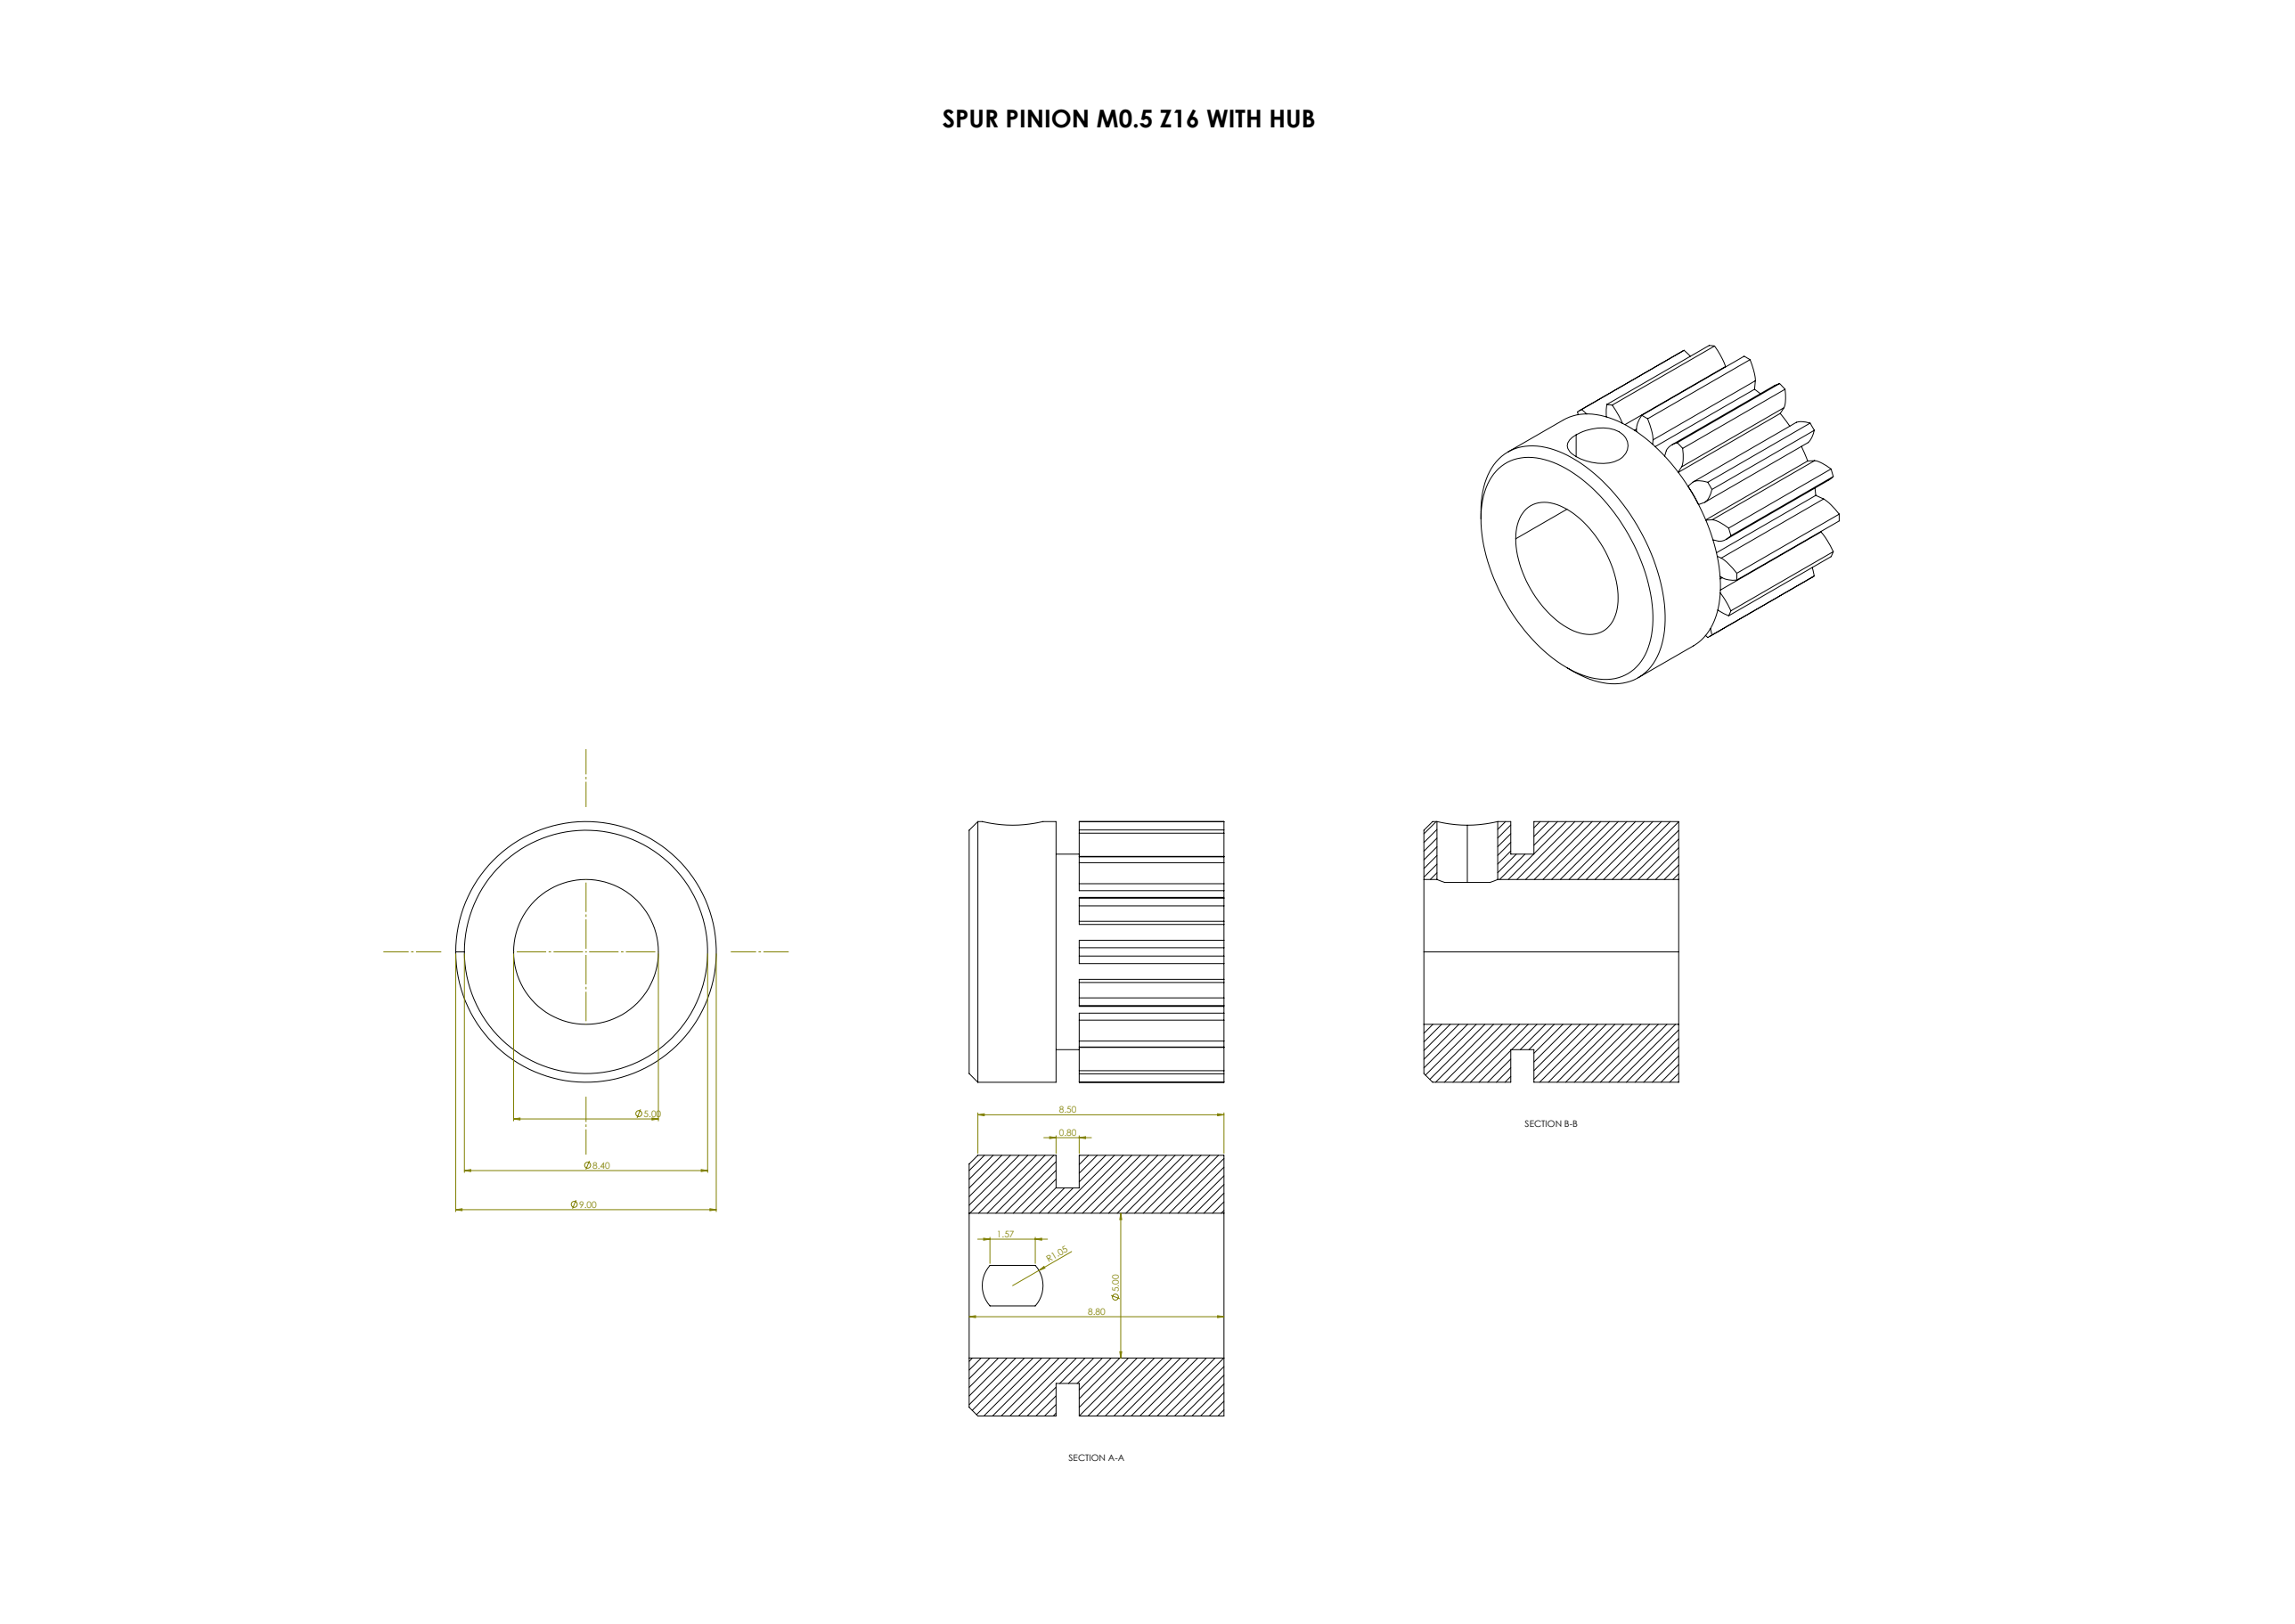
ISO-10303-21;
HEADER;
/* Generated by software containing ST-Developer
 * from STEP Tools, Inc. (www.steptools.com) 
 */

FILE_DESCRIPTION(
/* description */ (''),
/* implementation_level */ '2;1');

FILE_NAME(
/* name */ 'Spur Pinion m0.5 z16 with Hub.step',
/* time_stamp */ '2026-10-05T09:57:53+05:00',
/* author */ (''),
/* organization */ (''),
/* preprocessor_version */ 'ST-DEVELOPER v20.2',
/* originating_system */ 'Autodesk Translation Framework v15.15.0.0',
/* authorisation */ '');

FILE_SCHEMA (('AUTOMOTIVE_DESIGN { 1 0 10303 214 3 1 1 }'));
ENDSEC;

DATA;
#10=MECHANICAL_DESIGN_GEOMETRIC_PRESENTATION_REPRESENTATION('',(#555),#113984);
#110=(
BOUNDED_SURFACE()
B_SPLINE_SURFACE(5,1,((#92751,#92752),(#92753,#92754),(#92755,#92756),(#92757,
#92758),(#92759,#92760),(#92761,#92762),(#92763,#92764),(#92765,#92766),
(#92767,#92768),(#92769,#92770),(#92771,#92772),(#92773,#92774),(#92775,
#92776),(#92777,#92778),(#92779,#92780),(#92781,#92782),(#92783,#92784),
(#92785,#92786),(#92787,#92788),(#92789,#92790),(#92791,#92792),(#92793,
#92794),(#92795,#92796),(#92797,#92798),(#92799,#92800),(#92801,#92802),
(#92803,#92804),(#92805,#92806),(#92807,#92808),(#92809,#92810),(#92811,
#92812),(#92813,#92814),(#92815,#92816),(#92817,#92818),(#92819,#92820)),
 .UNSPECIFIED.,.F.,.F.,.F.)
B_SPLINE_SURFACE_WITH_KNOTS((6,1,1,1,1,1,1,1,1,1,1,1,1,1,1,1,1,1,1,1,1,
1,1,1,1,1,1,1,1,1,6),(2,2),(-1.,-0.966666666666667,-0.933333333333333,-0.9,
-0.866666666666667,-0.833333333333333,-0.8,-0.766666666666667,-0.733333333333333,
-0.7,-0.666666666666667,-0.633333333333333,-0.6,-0.566666666666667,-0.533333333333333,
-0.5,-0.466666666666667,-0.433333333333333,-0.4,-0.366666666666667,-0.333333333333333,
-0.3,-0.266666666666667,-0.233333333333333,-0.2,-0.166666666666667,-0.133333333333333,
-0.1,-0.0666666666666667,-0.0333333333333333,0.),(0.,0.5),.UNSPECIFIED.)
GEOMETRIC_REPRESENTATION_ITEM()
RATIONAL_B_SPLINE_SURFACE(((1.,1.),(1.,1.),(1.,1.),(1.,1.),(1.,1.),(1.,
1.),(1.,1.),(1.,1.),(1.,1.),(1.,1.),(1.,1.),(1.,1.),(1.,1.),(1.,1.),(1.,
1.),(1.,1.),(1.,1.),(1.,1.),(1.,1.),(1.,1.),(1.,1.),(1.,1.),(1.,1.),(1.,
1.),(1.,1.),(1.,1.),(1.,1.),(1.,1.),(1.,1.),(1.,1.),(1.,1.),(1.,1.),(1.,
1.),(1.,1.),(1.,1.)))
REPRESENTATION_ITEM('')
SURFACE()
);
#111=(
BOUNDED_SURFACE()
B_SPLINE_SURFACE(5,1,((#92900,#92901),(#92902,#92903),(#92904,#92905),(#92906,
#92907),(#92908,#92909),(#92910,#92911),(#92912,#92913),(#92914,#92915),
(#92916,#92917),(#92918,#92919),(#92920,#92921),(#92922,#92923),(#92924,
#92925),(#92926,#92927),(#92928,#92929),(#92930,#92931),(#92932,#92933),
(#92934,#92935),(#92936,#92937),(#92938,#92939),(#92940,#92941),(#92942,
#92943),(#92944,#92945),(#92946,#92947),(#92948,#92949),(#92950,#92951),
(#92952,#92953),(#92954,#92955),(#92956,#92957),(#92958,#92959),(#92960,
#92961),(#92962,#92963),(#92964,#92965),(#92966,#92967),(#92968,#92969)),
 .UNSPECIFIED.,.F.,.F.,.F.)
B_SPLINE_SURFACE_WITH_KNOTS((6,1,1,1,1,1,1,1,1,1,1,1,1,1,1,1,1,1,1,1,1,
1,1,1,1,1,1,1,1,1,6),(2,2),(0.,0.0333333333333333,0.0666666666666667,0.1,
0.133333333333333,0.166666666666667,0.2,0.233333333333333,0.266666666666667,
0.3,0.333333333333333,0.366666666666667,0.4,0.433333333333333,0.466666666666667,
0.5,0.533333333333333,0.566666666666667,0.6,0.633333333333333,0.666666666666667,
0.7,0.733333333333333,0.766666666666667,0.8,0.833333333333333,0.866666666666667,
0.9,0.933333333333333,0.966666666666667,1.),(0.,0.5),.UNSPECIFIED.)
GEOMETRIC_REPRESENTATION_ITEM()
RATIONAL_B_SPLINE_SURFACE(((1.,1.),(1.,1.),(1.,1.),(1.,1.),(1.,1.),(1.,
1.),(1.,1.),(1.,1.),(1.,1.),(1.,1.),(1.,1.),(1.,1.),(1.,1.),(1.,1.),(1.,
1.),(1.,1.),(1.,1.),(1.,1.),(1.,1.),(1.,1.),(1.,1.),(1.,1.),(1.,1.),(1.,
1.),(1.,1.),(1.,1.),(1.,1.),(1.,1.),(1.,1.),(1.,1.),(1.,1.),(1.,1.),(1.,
1.),(1.,1.),(1.,1.)))
REPRESENTATION_ITEM('')
SURFACE()
);
#112=(
BOUNDED_SURFACE()
B_SPLINE_SURFACE(5,1,((#93181,#93182),(#93183,#93184),(#93185,#93186),(#93187,
#93188),(#93189,#93190),(#93191,#93192),(#93193,#93194),(#93195,#93196),
(#93197,#93198),(#93199,#93200),(#93201,#93202),(#93203,#93204),(#93205,
#93206),(#93207,#93208),(#93209,#93210),(#93211,#93212),(#93213,#93214),
(#93215,#93216),(#93217,#93218),(#93219,#93220),(#93221,#93222),(#93223,
#93224),(#93225,#93226),(#93227,#93228),(#93229,#93230),(#93231,#93232),
(#93233,#93234),(#93235,#93236),(#93237,#93238),(#93239,#93240),(#93241,
#93242),(#93243,#93244),(#93245,#93246),(#93247,#93248),(#93249,#93250)),
 .UNSPECIFIED.,.F.,.F.,.F.)
B_SPLINE_SURFACE_WITH_KNOTS((6,1,1,1,1,1,1,1,1,1,1,1,1,1,1,1,1,1,1,1,1,
1,1,1,1,1,1,1,1,1,6),(2,2),(-1.,-0.966666666666667,-0.933333333333333,-0.9,
-0.866666666666667,-0.833333333333333,-0.8,-0.766666666666667,-0.733333333333333,
-0.7,-0.666666666666667,-0.633333333333333,-0.6,-0.566666666666667,-0.533333333333333,
-0.5,-0.466666666666667,-0.433333333333333,-0.4,-0.366666666666667,-0.333333333333333,
-0.3,-0.266666666666667,-0.233333333333333,-0.2,-0.166666666666667,-0.133333333333333,
-0.1,-0.0666666666666667,-0.0333333333333333,0.),(0.,0.5),.UNSPECIFIED.)
GEOMETRIC_REPRESENTATION_ITEM()
RATIONAL_B_SPLINE_SURFACE(((1.,1.),(1.,1.),(1.,1.),(1.,1.),(1.,1.),(1.,
1.),(1.,1.),(1.,1.),(1.,1.),(1.,1.),(1.,1.),(1.,1.),(1.,1.),(1.,1.),(1.,
1.),(1.,1.),(1.,1.),(1.,1.),(1.,1.),(1.,1.),(1.,1.),(1.,1.),(1.,1.),(1.,
1.),(1.,1.),(1.,1.),(1.,1.),(1.,1.),(1.,1.),(1.,1.),(1.,1.),(1.,1.),(1.,
1.),(1.,1.),(1.,1.)))
REPRESENTATION_ITEM('')
SURFACE()
);
#113=(
BOUNDED_SURFACE()
B_SPLINE_SURFACE(5,1,((#93330,#93331),(#93332,#93333),(#93334,#93335),(#93336,
#93337),(#93338,#93339),(#93340,#93341),(#93342,#93343),(#93344,#93345),
(#93346,#93347),(#93348,#93349),(#93350,#93351),(#93352,#93353),(#93354,
#93355),(#93356,#93357),(#93358,#93359),(#93360,#93361),(#93362,#93363),
(#93364,#93365),(#93366,#93367),(#93368,#93369),(#93370,#93371),(#93372,
#93373),(#93374,#93375),(#93376,#93377),(#93378,#93379),(#93380,#93381),
(#93382,#93383),(#93384,#93385),(#93386,#93387),(#93388,#93389),(#93390,
#93391),(#93392,#93393),(#93394,#93395),(#93396,#93397),(#93398,#93399)),
 .UNSPECIFIED.,.F.,.F.,.F.)
B_SPLINE_SURFACE_WITH_KNOTS((6,1,1,1,1,1,1,1,1,1,1,1,1,1,1,1,1,1,1,1,1,
1,1,1,1,1,1,1,1,1,6),(2,2),(0.,0.0333333333333333,0.0666666666666667,0.1,
0.133333333333333,0.166666666666667,0.2,0.233333333333333,0.266666666666667,
0.3,0.333333333333333,0.366666666666667,0.4,0.433333333333333,0.466666666666667,
0.5,0.533333333333333,0.566666666666667,0.6,0.633333333333333,0.666666666666667,
0.7,0.733333333333333,0.766666666666667,0.8,0.833333333333333,0.866666666666667,
0.9,0.933333333333333,0.966666666666667,1.),(0.,0.5),.UNSPECIFIED.)
GEOMETRIC_REPRESENTATION_ITEM()
RATIONAL_B_SPLINE_SURFACE(((1.,1.),(1.,1.),(1.,1.),(1.,1.),(1.,1.),(1.,
1.),(1.,1.),(1.,1.),(1.,1.),(1.,1.),(1.,1.),(1.,1.),(1.,1.),(1.,1.),(1.,
1.),(1.,1.),(1.,1.),(1.,1.),(1.,1.),(1.,1.),(1.,1.),(1.,1.),(1.,1.),(1.,
1.),(1.,1.),(1.,1.),(1.,1.),(1.,1.),(1.,1.),(1.,1.),(1.,1.),(1.,1.),(1.,
1.),(1.,1.),(1.,1.)))
REPRESENTATION_ITEM('')
SURFACE()
);
#114=(
BOUNDED_SURFACE()
B_SPLINE_SURFACE(5,1,((#93483,#93484),(#93485,#93486),(#93487,#93488),(#93489,
#93490),(#93491,#93492),(#93493,#93494),(#93495,#93496),(#93497,#93498),
(#93499,#93500),(#93501,#93502),(#93503,#93504),(#93505,#93506),(#93507,
#93508),(#93509,#93510),(#93511,#93512),(#93513,#93514),(#93515,#93516),
(#93517,#93518),(#93519,#93520),(#93521,#93522),(#93523,#93524),(#93525,
#93526),(#93527,#93528),(#93529,#93530),(#93531,#93532),(#93533,#93534),
(#93535,#93536),(#93537,#93538),(#93539,#93540),(#93541,#93542),(#93543,
#93544),(#93545,#93546),(#93547,#93548),(#93549,#93550),(#93551,#93552)),
 .UNSPECIFIED.,.F.,.F.,.F.)
B_SPLINE_SURFACE_WITH_KNOTS((6,1,1,1,1,1,1,1,1,1,1,1,1,1,1,1,1,1,1,1,1,
1,1,1,1,1,1,1,1,1,6),(2,2),(-1.,-0.966666666666667,-0.933333333333333,-0.9,
-0.866666666666667,-0.833333333333333,-0.8,-0.766666666666667,-0.733333333333333,
-0.7,-0.666666666666667,-0.633333333333333,-0.6,-0.566666666666667,-0.533333333333333,
-0.5,-0.466666666666667,-0.433333333333333,-0.4,-0.366666666666667,-0.333333333333333,
-0.3,-0.266666666666667,-0.233333333333333,-0.2,-0.166666666666667,-0.133333333333333,
-0.1,-0.0666666666666667,-0.0333333333333333,0.),(0.,0.5),.UNSPECIFIED.)
GEOMETRIC_REPRESENTATION_ITEM()
RATIONAL_B_SPLINE_SURFACE(((1.,1.),(1.,1.),(1.,1.),(1.,1.),(1.,1.),(1.,
1.),(1.,1.),(1.,1.),(1.,1.),(1.,1.),(1.,1.),(1.,1.),(1.,1.),(1.,1.),(1.,
1.),(1.,1.),(1.,1.),(1.,1.),(1.,1.),(1.,1.),(1.,1.),(1.,1.),(1.,1.),(1.,
1.),(1.,1.),(1.,1.),(1.,1.),(1.,1.),(1.,1.),(1.,1.),(1.,1.),(1.,1.),(1.,
1.),(1.,1.),(1.,1.)))
REPRESENTATION_ITEM('')
SURFACE()
);
#115=(
BOUNDED_SURFACE()
B_SPLINE_SURFACE(5,1,((#93632,#93633),(#93634,#93635),(#93636,#93637),(#93638,
#93639),(#93640,#93641),(#93642,#93643),(#93644,#93645),(#93646,#93647),
(#93648,#93649),(#93650,#93651),(#93652,#93653),(#93654,#93655),(#93656,
#93657),(#93658,#93659),(#93660,#93661),(#93662,#93663),(#93664,#93665),
(#93666,#93667),(#93668,#93669),(#93670,#93671),(#93672,#93673),(#93674,
#93675),(#93676,#93677),(#93678,#93679),(#93680,#93681),(#93682,#93683),
(#93684,#93685),(#93686,#93687),(#93688,#93689),(#93690,#93691),(#93692,
#93693),(#93694,#93695),(#93696,#93697),(#93698,#93699),(#93700,#93701)),
 .UNSPECIFIED.,.F.,.F.,.F.)
B_SPLINE_SURFACE_WITH_KNOTS((6,1,1,1,1,1,1,1,1,1,1,1,1,1,1,1,1,1,1,1,1,
1,1,1,1,1,1,1,1,1,6),(2,2),(0.,0.0333333333333333,0.0666666666666667,0.1,
0.133333333333333,0.166666666666667,0.2,0.233333333333333,0.266666666666667,
0.3,0.333333333333333,0.366666666666667,0.4,0.433333333333333,0.466666666666667,
0.5,0.533333333333333,0.566666666666667,0.6,0.633333333333333,0.666666666666667,
0.7,0.733333333333333,0.766666666666667,0.8,0.833333333333333,0.866666666666667,
0.9,0.933333333333333,0.966666666666667,1.),(0.,0.5),.UNSPECIFIED.)
GEOMETRIC_REPRESENTATION_ITEM()
RATIONAL_B_SPLINE_SURFACE(((1.,1.),(1.,1.),(1.,1.),(1.,1.),(1.,1.),(1.,
1.),(1.,1.),(1.,1.),(1.,1.),(1.,1.),(1.,1.),(1.,1.),(1.,1.),(1.,1.),(1.,
1.),(1.,1.),(1.,1.),(1.,1.),(1.,1.),(1.,1.),(1.,1.),(1.,1.),(1.,1.),(1.,
1.),(1.,1.),(1.,1.),(1.,1.),(1.,1.),(1.,1.),(1.,1.),(1.,1.),(1.,1.),(1.,
1.),(1.,1.),(1.,1.)))
REPRESENTATION_ITEM('')
SURFACE()
);
#116=(
BOUNDED_SURFACE()
B_SPLINE_SURFACE(5,1,((#93785,#93786),(#93787,#93788),(#93789,#93790),(#93791,
#93792),(#93793,#93794),(#93795,#93796),(#93797,#93798),(#93799,#93800),
(#93801,#93802),(#93803,#93804),(#93805,#93806),(#93807,#93808),(#93809,
#93810),(#93811,#93812),(#93813,#93814),(#93815,#93816),(#93817,#93818),
(#93819,#93820),(#93821,#93822),(#93823,#93824),(#93825,#93826),(#93827,
#93828),(#93829,#93830),(#93831,#93832),(#93833,#93834),(#93835,#93836),
(#93837,#93838),(#93839,#93840),(#93841,#93842),(#93843,#93844),(#93845,
#93846),(#93847,#93848),(#93849,#93850),(#93851,#93852),(#93853,#93854)),
 .UNSPECIFIED.,.F.,.F.,.F.)
B_SPLINE_SURFACE_WITH_KNOTS((6,1,1,1,1,1,1,1,1,1,1,1,1,1,1,1,1,1,1,1,1,
1,1,1,1,1,1,1,1,1,6),(2,2),(-1.,-0.966666666666667,-0.933333333333333,-0.9,
-0.866666666666667,-0.833333333333333,-0.8,-0.766666666666667,-0.733333333333333,
-0.7,-0.666666666666667,-0.633333333333333,-0.6,-0.566666666666667,-0.533333333333333,
-0.5,-0.466666666666667,-0.433333333333333,-0.4,-0.366666666666667,-0.333333333333333,
-0.3,-0.266666666666667,-0.233333333333333,-0.2,-0.166666666666667,-0.133333333333333,
-0.1,-0.0666666666666667,-0.0333333333333333,0.),(0.,0.5),.UNSPECIFIED.)
GEOMETRIC_REPRESENTATION_ITEM()
RATIONAL_B_SPLINE_SURFACE(((1.,1.),(1.,1.),(1.,1.),(1.,1.),(1.,1.),(1.,
1.),(1.,1.),(1.,1.),(1.,1.),(1.,1.),(1.,1.),(1.,1.),(1.,1.),(1.,1.),(1.,
1.),(1.,1.),(1.,1.),(1.,1.),(1.,1.),(1.,1.),(1.,1.),(1.,1.),(1.,1.),(1.,
1.),(1.,1.),(1.,1.),(1.,1.),(1.,1.),(1.,1.),(1.,1.),(1.,1.),(1.,1.),(1.,
1.),(1.,1.),(1.,1.)))
REPRESENTATION_ITEM('')
SURFACE()
);
#117=(
BOUNDED_SURFACE()
B_SPLINE_SURFACE(5,1,((#93934,#93935),(#93936,#93937),(#93938,#93939),(#93940,
#93941),(#93942,#93943),(#93944,#93945),(#93946,#93947),(#93948,#93949),
(#93950,#93951),(#93952,#93953),(#93954,#93955),(#93956,#93957),(#93958,
#93959),(#93960,#93961),(#93962,#93963),(#93964,#93965),(#93966,#93967),
(#93968,#93969),(#93970,#93971),(#93972,#93973),(#93974,#93975),(#93976,
#93977),(#93978,#93979),(#93980,#93981),(#93982,#93983),(#93984,#93985),
(#93986,#93987),(#93988,#93989),(#93990,#93991),(#93992,#93993),(#93994,
#93995),(#93996,#93997),(#93998,#93999),(#94000,#94001),(#94002,#94003)),
 .UNSPECIFIED.,.F.,.F.,.F.)
B_SPLINE_SURFACE_WITH_KNOTS((6,1,1,1,1,1,1,1,1,1,1,1,1,1,1,1,1,1,1,1,1,
1,1,1,1,1,1,1,1,1,6),(2,2),(0.,0.0333333333333333,0.0666666666666667,0.1,
0.133333333333333,0.166666666666667,0.2,0.233333333333333,0.266666666666667,
0.3,0.333333333333333,0.366666666666667,0.4,0.433333333333333,0.466666666666667,
0.5,0.533333333333333,0.566666666666667,0.6,0.633333333333333,0.666666666666667,
0.7,0.733333333333333,0.766666666666667,0.8,0.833333333333333,0.866666666666667,
0.9,0.933333333333333,0.966666666666667,1.),(0.,0.5),.UNSPECIFIED.)
GEOMETRIC_REPRESENTATION_ITEM()
RATIONAL_B_SPLINE_SURFACE(((1.,1.),(1.,1.),(1.,1.),(1.,1.),(1.,1.),(1.,
1.),(1.,1.),(1.,1.),(1.,1.),(1.,1.),(1.,1.),(1.,1.),(1.,1.),(1.,1.),(1.,
1.),(1.,1.),(1.,1.),(1.,1.),(1.,1.),(1.,1.),(1.,1.),(1.,1.),(1.,1.),(1.,
1.),(1.,1.),(1.,1.),(1.,1.),(1.,1.),(1.,1.),(1.,1.),(1.,1.),(1.,1.),(1.,
1.),(1.,1.),(1.,1.)))
REPRESENTATION_ITEM('')
SURFACE()
);
#118=(
BOUNDED_SURFACE()
B_SPLINE_SURFACE(5,1,((#94087,#94088),(#94089,#94090),(#94091,#94092),(#94093,
#94094),(#94095,#94096),(#94097,#94098),(#94099,#94100),(#94101,#94102),
(#94103,#94104),(#94105,#94106),(#94107,#94108),(#94109,#94110),(#94111,
#94112),(#94113,#94114),(#94115,#94116),(#94117,#94118),(#94119,#94120),
(#94121,#94122),(#94123,#94124),(#94125,#94126),(#94127,#94128),(#94129,
#94130),(#94131,#94132),(#94133,#94134),(#94135,#94136),(#94137,#94138),
(#94139,#94140),(#94141,#94142),(#94143,#94144),(#94145,#94146),(#94147,
#94148),(#94149,#94150),(#94151,#94152),(#94153,#94154),(#94155,#94156)),
 .UNSPECIFIED.,.F.,.F.,.F.)
B_SPLINE_SURFACE_WITH_KNOTS((6,1,1,1,1,1,1,1,1,1,1,1,1,1,1,1,1,1,1,1,1,
1,1,1,1,1,1,1,1,1,6),(2,2),(-1.,-0.966666666666667,-0.933333333333333,-0.9,
-0.866666666666667,-0.833333333333333,-0.8,-0.766666666666667,-0.733333333333333,
-0.7,-0.666666666666667,-0.633333333333333,-0.6,-0.566666666666667,-0.533333333333333,
-0.5,-0.466666666666667,-0.433333333333333,-0.4,-0.366666666666667,-0.333333333333333,
-0.3,-0.266666666666667,-0.233333333333333,-0.2,-0.166666666666667,-0.133333333333333,
-0.1,-0.0666666666666667,-0.0333333333333333,0.),(0.,0.5),.UNSPECIFIED.)
GEOMETRIC_REPRESENTATION_ITEM()
RATIONAL_B_SPLINE_SURFACE(((1.,1.),(1.,1.),(1.,1.),(1.,1.),(1.,1.),(1.,
1.),(1.,1.),(1.,1.),(1.,1.),(1.,1.),(1.,1.),(1.,1.),(1.,1.),(1.,1.),(1.,
1.),(1.,1.),(1.,1.),(1.,1.),(1.,1.),(1.,1.),(1.,1.),(1.,1.),(1.,1.),(1.,
1.),(1.,1.),(1.,1.),(1.,1.),(1.,1.),(1.,1.),(1.,1.),(1.,1.),(1.,1.),(1.,
1.),(1.,1.),(1.,1.)))
REPRESENTATION_ITEM('')
SURFACE()
);
#119=(
BOUNDED_SURFACE()
B_SPLINE_SURFACE(5,1,((#94236,#94237),(#94238,#94239),(#94240,#94241),(#94242,
#94243),(#94244,#94245),(#94246,#94247),(#94248,#94249),(#94250,#94251),
(#94252,#94253),(#94254,#94255),(#94256,#94257),(#94258,#94259),(#94260,
#94261),(#94262,#94263),(#94264,#94265),(#94266,#94267),(#94268,#94269),
(#94270,#94271),(#94272,#94273),(#94274,#94275),(#94276,#94277),(#94278,
#94279),(#94280,#94281),(#94282,#94283),(#94284,#94285),(#94286,#94287),
(#94288,#94289),(#94290,#94291),(#94292,#94293),(#94294,#94295),(#94296,
#94297),(#94298,#94299),(#94300,#94301),(#94302,#94303),(#94304,#94305)),
 .UNSPECIFIED.,.F.,.F.,.F.)
B_SPLINE_SURFACE_WITH_KNOTS((6,1,1,1,1,1,1,1,1,1,1,1,1,1,1,1,1,1,1,1,1,
1,1,1,1,1,1,1,1,1,6),(2,2),(0.,0.0333333333333333,0.0666666666666667,0.1,
0.133333333333333,0.166666666666667,0.2,0.233333333333333,0.266666666666667,
0.3,0.333333333333333,0.366666666666667,0.4,0.433333333333333,0.466666666666667,
0.5,0.533333333333333,0.566666666666667,0.6,0.633333333333333,0.666666666666667,
0.7,0.733333333333333,0.766666666666667,0.8,0.833333333333333,0.866666666666667,
0.9,0.933333333333333,0.966666666666667,1.),(0.,0.5),.UNSPECIFIED.)
GEOMETRIC_REPRESENTATION_ITEM()
RATIONAL_B_SPLINE_SURFACE(((1.,1.),(1.,1.),(1.,1.),(1.,1.),(1.,1.),(1.,
1.),(1.,1.),(1.,1.),(1.,1.),(1.,1.),(1.,1.),(1.,1.),(1.,1.),(1.,1.),(1.,
1.),(1.,1.),(1.,1.),(1.,1.),(1.,1.),(1.,1.),(1.,1.),(1.,1.),(1.,1.),(1.,
1.),(1.,1.),(1.,1.),(1.,1.),(1.,1.),(1.,1.),(1.,1.),(1.,1.),(1.,1.),(1.,
1.),(1.,1.),(1.,1.)))
REPRESENTATION_ITEM('')
SURFACE()
);
#120=(
BOUNDED_SURFACE()
B_SPLINE_SURFACE(5,1,((#94389,#94390),(#94391,#94392),(#94393,#94394),(#94395,
#94396),(#94397,#94398),(#94399,#94400),(#94401,#94402),(#94403,#94404),
(#94405,#94406),(#94407,#94408),(#94409,#94410),(#94411,#94412),(#94413,
#94414),(#94415,#94416),(#94417,#94418),(#94419,#94420),(#94421,#94422),
(#94423,#94424),(#94425,#94426),(#94427,#94428),(#94429,#94430),(#94431,
#94432),(#94433,#94434),(#94435,#94436),(#94437,#94438),(#94439,#94440),
(#94441,#94442),(#94443,#94444),(#94445,#94446),(#94447,#94448),(#94449,
#94450),(#94451,#94452),(#94453,#94454),(#94455,#94456),(#94457,#94458)),
 .UNSPECIFIED.,.F.,.F.,.F.)
B_SPLINE_SURFACE_WITH_KNOTS((6,1,1,1,1,1,1,1,1,1,1,1,1,1,1,1,1,1,1,1,1,
1,1,1,1,1,1,1,1,1,6),(2,2),(-1.,-0.966666666666667,-0.933333333333333,-0.9,
-0.866666666666667,-0.833333333333333,-0.8,-0.766666666666667,-0.733333333333333,
-0.7,-0.666666666666667,-0.633333333333333,-0.6,-0.566666666666667,-0.533333333333333,
-0.5,-0.466666666666667,-0.433333333333333,-0.4,-0.366666666666667,-0.333333333333333,
-0.3,-0.266666666666667,-0.233333333333333,-0.2,-0.166666666666667,-0.133333333333333,
-0.1,-0.0666666666666667,-0.0333333333333333,0.),(0.,0.5),.UNSPECIFIED.)
GEOMETRIC_REPRESENTATION_ITEM()
RATIONAL_B_SPLINE_SURFACE(((1.,1.),(1.,1.),(1.,1.),(1.,1.),(1.,1.),(1.,
1.),(1.,1.),(1.,1.),(1.,1.),(1.,1.),(1.,1.),(1.,1.),(1.,1.),(1.,1.),(1.,
1.),(1.,1.),(1.,1.),(1.,1.),(1.,1.),(1.,1.),(1.,1.),(1.,1.),(1.,1.),(1.,
1.),(1.,1.),(1.,1.),(1.,1.),(1.,1.),(1.,1.),(1.,1.),(1.,1.),(1.,1.),(1.,
1.),(1.,1.),(1.,1.)))
REPRESENTATION_ITEM('')
SURFACE()
);
#121=(
BOUNDED_SURFACE()
B_SPLINE_SURFACE(5,1,((#94538,#94539),(#94540,#94541),(#94542,#94543),(#94544,
#94545),(#94546,#94547),(#94548,#94549),(#94550,#94551),(#94552,#94553),
(#94554,#94555),(#94556,#94557),(#94558,#94559),(#94560,#94561),(#94562,
#94563),(#94564,#94565),(#94566,#94567),(#94568,#94569),(#94570,#94571),
(#94572,#94573),(#94574,#94575),(#94576,#94577),(#94578,#94579),(#94580,
#94581),(#94582,#94583),(#94584,#94585),(#94586,#94587),(#94588,#94589),
(#94590,#94591),(#94592,#94593),(#94594,#94595),(#94596,#94597),(#94598,
#94599),(#94600,#94601),(#94602,#94603),(#94604,#94605),(#94606,#94607)),
 .UNSPECIFIED.,.F.,.F.,.F.)
B_SPLINE_SURFACE_WITH_KNOTS((6,1,1,1,1,1,1,1,1,1,1,1,1,1,1,1,1,1,1,1,1,
1,1,1,1,1,1,1,1,1,6),(2,2),(0.,0.0333333333333333,0.0666666666666667,0.1,
0.133333333333333,0.166666666666667,0.2,0.233333333333333,0.266666666666667,
0.3,0.333333333333333,0.366666666666667,0.4,0.433333333333333,0.466666666666667,
0.5,0.533333333333333,0.566666666666667,0.6,0.633333333333333,0.666666666666667,
0.7,0.733333333333333,0.766666666666667,0.8,0.833333333333333,0.866666666666667,
0.9,0.933333333333333,0.966666666666667,1.),(0.,0.5),.UNSPECIFIED.)
GEOMETRIC_REPRESENTATION_ITEM()
RATIONAL_B_SPLINE_SURFACE(((1.,1.),(1.,1.),(1.,1.),(1.,1.),(1.,1.),(1.,
1.),(1.,1.),(1.,1.),(1.,1.),(1.,1.),(1.,1.),(1.,1.),(1.,1.),(1.,1.),(1.,
1.),(1.,1.),(1.,1.),(1.,1.),(1.,1.),(1.,1.),(1.,1.),(1.,1.),(1.,1.),(1.,
1.),(1.,1.),(1.,1.),(1.,1.),(1.,1.),(1.,1.),(1.,1.),(1.,1.),(1.,1.),(1.,
1.),(1.,1.),(1.,1.)))
REPRESENTATION_ITEM('')
SURFACE()
);
#122=(
BOUNDED_SURFACE()
B_SPLINE_SURFACE(5,1,((#94691,#94692),(#94693,#94694),(#94695,#94696),(#94697,
#94698),(#94699,#94700),(#94701,#94702),(#94703,#94704),(#94705,#94706),
(#94707,#94708),(#94709,#94710),(#94711,#94712),(#94713,#94714),(#94715,
#94716),(#94717,#94718),(#94719,#94720),(#94721,#94722),(#94723,#94724),
(#94725,#94726),(#94727,#94728),(#94729,#94730),(#94731,#94732),(#94733,
#94734),(#94735,#94736),(#94737,#94738),(#94739,#94740),(#94741,#94742),
(#94743,#94744),(#94745,#94746),(#94747,#94748),(#94749,#94750),(#94751,
#94752),(#94753,#94754),(#94755,#94756),(#94757,#94758),(#94759,#94760)),
 .UNSPECIFIED.,.F.,.F.,.F.)
B_SPLINE_SURFACE_WITH_KNOTS((6,1,1,1,1,1,1,1,1,1,1,1,1,1,1,1,1,1,1,1,1,
1,1,1,1,1,1,1,1,1,6),(2,2),(-1.,-0.966666666666667,-0.933333333333333,-0.9,
-0.866666666666667,-0.833333333333333,-0.8,-0.766666666666667,-0.733333333333333,
-0.7,-0.666666666666667,-0.633333333333333,-0.6,-0.566666666666667,-0.533333333333333,
-0.5,-0.466666666666667,-0.433333333333333,-0.4,-0.366666666666667,-0.333333333333333,
-0.3,-0.266666666666667,-0.233333333333333,-0.2,-0.166666666666667,-0.133333333333333,
-0.1,-0.0666666666666667,-0.0333333333333333,0.),(0.,0.5),.UNSPECIFIED.)
GEOMETRIC_REPRESENTATION_ITEM()
RATIONAL_B_SPLINE_SURFACE(((1.,1.),(1.,1.),(1.,1.),(1.,1.),(1.,1.),(1.,
1.),(1.,1.),(1.,1.),(1.,1.),(1.,1.),(1.,1.),(1.,1.),(1.,1.),(1.,1.),(1.,
1.),(1.,1.),(1.,1.),(1.,1.),(1.,1.),(1.,1.),(1.,1.),(1.,1.),(1.,1.),(1.,
1.),(1.,1.),(1.,1.),(1.,1.),(1.,1.),(1.,1.),(1.,1.),(1.,1.),(1.,1.),(1.,
1.),(1.,1.),(1.,1.)))
REPRESENTATION_ITEM('')
SURFACE()
);
#123=(
BOUNDED_SURFACE()
B_SPLINE_SURFACE(5,1,((#94840,#94841),(#94842,#94843),(#94844,#94845),(#94846,
#94847),(#94848,#94849),(#94850,#94851),(#94852,#94853),(#94854,#94855),
(#94856,#94857),(#94858,#94859),(#94860,#94861),(#94862,#94863),(#94864,
#94865),(#94866,#94867),(#94868,#94869),(#94870,#94871),(#94872,#94873),
(#94874,#94875),(#94876,#94877),(#94878,#94879),(#94880,#94881),(#94882,
#94883),(#94884,#94885),(#94886,#94887),(#94888,#94889),(#94890,#94891),
(#94892,#94893),(#94894,#94895),(#94896,#94897),(#94898,#94899),(#94900,
#94901),(#94902,#94903),(#94904,#94905),(#94906,#94907),(#94908,#94909)),
 .UNSPECIFIED.,.F.,.F.,.F.)
B_SPLINE_SURFACE_WITH_KNOTS((6,1,1,1,1,1,1,1,1,1,1,1,1,1,1,1,1,1,1,1,1,
1,1,1,1,1,1,1,1,1,6),(2,2),(0.,0.0333333333333333,0.0666666666666667,0.1,
0.133333333333333,0.166666666666667,0.2,0.233333333333333,0.266666666666667,
0.3,0.333333333333333,0.366666666666667,0.4,0.433333333333333,0.466666666666667,
0.5,0.533333333333333,0.566666666666667,0.6,0.633333333333333,0.666666666666667,
0.7,0.733333333333333,0.766666666666667,0.8,0.833333333333333,0.866666666666667,
0.9,0.933333333333333,0.966666666666667,1.),(0.,0.5),.UNSPECIFIED.)
GEOMETRIC_REPRESENTATION_ITEM()
RATIONAL_B_SPLINE_SURFACE(((1.,1.),(1.,1.),(1.,1.),(1.,1.),(1.,1.),(1.,
1.),(1.,1.),(1.,1.),(1.,1.),(1.,1.),(1.,1.),(1.,1.),(1.,1.),(1.,1.),(1.,
1.),(1.,1.),(1.,1.),(1.,1.),(1.,1.),(1.,1.),(1.,1.),(1.,1.),(1.,1.),(1.,
1.),(1.,1.),(1.,1.),(1.,1.),(1.,1.),(1.,1.),(1.,1.),(1.,1.),(1.,1.),(1.,
1.),(1.,1.),(1.,1.)))
REPRESENTATION_ITEM('')
SURFACE()
);
#124=(
BOUNDED_SURFACE()
B_SPLINE_SURFACE(5,1,((#94993,#94994),(#94995,#94996),(#94997,#94998),(#94999,
#95000),(#95001,#95002),(#95003,#95004),(#95005,#95006),(#95007,#95008),
(#95009,#95010),(#95011,#95012),(#95013,#95014),(#95015,#95016),(#95017,
#95018),(#95019,#95020),(#95021,#95022),(#95023,#95024),(#95025,#95026),
(#95027,#95028),(#95029,#95030),(#95031,#95032),(#95033,#95034),(#95035,
#95036),(#95037,#95038),(#95039,#95040),(#95041,#95042),(#95043,#95044),
(#95045,#95046),(#95047,#95048),(#95049,#95050),(#95051,#95052),(#95053,
#95054),(#95055,#95056),(#95057,#95058),(#95059,#95060),(#95061,#95062)),
 .UNSPECIFIED.,.F.,.F.,.F.)
B_SPLINE_SURFACE_WITH_KNOTS((6,1,1,1,1,1,1,1,1,1,1,1,1,1,1,1,1,1,1,1,1,
1,1,1,1,1,1,1,1,1,6),(2,2),(-1.,-0.966666666666667,-0.933333333333333,-0.9,
-0.866666666666667,-0.833333333333333,-0.8,-0.766666666666667,-0.733333333333333,
-0.7,-0.666666666666667,-0.633333333333333,-0.6,-0.566666666666667,-0.533333333333333,
-0.5,-0.466666666666667,-0.433333333333333,-0.4,-0.366666666666667,-0.333333333333333,
-0.3,-0.266666666666667,-0.233333333333333,-0.2,-0.166666666666667,-0.133333333333333,
-0.1,-0.0666666666666667,-0.0333333333333333,0.),(0.,0.5),.UNSPECIFIED.)
GEOMETRIC_REPRESENTATION_ITEM()
RATIONAL_B_SPLINE_SURFACE(((1.,1.),(1.,1.),(1.,1.),(1.,1.),(1.,1.),(1.,
1.),(1.,1.),(1.,1.),(1.,1.),(1.,1.),(1.,1.),(1.,1.),(1.,1.),(1.,1.),(1.,
1.),(1.,1.),(1.,1.),(1.,1.),(1.,1.),(1.,1.),(1.,1.),(1.,1.),(1.,1.),(1.,
1.),(1.,1.),(1.,1.),(1.,1.),(1.,1.),(1.,1.),(1.,1.),(1.,1.),(1.,1.),(1.,
1.),(1.,1.),(1.,1.)))
REPRESENTATION_ITEM('')
SURFACE()
);
#125=(
BOUNDED_SURFACE()
B_SPLINE_SURFACE(5,1,((#95142,#95143),(#95144,#95145),(#95146,#95147),(#95148,
#95149),(#95150,#95151),(#95152,#95153),(#95154,#95155),(#95156,#95157),
(#95158,#95159),(#95160,#95161),(#95162,#95163),(#95164,#95165),(#95166,
#95167),(#95168,#95169),(#95170,#95171),(#95172,#95173),(#95174,#95175),
(#95176,#95177),(#95178,#95179),(#95180,#95181),(#95182,#95183),(#95184,
#95185),(#95186,#95187),(#95188,#95189),(#95190,#95191),(#95192,#95193),
(#95194,#95195),(#95196,#95197),(#95198,#95199),(#95200,#95201),(#95202,
#95203),(#95204,#95205),(#95206,#95207),(#95208,#95209),(#95210,#95211)),
 .UNSPECIFIED.,.F.,.F.,.F.)
B_SPLINE_SURFACE_WITH_KNOTS((6,1,1,1,1,1,1,1,1,1,1,1,1,1,1,1,1,1,1,1,1,
1,1,1,1,1,1,1,1,1,6),(2,2),(0.,0.0333333333333333,0.0666666666666667,0.1,
0.133333333333333,0.166666666666667,0.2,0.233333333333333,0.266666666666667,
0.3,0.333333333333333,0.366666666666667,0.4,0.433333333333333,0.466666666666667,
0.5,0.533333333333333,0.566666666666667,0.6,0.633333333333333,0.666666666666667,
0.7,0.733333333333333,0.766666666666667,0.8,0.833333333333333,0.866666666666667,
0.9,0.933333333333333,0.966666666666667,1.),(0.,0.5),.UNSPECIFIED.)
GEOMETRIC_REPRESENTATION_ITEM()
RATIONAL_B_SPLINE_SURFACE(((1.,1.),(1.,1.),(1.,1.),(1.,1.),(1.,1.),(1.,
1.),(1.,1.),(1.,1.),(1.,1.),(1.,1.),(1.,1.),(1.,1.),(1.,1.),(1.,1.),(1.,
1.),(1.,1.),(1.,1.),(1.,1.),(1.,1.),(1.,1.),(1.,1.),(1.,1.),(1.,1.),(1.,
1.),(1.,1.),(1.,1.),(1.,1.),(1.,1.),(1.,1.),(1.,1.),(1.,1.),(1.,1.),(1.,
1.),(1.,1.),(1.,1.)))
REPRESENTATION_ITEM('')
SURFACE()
);
#126=(
BOUNDED_SURFACE()
B_SPLINE_SURFACE(5,1,((#95295,#95296),(#95297,#95298),(#95299,#95300),(#95301,
#95302),(#95303,#95304),(#95305,#95306),(#95307,#95308),(#95309,#95310),
(#95311,#95312),(#95313,#95314),(#95315,#95316),(#95317,#95318),(#95319,
#95320),(#95321,#95322),(#95323,#95324),(#95325,#95326),(#95327,#95328),
(#95329,#95330),(#95331,#95332),(#95333,#95334),(#95335,#95336),(#95337,
#95338),(#95339,#95340),(#95341,#95342),(#95343,#95344),(#95345,#95346),
(#95347,#95348),(#95349,#95350),(#95351,#95352),(#95353,#95354),(#95355,
#95356),(#95357,#95358),(#95359,#95360),(#95361,#95362),(#95363,#95364)),
 .UNSPECIFIED.,.F.,.F.,.F.)
B_SPLINE_SURFACE_WITH_KNOTS((6,1,1,1,1,1,1,1,1,1,1,1,1,1,1,1,1,1,1,1,1,
1,1,1,1,1,1,1,1,1,6),(2,2),(-1.,-0.966666666666667,-0.933333333333333,-0.9,
-0.866666666666667,-0.833333333333333,-0.8,-0.766666666666667,-0.733333333333333,
-0.7,-0.666666666666667,-0.633333333333333,-0.6,-0.566666666666667,-0.533333333333333,
-0.5,-0.466666666666667,-0.433333333333333,-0.4,-0.366666666666667,-0.333333333333333,
-0.3,-0.266666666666667,-0.233333333333333,-0.2,-0.166666666666667,-0.133333333333333,
-0.1,-0.0666666666666667,-0.0333333333333333,0.),(0.,0.5),.UNSPECIFIED.)
GEOMETRIC_REPRESENTATION_ITEM()
RATIONAL_B_SPLINE_SURFACE(((1.,1.),(1.,1.),(1.,1.),(1.,1.),(1.,1.),(1.,
1.),(1.,1.),(1.,1.),(1.,1.),(1.,1.),(1.,1.),(1.,1.),(1.,1.),(1.,1.),(1.,
1.),(1.,1.),(1.,1.),(1.,1.),(1.,1.),(1.,1.),(1.,1.),(1.,1.),(1.,1.),(1.,
1.),(1.,1.),(1.,1.),(1.,1.),(1.,1.),(1.,1.),(1.,1.),(1.,1.),(1.,1.),(1.,
1.),(1.,1.),(1.,1.)))
REPRESENTATION_ITEM('')
SURFACE()
);
#127=(
BOUNDED_SURFACE()
B_SPLINE_SURFACE(5,1,((#95444,#95445),(#95446,#95447),(#95448,#95449),(#95450,
#95451),(#95452,#95453),(#95454,#95455),(#95456,#95457),(#95458,#95459),
(#95460,#95461),(#95462,#95463),(#95464,#95465),(#95466,#95467),(#95468,
#95469),(#95470,#95471),(#95472,#95473),(#95474,#95475),(#95476,#95477),
(#95478,#95479),(#95480,#95481),(#95482,#95483),(#95484,#95485),(#95486,
#95487),(#95488,#95489),(#95490,#95491),(#95492,#95493),(#95494,#95495),
(#95496,#95497),(#95498,#95499),(#95500,#95501),(#95502,#95503),(#95504,
#95505),(#95506,#95507),(#95508,#95509),(#95510,#95511),(#95512,#95513)),
 .UNSPECIFIED.,.F.,.F.,.F.)
B_SPLINE_SURFACE_WITH_KNOTS((6,1,1,1,1,1,1,1,1,1,1,1,1,1,1,1,1,1,1,1,1,
1,1,1,1,1,1,1,1,1,6),(2,2),(0.,0.0333333333333333,0.0666666666666667,0.1,
0.133333333333333,0.166666666666667,0.2,0.233333333333333,0.266666666666667,
0.3,0.333333333333333,0.366666666666667,0.4,0.433333333333333,0.466666666666667,
0.5,0.533333333333333,0.566666666666667,0.6,0.633333333333333,0.666666666666667,
0.7,0.733333333333333,0.766666666666667,0.8,0.833333333333333,0.866666666666667,
0.9,0.933333333333333,0.966666666666667,1.),(0.,0.5),.UNSPECIFIED.)
GEOMETRIC_REPRESENTATION_ITEM()
RATIONAL_B_SPLINE_SURFACE(((1.,1.),(1.,1.),(1.,1.),(1.,1.),(1.,1.),(1.,
1.),(1.,1.),(1.,1.),(1.,1.),(1.,1.),(1.,1.),(1.,1.),(1.,1.),(1.,1.),(1.,
1.),(1.,1.),(1.,1.),(1.,1.),(1.,1.),(1.,1.),(1.,1.),(1.,1.),(1.,1.),(1.,
1.),(1.,1.),(1.,1.),(1.,1.),(1.,1.),(1.,1.),(1.,1.),(1.,1.),(1.,1.),(1.,
1.),(1.,1.),(1.,1.)))
REPRESENTATION_ITEM('')
SURFACE()
);
#128=(
BOUNDED_SURFACE()
B_SPLINE_SURFACE(5,1,((#95597,#95598),(#95599,#95600),(#95601,#95602),(#95603,
#95604),(#95605,#95606),(#95607,#95608),(#95609,#95610),(#95611,#95612),
(#95613,#95614),(#95615,#95616),(#95617,#95618),(#95619,#95620),(#95621,
#95622),(#95623,#95624),(#95625,#95626),(#95627,#95628),(#95629,#95630),
(#95631,#95632),(#95633,#95634),(#95635,#95636),(#95637,#95638),(#95639,
#95640),(#95641,#95642),(#95643,#95644),(#95645,#95646),(#95647,#95648),
(#95649,#95650),(#95651,#95652),(#95653,#95654),(#95655,#95656),(#95657,
#95658),(#95659,#95660),(#95661,#95662),(#95663,#95664),(#95665,#95666)),
 .UNSPECIFIED.,.F.,.F.,.F.)
B_SPLINE_SURFACE_WITH_KNOTS((6,1,1,1,1,1,1,1,1,1,1,1,1,1,1,1,1,1,1,1,1,
1,1,1,1,1,1,1,1,1,6),(2,2),(-1.,-0.966666666666667,-0.933333333333333,-0.9,
-0.866666666666667,-0.833333333333333,-0.8,-0.766666666666667,-0.733333333333333,
-0.7,-0.666666666666667,-0.633333333333333,-0.6,-0.566666666666667,-0.533333333333333,
-0.5,-0.466666666666667,-0.433333333333333,-0.4,-0.366666666666667,-0.333333333333333,
-0.3,-0.266666666666667,-0.233333333333333,-0.2,-0.166666666666667,-0.133333333333333,
-0.1,-0.0666666666666667,-0.0333333333333333,0.),(0.,0.5),.UNSPECIFIED.)
GEOMETRIC_REPRESENTATION_ITEM()
RATIONAL_B_SPLINE_SURFACE(((1.,1.),(1.,1.),(1.,1.),(1.,1.),(1.,1.),(1.,
1.),(1.,1.),(1.,1.),(1.,1.),(1.,1.),(1.,1.),(1.,1.),(1.,1.),(1.,1.),(1.,
1.),(1.,1.),(1.,1.),(1.,1.),(1.,1.),(1.,1.),(1.,1.),(1.,1.),(1.,1.),(1.,
1.),(1.,1.),(1.,1.),(1.,1.),(1.,1.),(1.,1.),(1.,1.),(1.,1.),(1.,1.),(1.,
1.),(1.,1.),(1.,1.)))
REPRESENTATION_ITEM('')
SURFACE()
);
#129=(
BOUNDED_SURFACE()
B_SPLINE_SURFACE(5,1,((#95746,#95747),(#95748,#95749),(#95750,#95751),(#95752,
#95753),(#95754,#95755),(#95756,#95757),(#95758,#95759),(#95760,#95761),
(#95762,#95763),(#95764,#95765),(#95766,#95767),(#95768,#95769),(#95770,
#95771),(#95772,#95773),(#95774,#95775),(#95776,#95777),(#95778,#95779),
(#95780,#95781),(#95782,#95783),(#95784,#95785),(#95786,#95787),(#95788,
#95789),(#95790,#95791),(#95792,#95793),(#95794,#95795),(#95796,#95797),
(#95798,#95799),(#95800,#95801),(#95802,#95803),(#95804,#95805),(#95806,
#95807),(#95808,#95809),(#95810,#95811),(#95812,#95813),(#95814,#95815)),
 .UNSPECIFIED.,.F.,.F.,.F.)
B_SPLINE_SURFACE_WITH_KNOTS((6,1,1,1,1,1,1,1,1,1,1,1,1,1,1,1,1,1,1,1,1,
1,1,1,1,1,1,1,1,1,6),(2,2),(0.,0.0333333333333333,0.0666666666666667,0.1,
0.133333333333333,0.166666666666667,0.2,0.233333333333333,0.266666666666667,
0.3,0.333333333333333,0.366666666666667,0.4,0.433333333333333,0.466666666666667,
0.5,0.533333333333333,0.566666666666667,0.6,0.633333333333333,0.666666666666667,
0.7,0.733333333333333,0.766666666666667,0.8,0.833333333333333,0.866666666666667,
0.9,0.933333333333333,0.966666666666667,1.),(0.,0.5),.UNSPECIFIED.)
GEOMETRIC_REPRESENTATION_ITEM()
RATIONAL_B_SPLINE_SURFACE(((1.,1.),(1.,1.),(1.,1.),(1.,1.),(1.,1.),(1.,
1.),(1.,1.),(1.,1.),(1.,1.),(1.,1.),(1.,1.),(1.,1.),(1.,1.),(1.,1.),(1.,
1.),(1.,1.),(1.,1.),(1.,1.),(1.,1.),(1.,1.),(1.,1.),(1.,1.),(1.,1.),(1.,
1.),(1.,1.),(1.,1.),(1.,1.),(1.,1.),(1.,1.),(1.,1.),(1.,1.),(1.,1.),(1.,
1.),(1.,1.),(1.,1.)))
REPRESENTATION_ITEM('')
SURFACE()
);
#130=(
BOUNDED_SURFACE()
B_SPLINE_SURFACE(5,1,((#95899,#95900),(#95901,#95902),(#95903,#95904),(#95905,
#95906),(#95907,#95908),(#95909,#95910),(#95911,#95912),(#95913,#95914),
(#95915,#95916),(#95917,#95918),(#95919,#95920),(#95921,#95922),(#95923,
#95924),(#95925,#95926),(#95927,#95928),(#95929,#95930),(#95931,#95932),
(#95933,#95934),(#95935,#95936),(#95937,#95938),(#95939,#95940),(#95941,
#95942),(#95943,#95944),(#95945,#95946),(#95947,#95948),(#95949,#95950),
(#95951,#95952),(#95953,#95954),(#95955,#95956),(#95957,#95958),(#95959,
#95960),(#95961,#95962),(#95963,#95964),(#95965,#95966),(#95967,#95968)),
 .UNSPECIFIED.,.F.,.F.,.F.)
B_SPLINE_SURFACE_WITH_KNOTS((6,1,1,1,1,1,1,1,1,1,1,1,1,1,1,1,1,1,1,1,1,
1,1,1,1,1,1,1,1,1,6),(2,2),(-1.,-0.966666666666667,-0.933333333333333,-0.9,
-0.866666666666667,-0.833333333333333,-0.8,-0.766666666666667,-0.733333333333333,
-0.7,-0.666666666666667,-0.633333333333333,-0.6,-0.566666666666667,-0.533333333333333,
-0.5,-0.466666666666667,-0.433333333333333,-0.4,-0.366666666666667,-0.333333333333333,
-0.3,-0.266666666666667,-0.233333333333333,-0.2,-0.166666666666667,-0.133333333333333,
-0.1,-0.0666666666666667,-0.0333333333333333,0.),(0.,0.5),.UNSPECIFIED.)
GEOMETRIC_REPRESENTATION_ITEM()
RATIONAL_B_SPLINE_SURFACE(((1.,1.),(1.,1.),(1.,1.),(1.,1.),(1.,1.),(1.,
1.),(1.,1.),(1.,1.),(1.,1.),(1.,1.),(1.,1.),(1.,1.),(1.,1.),(1.,1.),(1.,
1.),(1.,1.),(1.,1.),(1.,1.),(1.,1.),(1.,1.),(1.,1.),(1.,1.),(1.,1.),(1.,
1.),(1.,1.),(1.,1.),(1.,1.),(1.,1.),(1.,1.),(1.,1.),(1.,1.),(1.,1.),(1.,
1.),(1.,1.),(1.,1.)))
REPRESENTATION_ITEM('')
SURFACE()
);
#131=(
BOUNDED_SURFACE()
B_SPLINE_SURFACE(5,1,((#96048,#96049),(#96050,#96051),(#96052,#96053),(#96054,
#96055),(#96056,#96057),(#96058,#96059),(#96060,#96061),(#96062,#96063),
(#96064,#96065),(#96066,#96067),(#96068,#96069),(#96070,#96071),(#96072,
#96073),(#96074,#96075),(#96076,#96077),(#96078,#96079),(#96080,#96081),
(#96082,#96083),(#96084,#96085),(#96086,#96087),(#96088,#96089),(#96090,
#96091),(#96092,#96093),(#96094,#96095),(#96096,#96097),(#96098,#96099),
(#96100,#96101),(#96102,#96103),(#96104,#96105),(#96106,#96107),(#96108,
#96109),(#96110,#96111),(#96112,#96113),(#96114,#96115),(#96116,#96117)),
 .UNSPECIFIED.,.F.,.F.,.F.)
B_SPLINE_SURFACE_WITH_KNOTS((6,1,1,1,1,1,1,1,1,1,1,1,1,1,1,1,1,1,1,1,1,
1,1,1,1,1,1,1,1,1,6),(2,2),(0.,0.0333333333333333,0.0666666666666667,0.1,
0.133333333333333,0.166666666666667,0.2,0.233333333333333,0.266666666666667,
0.3,0.333333333333333,0.366666666666667,0.4,0.433333333333333,0.466666666666667,
0.5,0.533333333333333,0.566666666666667,0.6,0.633333333333333,0.666666666666667,
0.7,0.733333333333333,0.766666666666667,0.8,0.833333333333333,0.866666666666667,
0.9,0.933333333333333,0.966666666666667,1.),(0.,0.5),.UNSPECIFIED.)
GEOMETRIC_REPRESENTATION_ITEM()
RATIONAL_B_SPLINE_SURFACE(((1.,1.),(1.,1.),(1.,1.),(1.,1.),(1.,1.),(1.,
1.),(1.,1.),(1.,1.),(1.,1.),(1.,1.),(1.,1.),(1.,1.),(1.,1.),(1.,1.),(1.,
1.),(1.,1.),(1.,1.),(1.,1.),(1.,1.),(1.,1.),(1.,1.),(1.,1.),(1.,1.),(1.,
1.),(1.,1.),(1.,1.),(1.,1.),(1.,1.),(1.,1.),(1.,1.),(1.,1.),(1.,1.),(1.,
1.),(1.,1.),(1.,1.)))
REPRESENTATION_ITEM('')
SURFACE()
);
#132=(
BOUNDED_SURFACE()
B_SPLINE_SURFACE(5,1,((#96201,#96202),(#96203,#96204),(#96205,#96206),(#96207,
#96208),(#96209,#96210),(#96211,#96212),(#96213,#96214),(#96215,#96216),
(#96217,#96218),(#96219,#96220),(#96221,#96222),(#96223,#96224),(#96225,
#96226),(#96227,#96228),(#96229,#96230),(#96231,#96232),(#96233,#96234),
(#96235,#96236),(#96237,#96238),(#96239,#96240),(#96241,#96242),(#96243,
#96244),(#96245,#96246),(#96247,#96248),(#96249,#96250),(#96251,#96252),
(#96253,#96254),(#96255,#96256),(#96257,#96258),(#96259,#96260),(#96261,
#96262),(#96263,#96264),(#96265,#96266),(#96267,#96268),(#96269,#96270)),
 .UNSPECIFIED.,.F.,.F.,.F.)
B_SPLINE_SURFACE_WITH_KNOTS((6,1,1,1,1,1,1,1,1,1,1,1,1,1,1,1,1,1,1,1,1,
1,1,1,1,1,1,1,1,1,6),(2,2),(-1.,-0.966666666666667,-0.933333333333333,-0.9,
-0.866666666666667,-0.833333333333333,-0.8,-0.766666666666667,-0.733333333333333,
-0.7,-0.666666666666667,-0.633333333333333,-0.6,-0.566666666666667,-0.533333333333333,
-0.5,-0.466666666666667,-0.433333333333333,-0.4,-0.366666666666667,-0.333333333333333,
-0.3,-0.266666666666667,-0.233333333333333,-0.2,-0.166666666666667,-0.133333333333333,
-0.1,-0.0666666666666667,-0.0333333333333333,0.),(0.,0.5),.UNSPECIFIED.)
GEOMETRIC_REPRESENTATION_ITEM()
RATIONAL_B_SPLINE_SURFACE(((1.,1.),(1.,1.),(1.,1.),(1.,1.),(1.,1.),(1.,
1.),(1.,1.),(1.,1.),(1.,1.),(1.,1.),(1.,1.),(1.,1.),(1.,1.),(1.,1.),(1.,
1.),(1.,1.),(1.,1.),(1.,1.),(1.,1.),(1.,1.),(1.,1.),(1.,1.),(1.,1.),(1.,
1.),(1.,1.),(1.,1.),(1.,1.),(1.,1.),(1.,1.),(1.,1.),(1.,1.),(1.,1.),(1.,
1.),(1.,1.),(1.,1.)))
REPRESENTATION_ITEM('')
SURFACE()
);
#133=(
BOUNDED_SURFACE()
B_SPLINE_SURFACE(5,1,((#96350,#96351),(#96352,#96353),(#96354,#96355),(#96356,
#96357),(#96358,#96359),(#96360,#96361),(#96362,#96363),(#96364,#96365),
(#96366,#96367),(#96368,#96369),(#96370,#96371),(#96372,#96373),(#96374,
#96375),(#96376,#96377),(#96378,#96379),(#96380,#96381),(#96382,#96383),
(#96384,#96385),(#96386,#96387),(#96388,#96389),(#96390,#96391),(#96392,
#96393),(#96394,#96395),(#96396,#96397),(#96398,#96399),(#96400,#96401),
(#96402,#96403),(#96404,#96405),(#96406,#96407),(#96408,#96409),(#96410,
#96411),(#96412,#96413),(#96414,#96415),(#96416,#96417),(#96418,#96419)),
 .UNSPECIFIED.,.F.,.F.,.F.)
B_SPLINE_SURFACE_WITH_KNOTS((6,1,1,1,1,1,1,1,1,1,1,1,1,1,1,1,1,1,1,1,1,
1,1,1,1,1,1,1,1,1,6),(2,2),(0.,0.0333333333333333,0.0666666666666667,0.1,
0.133333333333333,0.166666666666667,0.2,0.233333333333333,0.266666666666667,
0.3,0.333333333333333,0.366666666666667,0.4,0.433333333333333,0.466666666666667,
0.5,0.533333333333333,0.566666666666667,0.6,0.633333333333333,0.666666666666667,
0.7,0.733333333333333,0.766666666666667,0.8,0.833333333333333,0.866666666666667,
0.9,0.933333333333333,0.966666666666667,1.),(0.,0.5),.UNSPECIFIED.)
GEOMETRIC_REPRESENTATION_ITEM()
RATIONAL_B_SPLINE_SURFACE(((1.,1.),(1.,1.),(1.,1.),(1.,1.),(1.,1.),(1.,
1.),(1.,1.),(1.,1.),(1.,1.),(1.,1.),(1.,1.),(1.,1.),(1.,1.),(1.,1.),(1.,
1.),(1.,1.),(1.,1.),(1.,1.),(1.,1.),(1.,1.),(1.,1.),(1.,1.),(1.,1.),(1.,
1.),(1.,1.),(1.,1.),(1.,1.),(1.,1.),(1.,1.),(1.,1.),(1.,1.),(1.,1.),(1.,
1.),(1.,1.),(1.,1.)))
REPRESENTATION_ITEM('')
SURFACE()
);
#134=(
BOUNDED_SURFACE()
B_SPLINE_SURFACE(5,1,((#96503,#96504),(#96505,#96506),(#96507,#96508),(#96509,
#96510),(#96511,#96512),(#96513,#96514),(#96515,#96516),(#96517,#96518),
(#96519,#96520),(#96521,#96522),(#96523,#96524),(#96525,#96526),(#96527,
#96528),(#96529,#96530),(#96531,#96532),(#96533,#96534),(#96535,#96536),
(#96537,#96538),(#96539,#96540),(#96541,#96542),(#96543,#96544),(#96545,
#96546),(#96547,#96548),(#96549,#96550),(#96551,#96552),(#96553,#96554),
(#96555,#96556),(#96557,#96558),(#96559,#96560),(#96561,#96562),(#96563,
#96564),(#96565,#96566),(#96567,#96568),(#96569,#96570),(#96571,#96572)),
 .UNSPECIFIED.,.F.,.F.,.F.)
B_SPLINE_SURFACE_WITH_KNOTS((6,1,1,1,1,1,1,1,1,1,1,1,1,1,1,1,1,1,1,1,1,
1,1,1,1,1,1,1,1,1,6),(2,2),(-1.,-0.966666666666667,-0.933333333333333,-0.9,
-0.866666666666667,-0.833333333333333,-0.8,-0.766666666666667,-0.733333333333333,
-0.7,-0.666666666666667,-0.633333333333333,-0.6,-0.566666666666667,-0.533333333333333,
-0.5,-0.466666666666667,-0.433333333333333,-0.4,-0.366666666666667,-0.333333333333333,
-0.3,-0.266666666666667,-0.233333333333333,-0.2,-0.166666666666667,-0.133333333333333,
-0.1,-0.0666666666666667,-0.0333333333333333,0.),(0.,0.5),.UNSPECIFIED.)
GEOMETRIC_REPRESENTATION_ITEM()
RATIONAL_B_SPLINE_SURFACE(((1.,1.),(1.,1.),(1.,1.),(1.,1.),(1.,1.),(1.,
1.),(1.,1.),(1.,1.),(1.,1.),(1.,1.),(1.,1.),(1.,1.),(1.,1.),(1.,1.),(1.,
1.),(1.,1.),(1.,1.),(1.,1.),(1.,1.),(1.,1.),(1.,1.),(1.,1.),(1.,1.),(1.,
1.),(1.,1.),(1.,1.),(1.,1.),(1.,1.),(1.,1.),(1.,1.),(1.,1.),(1.,1.),(1.,
1.),(1.,1.),(1.,1.)))
REPRESENTATION_ITEM('')
SURFACE()
);
#135=(
BOUNDED_SURFACE()
B_SPLINE_SURFACE(5,1,((#96652,#96653),(#96654,#96655),(#96656,#96657),(#96658,
#96659),(#96660,#96661),(#96662,#96663),(#96664,#96665),(#96666,#96667),
(#96668,#96669),(#96670,#96671),(#96672,#96673),(#96674,#96675),(#96676,
#96677),(#96678,#96679),(#96680,#96681),(#96682,#96683),(#96684,#96685),
(#96686,#96687),(#96688,#96689),(#96690,#96691),(#96692,#96693),(#96694,
#96695),(#96696,#96697),(#96698,#96699),(#96700,#96701),(#96702,#96703),
(#96704,#96705),(#96706,#96707),(#96708,#96709),(#96710,#96711),(#96712,
#96713),(#96714,#96715),(#96716,#96717),(#96718,#96719),(#96720,#96721)),
 .UNSPECIFIED.,.F.,.F.,.F.)
B_SPLINE_SURFACE_WITH_KNOTS((6,1,1,1,1,1,1,1,1,1,1,1,1,1,1,1,1,1,1,1,1,
1,1,1,1,1,1,1,1,1,6),(2,2),(0.,0.0333333333333333,0.0666666666666667,0.1,
0.133333333333333,0.166666666666667,0.2,0.233333333333333,0.266666666666667,
0.3,0.333333333333333,0.366666666666667,0.4,0.433333333333333,0.466666666666667,
0.5,0.533333333333333,0.566666666666667,0.6,0.633333333333333,0.666666666666667,
0.7,0.733333333333333,0.766666666666667,0.8,0.833333333333333,0.866666666666667,
0.9,0.933333333333333,0.966666666666667,1.),(0.,0.5),.UNSPECIFIED.)
GEOMETRIC_REPRESENTATION_ITEM()
RATIONAL_B_SPLINE_SURFACE(((1.,1.),(1.,1.),(1.,1.),(1.,1.),(1.,1.),(1.,
1.),(1.,1.),(1.,1.),(1.,1.),(1.,1.),(1.,1.),(1.,1.),(1.,1.),(1.,1.),(1.,
1.),(1.,1.),(1.,1.),(1.,1.),(1.,1.),(1.,1.),(1.,1.),(1.,1.),(1.,1.),(1.,
1.),(1.,1.),(1.,1.),(1.,1.),(1.,1.),(1.,1.),(1.,1.),(1.,1.),(1.,1.),(1.,
1.),(1.,1.),(1.,1.)))
REPRESENTATION_ITEM('')
SURFACE()
);
#136=(
BOUNDED_SURFACE()
B_SPLINE_SURFACE(5,1,((#96805,#96806),(#96807,#96808),(#96809,#96810),(#96811,
#96812),(#96813,#96814),(#96815,#96816),(#96817,#96818),(#96819,#96820),
(#96821,#96822),(#96823,#96824),(#96825,#96826),(#96827,#96828),(#96829,
#96830),(#96831,#96832),(#96833,#96834),(#96835,#96836),(#96837,#96838),
(#96839,#96840),(#96841,#96842),(#96843,#96844),(#96845,#96846),(#96847,
#96848),(#96849,#96850),(#96851,#96852),(#96853,#96854),(#96855,#96856),
(#96857,#96858),(#96859,#96860),(#96861,#96862),(#96863,#96864),(#96865,
#96866),(#96867,#96868),(#96869,#96870),(#96871,#96872),(#96873,#96874)),
 .UNSPECIFIED.,.F.,.F.,.F.)
B_SPLINE_SURFACE_WITH_KNOTS((6,1,1,1,1,1,1,1,1,1,1,1,1,1,1,1,1,1,1,1,1,
1,1,1,1,1,1,1,1,1,6),(2,2),(-1.,-0.966666666666667,-0.933333333333333,-0.9,
-0.866666666666667,-0.833333333333333,-0.8,-0.766666666666667,-0.733333333333333,
-0.7,-0.666666666666667,-0.633333333333333,-0.6,-0.566666666666667,-0.533333333333333,
-0.5,-0.466666666666667,-0.433333333333333,-0.4,-0.366666666666667,-0.333333333333333,
-0.3,-0.266666666666667,-0.233333333333333,-0.2,-0.166666666666667,-0.133333333333333,
-0.1,-0.0666666666666667,-0.0333333333333333,0.),(0.,0.5),.UNSPECIFIED.)
GEOMETRIC_REPRESENTATION_ITEM()
RATIONAL_B_SPLINE_SURFACE(((1.,1.),(1.,1.),(1.,1.),(1.,1.),(1.,1.),(1.,
1.),(1.,1.),(1.,1.),(1.,1.),(1.,1.),(1.,1.),(1.,1.),(1.,1.),(1.,1.),(1.,
1.),(1.,1.),(1.,1.),(1.,1.),(1.,1.),(1.,1.),(1.,1.),(1.,1.),(1.,1.),(1.,
1.),(1.,1.),(1.,1.),(1.,1.),(1.,1.),(1.,1.),(1.,1.),(1.,1.),(1.,1.),(1.,
1.),(1.,1.),(1.,1.)))
REPRESENTATION_ITEM('')
SURFACE()
);
#137=(
BOUNDED_SURFACE()
B_SPLINE_SURFACE(5,1,((#96954,#96955),(#96956,#96957),(#96958,#96959),(#96960,
#96961),(#96962,#96963),(#96964,#96965),(#96966,#96967),(#96968,#96969),
(#96970,#96971),(#96972,#96973),(#96974,#96975),(#96976,#96977),(#96978,
#96979),(#96980,#96981),(#96982,#96983),(#96984,#96985),(#96986,#96987),
(#96988,#96989),(#96990,#96991),(#96992,#96993),(#96994,#96995),(#96996,
#96997),(#96998,#96999),(#97000,#97001),(#97002,#97003),(#97004,#97005),
(#97006,#97007),(#97008,#97009),(#97010,#97011),(#97012,#97013),(#97014,
#97015),(#97016,#97017),(#97018,#97019),(#97020,#97021),(#97022,#97023)),
 .UNSPECIFIED.,.F.,.F.,.F.)
B_SPLINE_SURFACE_WITH_KNOTS((6,1,1,1,1,1,1,1,1,1,1,1,1,1,1,1,1,1,1,1,1,
1,1,1,1,1,1,1,1,1,6),(2,2),(0.,0.0333333333333333,0.0666666666666667,0.1,
0.133333333333333,0.166666666666667,0.2,0.233333333333333,0.266666666666667,
0.3,0.333333333333333,0.366666666666667,0.4,0.433333333333333,0.466666666666667,
0.5,0.533333333333333,0.566666666666667,0.6,0.633333333333333,0.666666666666667,
0.7,0.733333333333333,0.766666666666667,0.8,0.833333333333333,0.866666666666667,
0.9,0.933333333333333,0.966666666666667,1.),(0.,0.5),.UNSPECIFIED.)
GEOMETRIC_REPRESENTATION_ITEM()
RATIONAL_B_SPLINE_SURFACE(((1.,1.),(1.,1.),(1.,1.),(1.,1.),(1.,1.),(1.,
1.),(1.,1.),(1.,1.),(1.,1.),(1.,1.),(1.,1.),(1.,1.),(1.,1.),(1.,1.),(1.,
1.),(1.,1.),(1.,1.),(1.,1.),(1.,1.),(1.,1.),(1.,1.),(1.,1.),(1.,1.),(1.,
1.),(1.,1.),(1.,1.),(1.,1.),(1.,1.),(1.,1.),(1.,1.),(1.,1.),(1.,1.),(1.,
1.),(1.,1.),(1.,1.)))
REPRESENTATION_ITEM('')
SURFACE()
);
#138=(
BOUNDED_SURFACE()
B_SPLINE_SURFACE(5,1,((#97107,#97108),(#97109,#97110),(#97111,#97112),(#97113,
#97114),(#97115,#97116),(#97117,#97118),(#97119,#97120),(#97121,#97122),
(#97123,#97124),(#97125,#97126),(#97127,#97128),(#97129,#97130),(#97131,
#97132),(#97133,#97134),(#97135,#97136),(#97137,#97138),(#97139,#97140),
(#97141,#97142),(#97143,#97144),(#97145,#97146),(#97147,#97148),(#97149,
#97150),(#97151,#97152),(#97153,#97154),(#97155,#97156),(#97157,#97158),
(#97159,#97160),(#97161,#97162),(#97163,#97164),(#97165,#97166),(#97167,
#97168),(#97169,#97170),(#97171,#97172),(#97173,#97174),(#97175,#97176)),
 .UNSPECIFIED.,.F.,.F.,.F.)
B_SPLINE_SURFACE_WITH_KNOTS((6,1,1,1,1,1,1,1,1,1,1,1,1,1,1,1,1,1,1,1,1,
1,1,1,1,1,1,1,1,1,6),(2,2),(-1.,-0.966666666666667,-0.933333333333333,-0.9,
-0.866666666666667,-0.833333333333333,-0.8,-0.766666666666667,-0.733333333333333,
-0.7,-0.666666666666667,-0.633333333333333,-0.6,-0.566666666666667,-0.533333333333333,
-0.5,-0.466666666666667,-0.433333333333333,-0.4,-0.366666666666667,-0.333333333333333,
-0.3,-0.266666666666667,-0.233333333333333,-0.2,-0.166666666666667,-0.133333333333333,
-0.1,-0.0666666666666667,-0.0333333333333333,0.),(0.,0.5),.UNSPECIFIED.)
GEOMETRIC_REPRESENTATION_ITEM()
RATIONAL_B_SPLINE_SURFACE(((1.,1.),(1.,1.),(1.,1.),(1.,1.),(1.,1.),(1.,
1.),(1.,1.),(1.,1.),(1.,1.),(1.,1.),(1.,1.),(1.,1.),(1.,1.),(1.,1.),(1.,
1.),(1.,1.),(1.,1.),(1.,1.),(1.,1.),(1.,1.),(1.,1.),(1.,1.),(1.,1.),(1.,
1.),(1.,1.),(1.,1.),(1.,1.),(1.,1.),(1.,1.),(1.,1.),(1.,1.),(1.,1.),(1.,
1.),(1.,1.),(1.,1.)))
REPRESENTATION_ITEM('')
SURFACE()
);
#139=(
BOUNDED_SURFACE()
B_SPLINE_SURFACE(5,1,((#97256,#97257),(#97258,#97259),(#97260,#97261),(#97262,
#97263),(#97264,#97265),(#97266,#97267),(#97268,#97269),(#97270,#97271),
(#97272,#97273),(#97274,#97275),(#97276,#97277),(#97278,#97279),(#97280,
#97281),(#97282,#97283),(#97284,#97285),(#97286,#97287),(#97288,#97289),
(#97290,#97291),(#97292,#97293),(#97294,#97295),(#97296,#97297),(#97298,
#97299),(#97300,#97301),(#97302,#97303),(#97304,#97305),(#97306,#97307),
(#97308,#97309),(#97310,#97311),(#97312,#97313),(#97314,#97315),(#97316,
#97317),(#97318,#97319),(#97320,#97321),(#97322,#97323),(#97324,#97325)),
 .UNSPECIFIED.,.F.,.F.,.F.)
B_SPLINE_SURFACE_WITH_KNOTS((6,1,1,1,1,1,1,1,1,1,1,1,1,1,1,1,1,1,1,1,1,
1,1,1,1,1,1,1,1,1,6),(2,2),(0.,0.0333333333333333,0.0666666666666667,0.1,
0.133333333333333,0.166666666666667,0.2,0.233333333333333,0.266666666666667,
0.3,0.333333333333333,0.366666666666667,0.4,0.433333333333333,0.466666666666667,
0.5,0.533333333333333,0.566666666666667,0.6,0.633333333333333,0.666666666666667,
0.7,0.733333333333333,0.766666666666667,0.8,0.833333333333333,0.866666666666667,
0.9,0.933333333333333,0.966666666666667,1.),(0.,0.5),.UNSPECIFIED.)
GEOMETRIC_REPRESENTATION_ITEM()
RATIONAL_B_SPLINE_SURFACE(((1.,1.),(1.,1.),(1.,1.),(1.,1.),(1.,1.),(1.,
1.),(1.,1.),(1.,1.),(1.,1.),(1.,1.),(1.,1.),(1.,1.),(1.,1.),(1.,1.),(1.,
1.),(1.,1.),(1.,1.),(1.,1.),(1.,1.),(1.,1.),(1.,1.),(1.,1.),(1.,1.),(1.,
1.),(1.,1.),(1.,1.),(1.,1.),(1.,1.),(1.,1.),(1.,1.),(1.,1.),(1.,1.),(1.,
1.),(1.,1.),(1.,1.)))
REPRESENTATION_ITEM('')
SURFACE()
);
#140=(
BOUNDED_SURFACE()
B_SPLINE_SURFACE(5,1,((#97403,#97404),(#97405,#97406),(#97407,#97408),(#97409,
#97410),(#97411,#97412),(#97413,#97414),(#97415,#97416),(#97417,#97418),
(#97419,#97420),(#97421,#97422),(#97423,#97424),(#97425,#97426),(#97427,
#97428),(#97429,#97430),(#97431,#97432),(#97433,#97434),(#97435,#97436),
(#97437,#97438),(#97439,#97440),(#97441,#97442),(#97443,#97444),(#97445,
#97446),(#97447,#97448),(#97449,#97450),(#97451,#97452),(#97453,#97454),
(#97455,#97456),(#97457,#97458),(#97459,#97460),(#97461,#97462),(#97463,
#97464),(#97465,#97466),(#97467,#97468),(#97469,#97470),(#97471,#97472)),
 .UNSPECIFIED.,.F.,.F.,.F.)
B_SPLINE_SURFACE_WITH_KNOTS((6,1,1,1,1,1,1,1,1,1,1,1,1,1,1,1,1,1,1,1,1,
1,1,1,1,1,1,1,1,1,6),(2,2),(-1.,-0.966666666666667,-0.933333333333333,-0.9,
-0.866666666666667,-0.833333333333333,-0.8,-0.766666666666667,-0.733333333333333,
-0.7,-0.666666666666667,-0.633333333333333,-0.6,-0.566666666666667,-0.533333333333333,
-0.5,-0.466666666666667,-0.433333333333333,-0.4,-0.366666666666667,-0.333333333333333,
-0.3,-0.266666666666667,-0.233333333333333,-0.2,-0.166666666666667,-0.133333333333333,
-0.1,-0.0666666666666667,-0.0333333333333333,0.),(0.,0.5),.UNSPECIFIED.)
GEOMETRIC_REPRESENTATION_ITEM()
RATIONAL_B_SPLINE_SURFACE(((1.,1.),(1.,1.),(1.,1.),(1.,1.),(1.,1.),(1.,
1.),(1.,1.),(1.,1.),(1.,1.),(1.,1.),(1.,1.),(1.,1.),(1.,1.),(1.,1.),(1.,
1.),(1.,1.),(1.,1.),(1.,1.),(1.,1.),(1.,1.),(1.,1.),(1.,1.),(1.,1.),(1.,
1.),(1.,1.),(1.,1.),(1.,1.),(1.,1.),(1.,1.),(1.,1.),(1.,1.),(1.,1.),(1.,
1.),(1.,1.),(1.,1.)))
REPRESENTATION_ITEM('')
SURFACE()
);
#141=(
BOUNDED_SURFACE()
B_SPLINE_SURFACE(5,1,((#97552,#97553),(#97554,#97555),(#97556,#97557),(#97558,
#97559),(#97560,#97561),(#97562,#97563),(#97564,#97565),(#97566,#97567),
(#97568,#97569),(#97570,#97571),(#97572,#97573),(#97574,#97575),(#97576,
#97577),(#97578,#97579),(#97580,#97581),(#97582,#97583),(#97584,#97585),
(#97586,#97587),(#97588,#97589),(#97590,#97591),(#97592,#97593),(#97594,
#97595),(#97596,#97597),(#97598,#97599),(#97600,#97601),(#97602,#97603),
(#97604,#97605),(#97606,#97607),(#97608,#97609),(#97610,#97611),(#97612,
#97613),(#97614,#97615),(#97616,#97617),(#97618,#97619),(#97620,#97621)),
 .UNSPECIFIED.,.F.,.F.,.F.)
B_SPLINE_SURFACE_WITH_KNOTS((6,1,1,1,1,1,1,1,1,1,1,1,1,1,1,1,1,1,1,1,1,
1,1,1,1,1,1,1,1,1,6),(2,2),(0.,0.0333333333333333,0.0666666666666667,0.1,
0.133333333333333,0.166666666666667,0.2,0.233333333333333,0.266666666666667,
0.3,0.333333333333333,0.366666666666667,0.4,0.433333333333333,0.466666666666667,
0.5,0.533333333333333,0.566666666666667,0.6,0.633333333333333,0.666666666666667,
0.7,0.733333333333333,0.766666666666667,0.8,0.833333333333333,0.866666666666667,
0.9,0.933333333333333,0.966666666666667,1.),(0.,0.5),.UNSPECIFIED.)
GEOMETRIC_REPRESENTATION_ITEM()
RATIONAL_B_SPLINE_SURFACE(((1.,1.),(1.,1.),(1.,1.),(1.,1.),(1.,1.),(1.,
1.),(1.,1.),(1.,1.),(1.,1.),(1.,1.),(1.,1.),(1.,1.),(1.,1.),(1.,1.),(1.,
1.),(1.,1.),(1.,1.),(1.,1.),(1.,1.),(1.,1.),(1.,1.),(1.,1.),(1.,1.),(1.,
1.),(1.,1.),(1.,1.),(1.,1.),(1.,1.),(1.,1.),(1.,1.),(1.,1.),(1.,1.),(1.,
1.),(1.,1.),(1.,1.)))
REPRESENTATION_ITEM('')
SURFACE()
);
#147=(
BOUNDED_CURVE()
B_SPLINE_CURVE(5,(#92822,#92823,#92824,#92825,#92826,#92827,#92828,#92829,
#92830,#92831,#92832,#92833,#92834,#92835,#92836,#92837,#92838,#92839,#92840,
#92841,#92842,#92843,#92844,#92845,#92846,#92847,#92848,#92849,#92850,#92851,
#92852,#92853,#92854,#92855,#92856),.UNSPECIFIED.,.F.,.F.)
B_SPLINE_CURVE_WITH_KNOTS((6,1,1,1,1,1,1,1,1,1,1,1,1,1,1,1,1,1,1,1,1,1,
1,1,1,1,1,1,1,1,6),(0.,0.0333333333333333,0.0666666666666667,0.1,0.133333333333333,
0.166666666666667,0.2,0.233333333333333,0.266666666666667,0.3,0.333333333333333,
0.366666666666667,0.4,0.433333333333333,0.466666666666667,0.5,0.533333333333333,
0.566666666666667,0.6,0.633333333333333,0.666666666666667,0.7,0.733333333333333,
0.766666666666667,0.8,0.833333333333333,0.866666666666667,0.9,0.933333333333333,
0.966666666666667,1.),.UNSPECIFIED.)
CURVE()
GEOMETRIC_REPRESENTATION_ITEM()
RATIONAL_B_SPLINE_CURVE((1.,1.,1.,1.,1.,1.,1.,1.,1.,1.,1.,1.,1.,1.,1.,1.,
1.,1.,1.,1.,1.,1.,1.,1.,1.,1.,1.,1.,1.,1.,1.,1.,1.,1.,1.))
REPRESENTATION_ITEM('')
);
#148=(
BOUNDED_CURVE()
B_SPLINE_CURVE(5,(#92858,#92859,#92860,#92861,#92862,#92863,#92864,#92865,
#92866,#92867,#92868,#92869,#92870,#92871,#92872,#92873,#92874,#92875,#92876,
#92877,#92878,#92879,#92880,#92881,#92882,#92883,#92884,#92885,#92886,#92887,
#92888,#92889,#92890,#92891,#92892),.UNSPECIFIED.,.F.,.F.)
B_SPLINE_CURVE_WITH_KNOTS((6,1,1,1,1,1,1,1,1,1,1,1,1,1,1,1,1,1,1,1,1,1,
1,1,1,1,1,1,1,1,6),(-1.,-0.966666666666667,-0.933333333333333,-0.9,-0.866666666666667,
-0.833333333333333,-0.8,-0.766666666666667,-0.733333333333333,-0.7,-0.666666666666667,
-0.633333333333333,-0.6,-0.566666666666667,-0.533333333333333,-0.5,-0.466666666666667,
-0.433333333333333,-0.4,-0.366666666666667,-0.333333333333333,-0.3,-0.266666666666667,
-0.233333333333333,-0.2,-0.166666666666667,-0.133333333333333,-0.1,-0.0666666666666667,
-0.0333333333333333,0.),.UNSPECIFIED.)
CURVE()
GEOMETRIC_REPRESENTATION_ITEM()
RATIONAL_B_SPLINE_CURVE((1.,1.,1.,1.,1.,1.,1.,1.,1.,1.,1.,1.,1.,1.,1.,1.,
1.,1.,1.,1.,1.,1.,1.,1.,1.,1.,1.,1.,1.,1.,1.,1.,1.,1.,1.))
REPRESENTATION_ITEM('')
);
#149=(
BOUNDED_CURVE()
B_SPLINE_CURVE(5,(#92970,#92971,#92972,#92973,#92974,#92975,#92976,#92977,
#92978,#92979,#92980,#92981,#92982,#92983,#92984,#92985,#92986,#92987,#92988,
#92989,#92990,#92991,#92992,#92993,#92994,#92995,#92996,#92997,#92998,#92999,
#93000,#93001,#93002,#93003,#93004),.UNSPECIFIED.,.F.,.F.)
B_SPLINE_CURVE_WITH_KNOTS((6,1,1,1,1,1,1,1,1,1,1,1,1,1,1,1,1,1,1,1,1,1,
1,1,1,1,1,1,1,1,6),(0.,0.0333333333333333,0.0666666666666667,0.1,0.133333333333333,
0.166666666666667,0.2,0.233333333333333,0.266666666666667,0.3,0.333333333333333,
0.366666666666667,0.4,0.433333333333333,0.466666666666667,0.5,0.533333333333333,
0.566666666666667,0.6,0.633333333333333,0.666666666666667,0.7,0.733333333333333,
0.766666666666667,0.8,0.833333333333333,0.866666666666667,0.9,0.933333333333333,
0.966666666666667,1.),.UNSPECIFIED.)
CURVE()
GEOMETRIC_REPRESENTATION_ITEM()
RATIONAL_B_SPLINE_CURVE((1.,1.,1.,1.,1.,1.,1.,1.,1.,1.,1.,1.,1.,1.,1.,1.,
1.,1.,1.,1.,1.,1.,1.,1.,1.,1.,1.,1.,1.,1.,1.,1.,1.,1.,1.))
REPRESENTATION_ITEM('')
);
#150=(
BOUNDED_CURVE()
B_SPLINE_CURVE(5,(#93005,#93006,#93007,#93008,#93009,#93010,#93011,#93012,
#93013,#93014,#93015,#93016,#93017,#93018,#93019,#93020,#93021,#93022,#93023,
#93024,#93025,#93026,#93027,#93028,#93029,#93030,#93031,#93032,#93033,#93034,
#93035,#93036,#93037,#93038,#93039),.UNSPECIFIED.,.F.,.F.)
B_SPLINE_CURVE_WITH_KNOTS((6,1,1,1,1,1,1,1,1,1,1,1,1,1,1,1,1,1,1,1,1,1,
1,1,1,1,1,1,1,1,6),(0.,0.0333333333333333,0.0666666666666667,0.1,0.133333333333333,
0.166666666666667,0.2,0.233333333333333,0.266666666666667,0.3,0.333333333333333,
0.366666666666667,0.4,0.433333333333333,0.466666666666667,0.5,0.533333333333333,
0.566666666666667,0.6,0.633333333333333,0.666666666666667,0.7,0.733333333333333,
0.766666666666667,0.8,0.833333333333333,0.866666666666667,0.9,0.933333333333333,
0.966666666666667,1.),.UNSPECIFIED.)
CURVE()
GEOMETRIC_REPRESENTATION_ITEM()
RATIONAL_B_SPLINE_CURVE((1.,1.,1.,1.,1.,1.,1.,1.,1.,1.,1.,1.,1.,1.,1.,1.,
1.,1.,1.,1.,1.,1.,1.,1.,1.,1.,1.,1.,1.,1.,1.,1.,1.,1.,1.))
REPRESENTATION_ITEM('')
);
#151=(
BOUNDED_CURVE()
B_SPLINE_CURVE(5,(#93252,#93253,#93254,#93255,#93256,#93257,#93258,#93259,
#93260,#93261,#93262,#93263,#93264,#93265,#93266,#93267,#93268,#93269,#93270,
#93271,#93272,#93273,#93274,#93275,#93276,#93277,#93278,#93279,#93280,#93281,
#93282,#93283,#93284,#93285,#93286),.UNSPECIFIED.,.F.,.F.)
B_SPLINE_CURVE_WITH_KNOTS((6,1,1,1,1,1,1,1,1,1,1,1,1,1,1,1,1,1,1,1,1,1,
1,1,1,1,1,1,1,1,6),(0.,0.0333333333333333,0.0666666666666667,0.1,0.133333333333333,
0.166666666666667,0.2,0.233333333333333,0.266666666666667,0.3,0.333333333333333,
0.366666666666667,0.4,0.433333333333333,0.466666666666667,0.5,0.533333333333333,
0.566666666666667,0.6,0.633333333333333,0.666666666666667,0.7,0.733333333333333,
0.766666666666667,0.8,0.833333333333333,0.866666666666667,0.9,0.933333333333333,
0.966666666666667,1.),.UNSPECIFIED.)
CURVE()
GEOMETRIC_REPRESENTATION_ITEM()
RATIONAL_B_SPLINE_CURVE((1.,1.,1.,1.,1.,1.,1.,1.,1.,1.,1.,1.,1.,1.,1.,1.,
1.,1.,1.,1.,1.,1.,1.,1.,1.,1.,1.,1.,1.,1.,1.,1.,1.,1.,1.))
REPRESENTATION_ITEM('')
);
#152=(
BOUNDED_CURVE()
B_SPLINE_CURVE(5,(#93288,#93289,#93290,#93291,#93292,#93293,#93294,#93295,
#93296,#93297,#93298,#93299,#93300,#93301,#93302,#93303,#93304,#93305,#93306,
#93307,#93308,#93309,#93310,#93311,#93312,#93313,#93314,#93315,#93316,#93317,
#93318,#93319,#93320,#93321,#93322),.UNSPECIFIED.,.F.,.F.)
B_SPLINE_CURVE_WITH_KNOTS((6,1,1,1,1,1,1,1,1,1,1,1,1,1,1,1,1,1,1,1,1,1,
1,1,1,1,1,1,1,1,6),(-1.,-0.966666666666667,-0.933333333333333,-0.9,-0.866666666666667,
-0.833333333333333,-0.8,-0.766666666666667,-0.733333333333333,-0.7,-0.666666666666667,
-0.633333333333333,-0.6,-0.566666666666667,-0.533333333333333,-0.5,-0.466666666666667,
-0.433333333333333,-0.4,-0.366666666666667,-0.333333333333333,-0.3,-0.266666666666667,
-0.233333333333333,-0.2,-0.166666666666667,-0.133333333333333,-0.1,-0.0666666666666667,
-0.0333333333333333,0.),.UNSPECIFIED.)
CURVE()
GEOMETRIC_REPRESENTATION_ITEM()
RATIONAL_B_SPLINE_CURVE((1.,1.,1.,1.,1.,1.,1.,1.,1.,1.,1.,1.,1.,1.,1.,1.,
1.,1.,1.,1.,1.,1.,1.,1.,1.,1.,1.,1.,1.,1.,1.,1.,1.,1.,1.))
REPRESENTATION_ITEM('')
);
#153=(
BOUNDED_CURVE()
B_SPLINE_CURVE(5,(#93400,#93401,#93402,#93403,#93404,#93405,#93406,#93407,
#93408,#93409,#93410,#93411,#93412,#93413,#93414,#93415,#93416,#93417,#93418,
#93419,#93420,#93421,#93422,#93423,#93424,#93425,#93426,#93427,#93428,#93429,
#93430,#93431,#93432,#93433,#93434),.UNSPECIFIED.,.F.,.F.)
B_SPLINE_CURVE_WITH_KNOTS((6,1,1,1,1,1,1,1,1,1,1,1,1,1,1,1,1,1,1,1,1,1,
1,1,1,1,1,1,1,1,6),(0.,0.0333333333333333,0.0666666666666667,0.1,0.133333333333333,
0.166666666666667,0.2,0.233333333333333,0.266666666666667,0.3,0.333333333333333,
0.366666666666667,0.4,0.433333333333333,0.466666666666667,0.5,0.533333333333333,
0.566666666666667,0.6,0.633333333333333,0.666666666666667,0.7,0.733333333333333,
0.766666666666667,0.8,0.833333333333333,0.866666666666667,0.9,0.933333333333333,
0.966666666666667,1.),.UNSPECIFIED.)
CURVE()
GEOMETRIC_REPRESENTATION_ITEM()
RATIONAL_B_SPLINE_CURVE((1.,1.,1.,1.,1.,1.,1.,1.,1.,1.,1.,1.,1.,1.,1.,1.,
1.,1.,1.,1.,1.,1.,1.,1.,1.,1.,1.,1.,1.,1.,1.,1.,1.,1.,1.))
REPRESENTATION_ITEM('')
);
#154=(
BOUNDED_CURVE()
B_SPLINE_CURVE(5,(#93435,#93436,#93437,#93438,#93439,#93440,#93441,#93442,
#93443,#93444,#93445,#93446,#93447,#93448,#93449,#93450,#93451,#93452,#93453,
#93454,#93455,#93456,#93457,#93458,#93459,#93460,#93461,#93462,#93463,#93464,
#93465,#93466,#93467,#93468,#93469),.UNSPECIFIED.,.F.,.F.)
B_SPLINE_CURVE_WITH_KNOTS((6,1,1,1,1,1,1,1,1,1,1,1,1,1,1,1,1,1,1,1,1,1,
1,1,1,1,1,1,1,1,6),(0.,0.0333333333333333,0.0666666666666667,0.1,0.133333333333333,
0.166666666666667,0.2,0.233333333333333,0.266666666666667,0.3,0.333333333333333,
0.366666666666667,0.4,0.433333333333333,0.466666666666667,0.5,0.533333333333333,
0.566666666666667,0.6,0.633333333333333,0.666666666666667,0.7,0.733333333333333,
0.766666666666667,0.8,0.833333333333333,0.866666666666667,0.9,0.933333333333333,
0.966666666666667,1.),.UNSPECIFIED.)
CURVE()
GEOMETRIC_REPRESENTATION_ITEM()
RATIONAL_B_SPLINE_CURVE((1.,1.,1.,1.,1.,1.,1.,1.,1.,1.,1.,1.,1.,1.,1.,1.,
1.,1.,1.,1.,1.,1.,1.,1.,1.,1.,1.,1.,1.,1.,1.,1.,1.,1.,1.))
REPRESENTATION_ITEM('')
);
#155=(
BOUNDED_CURVE()
B_SPLINE_CURVE(5,(#93554,#93555,#93556,#93557,#93558,#93559,#93560,#93561,
#93562,#93563,#93564,#93565,#93566,#93567,#93568,#93569,#93570,#93571,#93572,
#93573,#93574,#93575,#93576,#93577,#93578,#93579,#93580,#93581,#93582,#93583,
#93584,#93585,#93586,#93587,#93588),.UNSPECIFIED.,.F.,.F.)
B_SPLINE_CURVE_WITH_KNOTS((6,1,1,1,1,1,1,1,1,1,1,1,1,1,1,1,1,1,1,1,1,1,
1,1,1,1,1,1,1,1,6),(0.,0.0333333333333333,0.0666666666666667,0.1,0.133333333333333,
0.166666666666667,0.2,0.233333333333333,0.266666666666667,0.3,0.333333333333333,
0.366666666666667,0.4,0.433333333333333,0.466666666666667,0.5,0.533333333333333,
0.566666666666667,0.6,0.633333333333333,0.666666666666667,0.7,0.733333333333333,
0.766666666666667,0.8,0.833333333333333,0.866666666666667,0.9,0.933333333333333,
0.966666666666667,1.),.UNSPECIFIED.)
CURVE()
GEOMETRIC_REPRESENTATION_ITEM()
RATIONAL_B_SPLINE_CURVE((1.,1.,1.,1.,1.,1.,1.,1.,1.,1.,1.,1.,1.,1.,1.,1.,
1.,1.,1.,1.,1.,1.,1.,1.,1.,1.,1.,1.,1.,1.,1.,1.,1.,1.,1.))
REPRESENTATION_ITEM('')
);
#156=(
BOUNDED_CURVE()
B_SPLINE_CURVE(5,(#93590,#93591,#93592,#93593,#93594,#93595,#93596,#93597,
#93598,#93599,#93600,#93601,#93602,#93603,#93604,#93605,#93606,#93607,#93608,
#93609,#93610,#93611,#93612,#93613,#93614,#93615,#93616,#93617,#93618,#93619,
#93620,#93621,#93622,#93623,#93624),.UNSPECIFIED.,.F.,.F.)
B_SPLINE_CURVE_WITH_KNOTS((6,1,1,1,1,1,1,1,1,1,1,1,1,1,1,1,1,1,1,1,1,1,
1,1,1,1,1,1,1,1,6),(-1.,-0.966666666666667,-0.933333333333333,-0.9,-0.866666666666667,
-0.833333333333333,-0.8,-0.766666666666667,-0.733333333333333,-0.7,-0.666666666666667,
-0.633333333333333,-0.6,-0.566666666666667,-0.533333333333333,-0.5,-0.466666666666667,
-0.433333333333333,-0.4,-0.366666666666667,-0.333333333333333,-0.3,-0.266666666666667,
-0.233333333333333,-0.2,-0.166666666666667,-0.133333333333333,-0.1,-0.0666666666666667,
-0.0333333333333333,0.),.UNSPECIFIED.)
CURVE()
GEOMETRIC_REPRESENTATION_ITEM()
RATIONAL_B_SPLINE_CURVE((1.,1.,1.,1.,1.,1.,1.,1.,1.,1.,1.,1.,1.,1.,1.,1.,
1.,1.,1.,1.,1.,1.,1.,1.,1.,1.,1.,1.,1.,1.,1.,1.,1.,1.,1.))
REPRESENTATION_ITEM('')
);
#157=(
BOUNDED_CURVE()
B_SPLINE_CURVE(5,(#93702,#93703,#93704,#93705,#93706,#93707,#93708,#93709,
#93710,#93711,#93712,#93713,#93714,#93715,#93716,#93717,#93718,#93719,#93720,
#93721,#93722,#93723,#93724,#93725,#93726,#93727,#93728,#93729,#93730,#93731,
#93732,#93733,#93734,#93735,#93736),.UNSPECIFIED.,.F.,.F.)
B_SPLINE_CURVE_WITH_KNOTS((6,1,1,1,1,1,1,1,1,1,1,1,1,1,1,1,1,1,1,1,1,1,
1,1,1,1,1,1,1,1,6),(0.,0.0333333333333333,0.0666666666666667,0.1,0.133333333333333,
0.166666666666667,0.2,0.233333333333333,0.266666666666667,0.3,0.333333333333333,
0.366666666666667,0.4,0.433333333333333,0.466666666666667,0.5,0.533333333333333,
0.566666666666667,0.6,0.633333333333333,0.666666666666667,0.7,0.733333333333333,
0.766666666666667,0.8,0.833333333333333,0.866666666666667,0.9,0.933333333333333,
0.966666666666667,1.),.UNSPECIFIED.)
CURVE()
GEOMETRIC_REPRESENTATION_ITEM()
RATIONAL_B_SPLINE_CURVE((1.,1.,1.,1.,1.,1.,1.,1.,1.,1.,1.,1.,1.,1.,1.,1.,
1.,1.,1.,1.,1.,1.,1.,1.,1.,1.,1.,1.,1.,1.,1.,1.,1.,1.,1.))
REPRESENTATION_ITEM('')
);
#158=(
BOUNDED_CURVE()
B_SPLINE_CURVE(5,(#93737,#93738,#93739,#93740,#93741,#93742,#93743,#93744,
#93745,#93746,#93747,#93748,#93749,#93750,#93751,#93752,#93753,#93754,#93755,
#93756,#93757,#93758,#93759,#93760,#93761,#93762,#93763,#93764,#93765,#93766,
#93767,#93768,#93769,#93770,#93771),.UNSPECIFIED.,.F.,.F.)
B_SPLINE_CURVE_WITH_KNOTS((6,1,1,1,1,1,1,1,1,1,1,1,1,1,1,1,1,1,1,1,1,1,
1,1,1,1,1,1,1,1,6),(0.,0.0333333333333333,0.0666666666666667,0.1,0.133333333333333,
0.166666666666667,0.2,0.233333333333333,0.266666666666667,0.3,0.333333333333333,
0.366666666666667,0.4,0.433333333333333,0.466666666666667,0.5,0.533333333333333,
0.566666666666667,0.6,0.633333333333333,0.666666666666667,0.7,0.733333333333333,
0.766666666666667,0.8,0.833333333333333,0.866666666666667,0.9,0.933333333333333,
0.966666666666667,1.),.UNSPECIFIED.)
CURVE()
GEOMETRIC_REPRESENTATION_ITEM()
RATIONAL_B_SPLINE_CURVE((1.,1.,1.,1.,1.,1.,1.,1.,1.,1.,1.,1.,1.,1.,1.,1.,
1.,1.,1.,1.,1.,1.,1.,1.,1.,1.,1.,1.,1.,1.,1.,1.,1.,1.,1.))
REPRESENTATION_ITEM('')
);
#159=(
BOUNDED_CURVE()
B_SPLINE_CURVE(5,(#93856,#93857,#93858,#93859,#93860,#93861,#93862,#93863,
#93864,#93865,#93866,#93867,#93868,#93869,#93870,#93871,#93872,#93873,#93874,
#93875,#93876,#93877,#93878,#93879,#93880,#93881,#93882,#93883,#93884,#93885,
#93886,#93887,#93888,#93889,#93890),.UNSPECIFIED.,.F.,.F.)
B_SPLINE_CURVE_WITH_KNOTS((6,1,1,1,1,1,1,1,1,1,1,1,1,1,1,1,1,1,1,1,1,1,
1,1,1,1,1,1,1,1,6),(0.,0.0333333333333333,0.0666666666666667,0.1,0.133333333333333,
0.166666666666667,0.2,0.233333333333333,0.266666666666667,0.3,0.333333333333333,
0.366666666666667,0.4,0.433333333333333,0.466666666666667,0.5,0.533333333333333,
0.566666666666667,0.6,0.633333333333333,0.666666666666667,0.7,0.733333333333333,
0.766666666666667,0.8,0.833333333333333,0.866666666666667,0.9,0.933333333333333,
0.966666666666667,1.),.UNSPECIFIED.)
CURVE()
GEOMETRIC_REPRESENTATION_ITEM()
RATIONAL_B_SPLINE_CURVE((1.,1.,1.,1.,1.,1.,1.,1.,1.,1.,1.,1.,1.,1.,1.,1.,
1.,1.,1.,1.,1.,1.,1.,1.,1.,1.,1.,1.,1.,1.,1.,1.,1.,1.,1.))
REPRESENTATION_ITEM('')
);
#160=(
BOUNDED_CURVE()
B_SPLINE_CURVE(5,(#93892,#93893,#93894,#93895,#93896,#93897,#93898,#93899,
#93900,#93901,#93902,#93903,#93904,#93905,#93906,#93907,#93908,#93909,#93910,
#93911,#93912,#93913,#93914,#93915,#93916,#93917,#93918,#93919,#93920,#93921,
#93922,#93923,#93924,#93925,#93926),.UNSPECIFIED.,.F.,.F.)
B_SPLINE_CURVE_WITH_KNOTS((6,1,1,1,1,1,1,1,1,1,1,1,1,1,1,1,1,1,1,1,1,1,
1,1,1,1,1,1,1,1,6),(-1.,-0.966666666666667,-0.933333333333333,-0.9,-0.866666666666667,
-0.833333333333333,-0.8,-0.766666666666667,-0.733333333333333,-0.7,-0.666666666666667,
-0.633333333333333,-0.6,-0.566666666666667,-0.533333333333333,-0.5,-0.466666666666667,
-0.433333333333333,-0.4,-0.366666666666667,-0.333333333333333,-0.3,-0.266666666666667,
-0.233333333333333,-0.2,-0.166666666666667,-0.133333333333333,-0.1,-0.0666666666666667,
-0.0333333333333333,0.),.UNSPECIFIED.)
CURVE()
GEOMETRIC_REPRESENTATION_ITEM()
RATIONAL_B_SPLINE_CURVE((1.,1.,1.,1.,1.,1.,1.,1.,1.,1.,1.,1.,1.,1.,1.,1.,
1.,1.,1.,1.,1.,1.,1.,1.,1.,1.,1.,1.,1.,1.,1.,1.,1.,1.,1.))
REPRESENTATION_ITEM('')
);
#161=(
BOUNDED_CURVE()
B_SPLINE_CURVE(5,(#94004,#94005,#94006,#94007,#94008,#94009,#94010,#94011,
#94012,#94013,#94014,#94015,#94016,#94017,#94018,#94019,#94020,#94021,#94022,
#94023,#94024,#94025,#94026,#94027,#94028,#94029,#94030,#94031,#94032,#94033,
#94034,#94035,#94036,#94037,#94038),.UNSPECIFIED.,.F.,.F.)
B_SPLINE_CURVE_WITH_KNOTS((6,1,1,1,1,1,1,1,1,1,1,1,1,1,1,1,1,1,1,1,1,1,
1,1,1,1,1,1,1,1,6),(0.,0.0333333333333333,0.0666666666666667,0.1,0.133333333333333,
0.166666666666667,0.2,0.233333333333333,0.266666666666667,0.3,0.333333333333333,
0.366666666666667,0.4,0.433333333333333,0.466666666666667,0.5,0.533333333333333,
0.566666666666667,0.6,0.633333333333333,0.666666666666667,0.7,0.733333333333333,
0.766666666666667,0.8,0.833333333333333,0.866666666666667,0.9,0.933333333333333,
0.966666666666667,1.),.UNSPECIFIED.)
CURVE()
GEOMETRIC_REPRESENTATION_ITEM()
RATIONAL_B_SPLINE_CURVE((1.,1.,1.,1.,1.,1.,1.,1.,1.,1.,1.,1.,1.,1.,1.,1.,
1.,1.,1.,1.,1.,1.,1.,1.,1.,1.,1.,1.,1.,1.,1.,1.,1.,1.,1.))
REPRESENTATION_ITEM('')
);
#162=(
BOUNDED_CURVE()
B_SPLINE_CURVE(5,(#94039,#94040,#94041,#94042,#94043,#94044,#94045,#94046,
#94047,#94048,#94049,#94050,#94051,#94052,#94053,#94054,#94055,#94056,#94057,
#94058,#94059,#94060,#94061,#94062,#94063,#94064,#94065,#94066,#94067,#94068,
#94069,#94070,#94071,#94072,#94073),.UNSPECIFIED.,.F.,.F.)
B_SPLINE_CURVE_WITH_KNOTS((6,1,1,1,1,1,1,1,1,1,1,1,1,1,1,1,1,1,1,1,1,1,
1,1,1,1,1,1,1,1,6),(0.,0.0333333333333333,0.0666666666666667,0.1,0.133333333333333,
0.166666666666667,0.2,0.233333333333333,0.266666666666667,0.3,0.333333333333333,
0.366666666666667,0.4,0.433333333333333,0.466666666666667,0.5,0.533333333333333,
0.566666666666667,0.6,0.633333333333333,0.666666666666667,0.7,0.733333333333333,
0.766666666666667,0.8,0.833333333333333,0.866666666666667,0.9,0.933333333333333,
0.966666666666667,1.),.UNSPECIFIED.)
CURVE()
GEOMETRIC_REPRESENTATION_ITEM()
RATIONAL_B_SPLINE_CURVE((1.,1.,1.,1.,1.,1.,1.,1.,1.,1.,1.,1.,1.,1.,1.,1.,
1.,1.,1.,1.,1.,1.,1.,1.,1.,1.,1.,1.,1.,1.,1.,1.,1.,1.,1.))
REPRESENTATION_ITEM('')
);
#163=(
BOUNDED_CURVE()
B_SPLINE_CURVE(5,(#94158,#94159,#94160,#94161,#94162,#94163,#94164,#94165,
#94166,#94167,#94168,#94169,#94170,#94171,#94172,#94173,#94174,#94175,#94176,
#94177,#94178,#94179,#94180,#94181,#94182,#94183,#94184,#94185,#94186,#94187,
#94188,#94189,#94190,#94191,#94192),.UNSPECIFIED.,.F.,.F.)
B_SPLINE_CURVE_WITH_KNOTS((6,1,1,1,1,1,1,1,1,1,1,1,1,1,1,1,1,1,1,1,1,1,
1,1,1,1,1,1,1,1,6),(0.,0.0333333333333333,0.0666666666666667,0.1,0.133333333333333,
0.166666666666667,0.2,0.233333333333333,0.266666666666667,0.3,0.333333333333333,
0.366666666666667,0.4,0.433333333333333,0.466666666666667,0.5,0.533333333333333,
0.566666666666667,0.6,0.633333333333333,0.666666666666667,0.7,0.733333333333333,
0.766666666666667,0.8,0.833333333333333,0.866666666666667,0.9,0.933333333333333,
0.966666666666667,1.),.UNSPECIFIED.)
CURVE()
GEOMETRIC_REPRESENTATION_ITEM()
RATIONAL_B_SPLINE_CURVE((1.,1.,1.,1.,1.,1.,1.,1.,1.,1.,1.,1.,1.,1.,1.,1.,
1.,1.,1.,1.,1.,1.,1.,1.,1.,1.,1.,1.,1.,1.,1.,1.,1.,1.,1.))
REPRESENTATION_ITEM('')
);
#164=(
BOUNDED_CURVE()
B_SPLINE_CURVE(5,(#94194,#94195,#94196,#94197,#94198,#94199,#94200,#94201,
#94202,#94203,#94204,#94205,#94206,#94207,#94208,#94209,#94210,#94211,#94212,
#94213,#94214,#94215,#94216,#94217,#94218,#94219,#94220,#94221,#94222,#94223,
#94224,#94225,#94226,#94227,#94228),.UNSPECIFIED.,.F.,.F.)
B_SPLINE_CURVE_WITH_KNOTS((6,1,1,1,1,1,1,1,1,1,1,1,1,1,1,1,1,1,1,1,1,1,
1,1,1,1,1,1,1,1,6),(-1.,-0.966666666666667,-0.933333333333333,-0.9,-0.866666666666667,
-0.833333333333333,-0.8,-0.766666666666667,-0.733333333333333,-0.7,-0.666666666666667,
-0.633333333333333,-0.6,-0.566666666666667,-0.533333333333333,-0.5,-0.466666666666667,
-0.433333333333333,-0.4,-0.366666666666667,-0.333333333333333,-0.3,-0.266666666666667,
-0.233333333333333,-0.2,-0.166666666666667,-0.133333333333333,-0.1,-0.0666666666666667,
-0.0333333333333333,0.),.UNSPECIFIED.)
CURVE()
GEOMETRIC_REPRESENTATION_ITEM()
RATIONAL_B_SPLINE_CURVE((1.,1.,1.,1.,1.,1.,1.,1.,1.,1.,1.,1.,1.,1.,1.,1.,
1.,1.,1.,1.,1.,1.,1.,1.,1.,1.,1.,1.,1.,1.,1.,1.,1.,1.,1.))
REPRESENTATION_ITEM('')
);
#165=(
BOUNDED_CURVE()
B_SPLINE_CURVE(5,(#94306,#94307,#94308,#94309,#94310,#94311,#94312,#94313,
#94314,#94315,#94316,#94317,#94318,#94319,#94320,#94321,#94322,#94323,#94324,
#94325,#94326,#94327,#94328,#94329,#94330,#94331,#94332,#94333,#94334,#94335,
#94336,#94337,#94338,#94339,#94340),.UNSPECIFIED.,.F.,.F.)
B_SPLINE_CURVE_WITH_KNOTS((6,1,1,1,1,1,1,1,1,1,1,1,1,1,1,1,1,1,1,1,1,1,
1,1,1,1,1,1,1,1,6),(0.,0.0333333333333333,0.0666666666666667,0.1,0.133333333333333,
0.166666666666667,0.2,0.233333333333333,0.266666666666667,0.3,0.333333333333333,
0.366666666666667,0.4,0.433333333333333,0.466666666666667,0.5,0.533333333333333,
0.566666666666667,0.6,0.633333333333333,0.666666666666667,0.7,0.733333333333333,
0.766666666666667,0.8,0.833333333333333,0.866666666666667,0.9,0.933333333333333,
0.966666666666667,1.),.UNSPECIFIED.)
CURVE()
GEOMETRIC_REPRESENTATION_ITEM()
RATIONAL_B_SPLINE_CURVE((1.,1.,1.,1.,1.,1.,1.,1.,1.,1.,1.,1.,1.,1.,1.,1.,
1.,1.,1.,1.,1.,1.,1.,1.,1.,1.,1.,1.,1.,1.,1.,1.,1.,1.,1.))
REPRESENTATION_ITEM('')
);
#166=(
BOUNDED_CURVE()
B_SPLINE_CURVE(5,(#94341,#94342,#94343,#94344,#94345,#94346,#94347,#94348,
#94349,#94350,#94351,#94352,#94353,#94354,#94355,#94356,#94357,#94358,#94359,
#94360,#94361,#94362,#94363,#94364,#94365,#94366,#94367,#94368,#94369,#94370,
#94371,#94372,#94373,#94374,#94375),.UNSPECIFIED.,.F.,.F.)
B_SPLINE_CURVE_WITH_KNOTS((6,1,1,1,1,1,1,1,1,1,1,1,1,1,1,1,1,1,1,1,1,1,
1,1,1,1,1,1,1,1,6),(0.,0.0333333333333333,0.0666666666666667,0.1,0.133333333333333,
0.166666666666667,0.2,0.233333333333333,0.266666666666667,0.3,0.333333333333333,
0.366666666666667,0.4,0.433333333333333,0.466666666666667,0.5,0.533333333333333,
0.566666666666667,0.6,0.633333333333333,0.666666666666667,0.7,0.733333333333333,
0.766666666666667,0.8,0.833333333333333,0.866666666666667,0.9,0.933333333333333,
0.966666666666667,1.),.UNSPECIFIED.)
CURVE()
GEOMETRIC_REPRESENTATION_ITEM()
RATIONAL_B_SPLINE_CURVE((1.,1.,1.,1.,1.,1.,1.,1.,1.,1.,1.,1.,1.,1.,1.,1.,
1.,1.,1.,1.,1.,1.,1.,1.,1.,1.,1.,1.,1.,1.,1.,1.,1.,1.,1.))
REPRESENTATION_ITEM('')
);
#167=(
BOUNDED_CURVE()
B_SPLINE_CURVE(5,(#94460,#94461,#94462,#94463,#94464,#94465,#94466,#94467,
#94468,#94469,#94470,#94471,#94472,#94473,#94474,#94475,#94476,#94477,#94478,
#94479,#94480,#94481,#94482,#94483,#94484,#94485,#94486,#94487,#94488,#94489,
#94490,#94491,#94492,#94493,#94494),.UNSPECIFIED.,.F.,.F.)
B_SPLINE_CURVE_WITH_KNOTS((6,1,1,1,1,1,1,1,1,1,1,1,1,1,1,1,1,1,1,1,1,1,
1,1,1,1,1,1,1,1,6),(0.,0.0333333333333333,0.0666666666666667,0.1,0.133333333333333,
0.166666666666667,0.2,0.233333333333333,0.266666666666667,0.3,0.333333333333333,
0.366666666666667,0.4,0.433333333333333,0.466666666666667,0.5,0.533333333333333,
0.566666666666667,0.6,0.633333333333333,0.666666666666667,0.7,0.733333333333333,
0.766666666666667,0.8,0.833333333333333,0.866666666666667,0.9,0.933333333333333,
0.966666666666667,1.),.UNSPECIFIED.)
CURVE()
GEOMETRIC_REPRESENTATION_ITEM()
RATIONAL_B_SPLINE_CURVE((1.,1.,1.,1.,1.,1.,1.,1.,1.,1.,1.,1.,1.,1.,1.,1.,
1.,1.,1.,1.,1.,1.,1.,1.,1.,1.,1.,1.,1.,1.,1.,1.,1.,1.,1.))
REPRESENTATION_ITEM('')
);
#168=(
BOUNDED_CURVE()
B_SPLINE_CURVE(5,(#94496,#94497,#94498,#94499,#94500,#94501,#94502,#94503,
#94504,#94505,#94506,#94507,#94508,#94509,#94510,#94511,#94512,#94513,#94514,
#94515,#94516,#94517,#94518,#94519,#94520,#94521,#94522,#94523,#94524,#94525,
#94526,#94527,#94528,#94529,#94530),.UNSPECIFIED.,.F.,.F.)
B_SPLINE_CURVE_WITH_KNOTS((6,1,1,1,1,1,1,1,1,1,1,1,1,1,1,1,1,1,1,1,1,1,
1,1,1,1,1,1,1,1,6),(-1.,-0.966666666666667,-0.933333333333333,-0.9,-0.866666666666667,
-0.833333333333333,-0.8,-0.766666666666667,-0.733333333333333,-0.7,-0.666666666666667,
-0.633333333333333,-0.6,-0.566666666666667,-0.533333333333333,-0.5,-0.466666666666667,
-0.433333333333333,-0.4,-0.366666666666667,-0.333333333333333,-0.3,-0.266666666666667,
-0.233333333333333,-0.2,-0.166666666666667,-0.133333333333333,-0.1,-0.0666666666666667,
-0.0333333333333333,0.),.UNSPECIFIED.)
CURVE()
GEOMETRIC_REPRESENTATION_ITEM()
RATIONAL_B_SPLINE_CURVE((1.,1.,1.,1.,1.,1.,1.,1.,1.,1.,1.,1.,1.,1.,1.,1.,
1.,1.,1.,1.,1.,1.,1.,1.,1.,1.,1.,1.,1.,1.,1.,1.,1.,1.,1.))
REPRESENTATION_ITEM('')
);
#169=(
BOUNDED_CURVE()
B_SPLINE_CURVE(5,(#94608,#94609,#94610,#94611,#94612,#94613,#94614,#94615,
#94616,#94617,#94618,#94619,#94620,#94621,#94622,#94623,#94624,#94625,#94626,
#94627,#94628,#94629,#94630,#94631,#94632,#94633,#94634,#94635,#94636,#94637,
#94638,#94639,#94640,#94641,#94642),.UNSPECIFIED.,.F.,.F.)
B_SPLINE_CURVE_WITH_KNOTS((6,1,1,1,1,1,1,1,1,1,1,1,1,1,1,1,1,1,1,1,1,1,
1,1,1,1,1,1,1,1,6),(0.,0.0333333333333333,0.0666666666666667,0.1,0.133333333333333,
0.166666666666667,0.2,0.233333333333333,0.266666666666667,0.3,0.333333333333333,
0.366666666666667,0.4,0.433333333333333,0.466666666666667,0.5,0.533333333333333,
0.566666666666667,0.6,0.633333333333333,0.666666666666667,0.7,0.733333333333333,
0.766666666666667,0.8,0.833333333333333,0.866666666666667,0.9,0.933333333333333,
0.966666666666667,1.),.UNSPECIFIED.)
CURVE()
GEOMETRIC_REPRESENTATION_ITEM()
RATIONAL_B_SPLINE_CURVE((1.,1.,1.,1.,1.,1.,1.,1.,1.,1.,1.,1.,1.,1.,1.,1.,
1.,1.,1.,1.,1.,1.,1.,1.,1.,1.,1.,1.,1.,1.,1.,1.,1.,1.,1.))
REPRESENTATION_ITEM('')
);
#170=(
BOUNDED_CURVE()
B_SPLINE_CURVE(5,(#94643,#94644,#94645,#94646,#94647,#94648,#94649,#94650,
#94651,#94652,#94653,#94654,#94655,#94656,#94657,#94658,#94659,#94660,#94661,
#94662,#94663,#94664,#94665,#94666,#94667,#94668,#94669,#94670,#94671,#94672,
#94673,#94674,#94675,#94676,#94677),.UNSPECIFIED.,.F.,.F.)
B_SPLINE_CURVE_WITH_KNOTS((6,1,1,1,1,1,1,1,1,1,1,1,1,1,1,1,1,1,1,1,1,1,
1,1,1,1,1,1,1,1,6),(0.,0.0333333333333333,0.0666666666666667,0.1,0.133333333333333,
0.166666666666667,0.2,0.233333333333333,0.266666666666667,0.3,0.333333333333333,
0.366666666666667,0.4,0.433333333333333,0.466666666666667,0.5,0.533333333333333,
0.566666666666667,0.6,0.633333333333333,0.666666666666667,0.7,0.733333333333333,
0.766666666666667,0.8,0.833333333333333,0.866666666666667,0.9,0.933333333333333,
0.966666666666667,1.),.UNSPECIFIED.)
CURVE()
GEOMETRIC_REPRESENTATION_ITEM()
RATIONAL_B_SPLINE_CURVE((1.,1.,1.,1.,1.,1.,1.,1.,1.,1.,1.,1.,1.,1.,1.,1.,
1.,1.,1.,1.,1.,1.,1.,1.,1.,1.,1.,1.,1.,1.,1.,1.,1.,1.,1.))
REPRESENTATION_ITEM('')
);
#171=(
BOUNDED_CURVE()
B_SPLINE_CURVE(5,(#94762,#94763,#94764,#94765,#94766,#94767,#94768,#94769,
#94770,#94771,#94772,#94773,#94774,#94775,#94776,#94777,#94778,#94779,#94780,
#94781,#94782,#94783,#94784,#94785,#94786,#94787,#94788,#94789,#94790,#94791,
#94792,#94793,#94794,#94795,#94796),.UNSPECIFIED.,.F.,.F.)
B_SPLINE_CURVE_WITH_KNOTS((6,1,1,1,1,1,1,1,1,1,1,1,1,1,1,1,1,1,1,1,1,1,
1,1,1,1,1,1,1,1,6),(0.,0.0333333333333333,0.0666666666666667,0.1,0.133333333333333,
0.166666666666667,0.2,0.233333333333333,0.266666666666667,0.3,0.333333333333333,
0.366666666666667,0.4,0.433333333333333,0.466666666666667,0.5,0.533333333333333,
0.566666666666667,0.6,0.633333333333333,0.666666666666667,0.7,0.733333333333333,
0.766666666666667,0.8,0.833333333333333,0.866666666666667,0.9,0.933333333333333,
0.966666666666667,1.),.UNSPECIFIED.)
CURVE()
GEOMETRIC_REPRESENTATION_ITEM()
RATIONAL_B_SPLINE_CURVE((1.,1.,1.,1.,1.,1.,1.,1.,1.,1.,1.,1.,1.,1.,1.,1.,
1.,1.,1.,1.,1.,1.,1.,1.,1.,1.,1.,1.,1.,1.,1.,1.,1.,1.,1.))
REPRESENTATION_ITEM('')
);
#172=(
BOUNDED_CURVE()
B_SPLINE_CURVE(5,(#94798,#94799,#94800,#94801,#94802,#94803,#94804,#94805,
#94806,#94807,#94808,#94809,#94810,#94811,#94812,#94813,#94814,#94815,#94816,
#94817,#94818,#94819,#94820,#94821,#94822,#94823,#94824,#94825,#94826,#94827,
#94828,#94829,#94830,#94831,#94832),.UNSPECIFIED.,.F.,.F.)
B_SPLINE_CURVE_WITH_KNOTS((6,1,1,1,1,1,1,1,1,1,1,1,1,1,1,1,1,1,1,1,1,1,
1,1,1,1,1,1,1,1,6),(-1.,-0.966666666666667,-0.933333333333333,-0.9,-0.866666666666667,
-0.833333333333333,-0.8,-0.766666666666667,-0.733333333333333,-0.7,-0.666666666666667,
-0.633333333333333,-0.6,-0.566666666666667,-0.533333333333333,-0.5,-0.466666666666667,
-0.433333333333333,-0.4,-0.366666666666667,-0.333333333333333,-0.3,-0.266666666666667,
-0.233333333333333,-0.2,-0.166666666666667,-0.133333333333333,-0.1,-0.0666666666666667,
-0.0333333333333333,0.),.UNSPECIFIED.)
CURVE()
GEOMETRIC_REPRESENTATION_ITEM()
RATIONAL_B_SPLINE_CURVE((1.,1.,1.,1.,1.,1.,1.,1.,1.,1.,1.,1.,1.,1.,1.,1.,
1.,1.,1.,1.,1.,1.,1.,1.,1.,1.,1.,1.,1.,1.,1.,1.,1.,1.,1.))
REPRESENTATION_ITEM('')
);
#173=(
BOUNDED_CURVE()
B_SPLINE_CURVE(5,(#94910,#94911,#94912,#94913,#94914,#94915,#94916,#94917,
#94918,#94919,#94920,#94921,#94922,#94923,#94924,#94925,#94926,#94927,#94928,
#94929,#94930,#94931,#94932,#94933,#94934,#94935,#94936,#94937,#94938,#94939,
#94940,#94941,#94942,#94943,#94944),.UNSPECIFIED.,.F.,.F.)
B_SPLINE_CURVE_WITH_KNOTS((6,1,1,1,1,1,1,1,1,1,1,1,1,1,1,1,1,1,1,1,1,1,
1,1,1,1,1,1,1,1,6),(0.,0.0333333333333333,0.0666666666666667,0.1,0.133333333333333,
0.166666666666667,0.2,0.233333333333333,0.266666666666667,0.3,0.333333333333333,
0.366666666666667,0.4,0.433333333333333,0.466666666666667,0.5,0.533333333333333,
0.566666666666667,0.6,0.633333333333333,0.666666666666667,0.7,0.733333333333333,
0.766666666666667,0.8,0.833333333333333,0.866666666666667,0.9,0.933333333333333,
0.966666666666667,1.),.UNSPECIFIED.)
CURVE()
GEOMETRIC_REPRESENTATION_ITEM()
RATIONAL_B_SPLINE_CURVE((1.,1.,1.,1.,1.,1.,1.,1.,1.,1.,1.,1.,1.,1.,1.,1.,
1.,1.,1.,1.,1.,1.,1.,1.,1.,1.,1.,1.,1.,1.,1.,1.,1.,1.,1.))
REPRESENTATION_ITEM('')
);
#174=(
BOUNDED_CURVE()
B_SPLINE_CURVE(5,(#94945,#94946,#94947,#94948,#94949,#94950,#94951,#94952,
#94953,#94954,#94955,#94956,#94957,#94958,#94959,#94960,#94961,#94962,#94963,
#94964,#94965,#94966,#94967,#94968,#94969,#94970,#94971,#94972,#94973,#94974,
#94975,#94976,#94977,#94978,#94979),.UNSPECIFIED.,.F.,.F.)
B_SPLINE_CURVE_WITH_KNOTS((6,1,1,1,1,1,1,1,1,1,1,1,1,1,1,1,1,1,1,1,1,1,
1,1,1,1,1,1,1,1,6),(0.,0.0333333333333333,0.0666666666666667,0.1,0.133333333333333,
0.166666666666667,0.2,0.233333333333333,0.266666666666667,0.3,0.333333333333333,
0.366666666666667,0.4,0.433333333333333,0.466666666666667,0.5,0.533333333333333,
0.566666666666667,0.6,0.633333333333333,0.666666666666667,0.7,0.733333333333333,
0.766666666666667,0.8,0.833333333333333,0.866666666666667,0.9,0.933333333333333,
0.966666666666667,1.),.UNSPECIFIED.)
CURVE()
GEOMETRIC_REPRESENTATION_ITEM()
RATIONAL_B_SPLINE_CURVE((1.,1.,1.,1.,1.,1.,1.,1.,1.,1.,1.,1.,1.,1.,1.,1.,
1.,1.,1.,1.,1.,1.,1.,1.,1.,1.,1.,1.,1.,1.,1.,1.,1.,1.,1.))
REPRESENTATION_ITEM('')
);
#175=(
BOUNDED_CURVE()
B_SPLINE_CURVE(5,(#95064,#95065,#95066,#95067,#95068,#95069,#95070,#95071,
#95072,#95073,#95074,#95075,#95076,#95077,#95078,#95079,#95080,#95081,#95082,
#95083,#95084,#95085,#95086,#95087,#95088,#95089,#95090,#95091,#95092,#95093,
#95094,#95095,#95096,#95097,#95098),.UNSPECIFIED.,.F.,.F.)
B_SPLINE_CURVE_WITH_KNOTS((6,1,1,1,1,1,1,1,1,1,1,1,1,1,1,1,1,1,1,1,1,1,
1,1,1,1,1,1,1,1,6),(0.,0.0333333333333333,0.0666666666666667,0.1,0.133333333333333,
0.166666666666667,0.2,0.233333333333333,0.266666666666667,0.3,0.333333333333333,
0.366666666666667,0.4,0.433333333333333,0.466666666666667,0.5,0.533333333333333,
0.566666666666667,0.6,0.633333333333333,0.666666666666667,0.7,0.733333333333333,
0.766666666666667,0.8,0.833333333333333,0.866666666666667,0.9,0.933333333333333,
0.966666666666667,1.),.UNSPECIFIED.)
CURVE()
GEOMETRIC_REPRESENTATION_ITEM()
RATIONAL_B_SPLINE_CURVE((1.,1.,1.,1.,1.,1.,1.,1.,1.,1.,1.,1.,1.,1.,1.,1.,
1.,1.,1.,1.,1.,1.,1.,1.,1.,1.,1.,1.,1.,1.,1.,1.,1.,1.,1.))
REPRESENTATION_ITEM('')
);
#176=(
BOUNDED_CURVE()
B_SPLINE_CURVE(5,(#95100,#95101,#95102,#95103,#95104,#95105,#95106,#95107,
#95108,#95109,#95110,#95111,#95112,#95113,#95114,#95115,#95116,#95117,#95118,
#95119,#95120,#95121,#95122,#95123,#95124,#95125,#95126,#95127,#95128,#95129,
#95130,#95131,#95132,#95133,#95134),.UNSPECIFIED.,.F.,.F.)
B_SPLINE_CURVE_WITH_KNOTS((6,1,1,1,1,1,1,1,1,1,1,1,1,1,1,1,1,1,1,1,1,1,
1,1,1,1,1,1,1,1,6),(-1.,-0.966666666666667,-0.933333333333333,-0.9,-0.866666666666667,
-0.833333333333333,-0.8,-0.766666666666667,-0.733333333333333,-0.7,-0.666666666666667,
-0.633333333333333,-0.6,-0.566666666666667,-0.533333333333333,-0.5,-0.466666666666667,
-0.433333333333333,-0.4,-0.366666666666667,-0.333333333333333,-0.3,-0.266666666666667,
-0.233333333333333,-0.2,-0.166666666666667,-0.133333333333333,-0.1,-0.0666666666666667,
-0.0333333333333333,0.),.UNSPECIFIED.)
CURVE()
GEOMETRIC_REPRESENTATION_ITEM()
RATIONAL_B_SPLINE_CURVE((1.,1.,1.,1.,1.,1.,1.,1.,1.,1.,1.,1.,1.,1.,1.,1.,
1.,1.,1.,1.,1.,1.,1.,1.,1.,1.,1.,1.,1.,1.,1.,1.,1.,1.,1.))
REPRESENTATION_ITEM('')
);
#177=(
BOUNDED_CURVE()
B_SPLINE_CURVE(5,(#95212,#95213,#95214,#95215,#95216,#95217,#95218,#95219,
#95220,#95221,#95222,#95223,#95224,#95225,#95226,#95227,#95228,#95229,#95230,
#95231,#95232,#95233,#95234,#95235,#95236,#95237,#95238,#95239,#95240,#95241,
#95242,#95243,#95244,#95245,#95246),.UNSPECIFIED.,.F.,.F.)
B_SPLINE_CURVE_WITH_KNOTS((6,1,1,1,1,1,1,1,1,1,1,1,1,1,1,1,1,1,1,1,1,1,
1,1,1,1,1,1,1,1,6),(0.,0.0333333333333333,0.0666666666666667,0.1,0.133333333333333,
0.166666666666667,0.2,0.233333333333333,0.266666666666667,0.3,0.333333333333333,
0.366666666666667,0.4,0.433333333333333,0.466666666666667,0.5,0.533333333333333,
0.566666666666667,0.6,0.633333333333333,0.666666666666667,0.7,0.733333333333333,
0.766666666666667,0.8,0.833333333333333,0.866666666666667,0.9,0.933333333333333,
0.966666666666667,1.),.UNSPECIFIED.)
CURVE()
GEOMETRIC_REPRESENTATION_ITEM()
RATIONAL_B_SPLINE_CURVE((1.,1.,1.,1.,1.,1.,1.,1.,1.,1.,1.,1.,1.,1.,1.,1.,
1.,1.,1.,1.,1.,1.,1.,1.,1.,1.,1.,1.,1.,1.,1.,1.,1.,1.,1.))
REPRESENTATION_ITEM('')
);
#178=(
BOUNDED_CURVE()
B_SPLINE_CURVE(5,(#95247,#95248,#95249,#95250,#95251,#95252,#95253,#95254,
#95255,#95256,#95257,#95258,#95259,#95260,#95261,#95262,#95263,#95264,#95265,
#95266,#95267,#95268,#95269,#95270,#95271,#95272,#95273,#95274,#95275,#95276,
#95277,#95278,#95279,#95280,#95281),.UNSPECIFIED.,.F.,.F.)
B_SPLINE_CURVE_WITH_KNOTS((6,1,1,1,1,1,1,1,1,1,1,1,1,1,1,1,1,1,1,1,1,1,
1,1,1,1,1,1,1,1,6),(0.,0.0333333333333333,0.0666666666666667,0.1,0.133333333333333,
0.166666666666667,0.2,0.233333333333333,0.266666666666667,0.3,0.333333333333333,
0.366666666666667,0.4,0.433333333333333,0.466666666666667,0.5,0.533333333333333,
0.566666666666667,0.6,0.633333333333333,0.666666666666667,0.7,0.733333333333333,
0.766666666666667,0.8,0.833333333333333,0.866666666666667,0.9,0.933333333333333,
0.966666666666667,1.),.UNSPECIFIED.)
CURVE()
GEOMETRIC_REPRESENTATION_ITEM()
RATIONAL_B_SPLINE_CURVE((1.,1.,1.,1.,1.,1.,1.,1.,1.,1.,1.,1.,1.,1.,1.,1.,
1.,1.,1.,1.,1.,1.,1.,1.,1.,1.,1.,1.,1.,1.,1.,1.,1.,1.,1.))
REPRESENTATION_ITEM('')
);
#179=(
BOUNDED_CURVE()
B_SPLINE_CURVE(5,(#95366,#95367,#95368,#95369,#95370,#95371,#95372,#95373,
#95374,#95375,#95376,#95377,#95378,#95379,#95380,#95381,#95382,#95383,#95384,
#95385,#95386,#95387,#95388,#95389,#95390,#95391,#95392,#95393,#95394,#95395,
#95396,#95397,#95398,#95399,#95400),.UNSPECIFIED.,.F.,.F.)
B_SPLINE_CURVE_WITH_KNOTS((6,1,1,1,1,1,1,1,1,1,1,1,1,1,1,1,1,1,1,1,1,1,
1,1,1,1,1,1,1,1,6),(0.,0.0333333333333333,0.0666666666666667,0.1,0.133333333333333,
0.166666666666667,0.2,0.233333333333333,0.266666666666667,0.3,0.333333333333333,
0.366666666666667,0.4,0.433333333333333,0.466666666666667,0.5,0.533333333333333,
0.566666666666667,0.6,0.633333333333333,0.666666666666667,0.7,0.733333333333333,
0.766666666666667,0.8,0.833333333333333,0.866666666666667,0.9,0.933333333333333,
0.966666666666667,1.),.UNSPECIFIED.)
CURVE()
GEOMETRIC_REPRESENTATION_ITEM()
RATIONAL_B_SPLINE_CURVE((1.,1.,1.,1.,1.,1.,1.,1.,1.,1.,1.,1.,1.,1.,1.,1.,
1.,1.,1.,1.,1.,1.,1.,1.,1.,1.,1.,1.,1.,1.,1.,1.,1.,1.,1.))
REPRESENTATION_ITEM('')
);
#180=(
BOUNDED_CURVE()
B_SPLINE_CURVE(5,(#95402,#95403,#95404,#95405,#95406,#95407,#95408,#95409,
#95410,#95411,#95412,#95413,#95414,#95415,#95416,#95417,#95418,#95419,#95420,
#95421,#95422,#95423,#95424,#95425,#95426,#95427,#95428,#95429,#95430,#95431,
#95432,#95433,#95434,#95435,#95436),.UNSPECIFIED.,.F.,.F.)
B_SPLINE_CURVE_WITH_KNOTS((6,1,1,1,1,1,1,1,1,1,1,1,1,1,1,1,1,1,1,1,1,1,
1,1,1,1,1,1,1,1,6),(-1.,-0.966666666666667,-0.933333333333333,-0.9,-0.866666666666667,
-0.833333333333333,-0.8,-0.766666666666667,-0.733333333333333,-0.7,-0.666666666666667,
-0.633333333333333,-0.6,-0.566666666666667,-0.533333333333333,-0.5,-0.466666666666667,
-0.433333333333333,-0.4,-0.366666666666667,-0.333333333333333,-0.3,-0.266666666666667,
-0.233333333333333,-0.2,-0.166666666666667,-0.133333333333333,-0.1,-0.0666666666666667,
-0.0333333333333333,0.),.UNSPECIFIED.)
CURVE()
GEOMETRIC_REPRESENTATION_ITEM()
RATIONAL_B_SPLINE_CURVE((1.,1.,1.,1.,1.,1.,1.,1.,1.,1.,1.,1.,1.,1.,1.,1.,
1.,1.,1.,1.,1.,1.,1.,1.,1.,1.,1.,1.,1.,1.,1.,1.,1.,1.,1.))
REPRESENTATION_ITEM('')
);
#181=(
BOUNDED_CURVE()
B_SPLINE_CURVE(5,(#95514,#95515,#95516,#95517,#95518,#95519,#95520,#95521,
#95522,#95523,#95524,#95525,#95526,#95527,#95528,#95529,#95530,#95531,#95532,
#95533,#95534,#95535,#95536,#95537,#95538,#95539,#95540,#95541,#95542,#95543,
#95544,#95545,#95546,#95547,#95548),.UNSPECIFIED.,.F.,.F.)
B_SPLINE_CURVE_WITH_KNOTS((6,1,1,1,1,1,1,1,1,1,1,1,1,1,1,1,1,1,1,1,1,1,
1,1,1,1,1,1,1,1,6),(0.,0.0333333333333333,0.0666666666666667,0.1,0.133333333333333,
0.166666666666667,0.2,0.233333333333333,0.266666666666667,0.3,0.333333333333333,
0.366666666666667,0.4,0.433333333333333,0.466666666666667,0.5,0.533333333333333,
0.566666666666667,0.6,0.633333333333333,0.666666666666667,0.7,0.733333333333333,
0.766666666666667,0.8,0.833333333333333,0.866666666666667,0.9,0.933333333333333,
0.966666666666667,1.),.UNSPECIFIED.)
CURVE()
GEOMETRIC_REPRESENTATION_ITEM()
RATIONAL_B_SPLINE_CURVE((1.,1.,1.,1.,1.,1.,1.,1.,1.,1.,1.,1.,1.,1.,1.,1.,
1.,1.,1.,1.,1.,1.,1.,1.,1.,1.,1.,1.,1.,1.,1.,1.,1.,1.,1.))
REPRESENTATION_ITEM('')
);
#182=(
BOUNDED_CURVE()
B_SPLINE_CURVE(5,(#95549,#95550,#95551,#95552,#95553,#95554,#95555,#95556,
#95557,#95558,#95559,#95560,#95561,#95562,#95563,#95564,#95565,#95566,#95567,
#95568,#95569,#95570,#95571,#95572,#95573,#95574,#95575,#95576,#95577,#95578,
#95579,#95580,#95581,#95582,#95583),.UNSPECIFIED.,.F.,.F.)
B_SPLINE_CURVE_WITH_KNOTS((6,1,1,1,1,1,1,1,1,1,1,1,1,1,1,1,1,1,1,1,1,1,
1,1,1,1,1,1,1,1,6),(0.,0.0333333333333333,0.0666666666666667,0.1,0.133333333333333,
0.166666666666667,0.2,0.233333333333333,0.266666666666667,0.3,0.333333333333333,
0.366666666666667,0.4,0.433333333333333,0.466666666666667,0.5,0.533333333333333,
0.566666666666667,0.6,0.633333333333333,0.666666666666667,0.7,0.733333333333333,
0.766666666666667,0.8,0.833333333333333,0.866666666666667,0.9,0.933333333333333,
0.966666666666667,1.),.UNSPECIFIED.)
CURVE()
GEOMETRIC_REPRESENTATION_ITEM()
RATIONAL_B_SPLINE_CURVE((1.,1.,1.,1.,1.,1.,1.,1.,1.,1.,1.,1.,1.,1.,1.,1.,
1.,1.,1.,1.,1.,1.,1.,1.,1.,1.,1.,1.,1.,1.,1.,1.,1.,1.,1.))
REPRESENTATION_ITEM('')
);
#183=(
BOUNDED_CURVE()
B_SPLINE_CURVE(5,(#95668,#95669,#95670,#95671,#95672,#95673,#95674,#95675,
#95676,#95677,#95678,#95679,#95680,#95681,#95682,#95683,#95684,#95685,#95686,
#95687,#95688,#95689,#95690,#95691,#95692,#95693,#95694,#95695,#95696,#95697,
#95698,#95699,#95700,#95701,#95702),.UNSPECIFIED.,.F.,.F.)
B_SPLINE_CURVE_WITH_KNOTS((6,1,1,1,1,1,1,1,1,1,1,1,1,1,1,1,1,1,1,1,1,1,
1,1,1,1,1,1,1,1,6),(0.,0.0333333333333333,0.0666666666666667,0.1,0.133333333333333,
0.166666666666667,0.2,0.233333333333333,0.266666666666667,0.3,0.333333333333333,
0.366666666666667,0.4,0.433333333333333,0.466666666666667,0.5,0.533333333333333,
0.566666666666667,0.6,0.633333333333333,0.666666666666667,0.7,0.733333333333333,
0.766666666666667,0.8,0.833333333333333,0.866666666666667,0.9,0.933333333333333,
0.966666666666667,1.),.UNSPECIFIED.)
CURVE()
GEOMETRIC_REPRESENTATION_ITEM()
RATIONAL_B_SPLINE_CURVE((1.,1.,1.,1.,1.,1.,1.,1.,1.,1.,1.,1.,1.,1.,1.,1.,
1.,1.,1.,1.,1.,1.,1.,1.,1.,1.,1.,1.,1.,1.,1.,1.,1.,1.,1.))
REPRESENTATION_ITEM('')
);
#184=(
BOUNDED_CURVE()
B_SPLINE_CURVE(5,(#95704,#95705,#95706,#95707,#95708,#95709,#95710,#95711,
#95712,#95713,#95714,#95715,#95716,#95717,#95718,#95719,#95720,#95721,#95722,
#95723,#95724,#95725,#95726,#95727,#95728,#95729,#95730,#95731,#95732,#95733,
#95734,#95735,#95736,#95737,#95738),.UNSPECIFIED.,.F.,.F.)
B_SPLINE_CURVE_WITH_KNOTS((6,1,1,1,1,1,1,1,1,1,1,1,1,1,1,1,1,1,1,1,1,1,
1,1,1,1,1,1,1,1,6),(-1.,-0.966666666666667,-0.933333333333333,-0.9,-0.866666666666667,
-0.833333333333333,-0.8,-0.766666666666667,-0.733333333333333,-0.7,-0.666666666666667,
-0.633333333333333,-0.6,-0.566666666666667,-0.533333333333333,-0.5,-0.466666666666667,
-0.433333333333333,-0.4,-0.366666666666667,-0.333333333333333,-0.3,-0.266666666666667,
-0.233333333333333,-0.2,-0.166666666666667,-0.133333333333333,-0.1,-0.0666666666666667,
-0.0333333333333333,0.),.UNSPECIFIED.)
CURVE()
GEOMETRIC_REPRESENTATION_ITEM()
RATIONAL_B_SPLINE_CURVE((1.,1.,1.,1.,1.,1.,1.,1.,1.,1.,1.,1.,1.,1.,1.,1.,
1.,1.,1.,1.,1.,1.,1.,1.,1.,1.,1.,1.,1.,1.,1.,1.,1.,1.,1.))
REPRESENTATION_ITEM('')
);
#185=(
BOUNDED_CURVE()
B_SPLINE_CURVE(5,(#95816,#95817,#95818,#95819,#95820,#95821,#95822,#95823,
#95824,#95825,#95826,#95827,#95828,#95829,#95830,#95831,#95832,#95833,#95834,
#95835,#95836,#95837,#95838,#95839,#95840,#95841,#95842,#95843,#95844,#95845,
#95846,#95847,#95848,#95849,#95850),.UNSPECIFIED.,.F.,.F.)
B_SPLINE_CURVE_WITH_KNOTS((6,1,1,1,1,1,1,1,1,1,1,1,1,1,1,1,1,1,1,1,1,1,
1,1,1,1,1,1,1,1,6),(0.,0.0333333333333333,0.0666666666666667,0.1,0.133333333333333,
0.166666666666667,0.2,0.233333333333333,0.266666666666667,0.3,0.333333333333333,
0.366666666666667,0.4,0.433333333333333,0.466666666666667,0.5,0.533333333333333,
0.566666666666667,0.6,0.633333333333333,0.666666666666667,0.7,0.733333333333333,
0.766666666666667,0.8,0.833333333333333,0.866666666666667,0.9,0.933333333333333,
0.966666666666667,1.),.UNSPECIFIED.)
CURVE()
GEOMETRIC_REPRESENTATION_ITEM()
RATIONAL_B_SPLINE_CURVE((1.,1.,1.,1.,1.,1.,1.,1.,1.,1.,1.,1.,1.,1.,1.,1.,
1.,1.,1.,1.,1.,1.,1.,1.,1.,1.,1.,1.,1.,1.,1.,1.,1.,1.,1.))
REPRESENTATION_ITEM('')
);
#186=(
BOUNDED_CURVE()
B_SPLINE_CURVE(5,(#95851,#95852,#95853,#95854,#95855,#95856,#95857,#95858,
#95859,#95860,#95861,#95862,#95863,#95864,#95865,#95866,#95867,#95868,#95869,
#95870,#95871,#95872,#95873,#95874,#95875,#95876,#95877,#95878,#95879,#95880,
#95881,#95882,#95883,#95884,#95885),.UNSPECIFIED.,.F.,.F.)
B_SPLINE_CURVE_WITH_KNOTS((6,1,1,1,1,1,1,1,1,1,1,1,1,1,1,1,1,1,1,1,1,1,
1,1,1,1,1,1,1,1,6),(0.,0.0333333333333333,0.0666666666666667,0.1,0.133333333333333,
0.166666666666667,0.2,0.233333333333333,0.266666666666667,0.3,0.333333333333333,
0.366666666666667,0.4,0.433333333333333,0.466666666666667,0.5,0.533333333333333,
0.566666666666667,0.6,0.633333333333333,0.666666666666667,0.7,0.733333333333333,
0.766666666666667,0.8,0.833333333333333,0.866666666666667,0.9,0.933333333333333,
0.966666666666667,1.),.UNSPECIFIED.)
CURVE()
GEOMETRIC_REPRESENTATION_ITEM()
RATIONAL_B_SPLINE_CURVE((1.,1.,1.,1.,1.,1.,1.,1.,1.,1.,1.,1.,1.,1.,1.,1.,
1.,1.,1.,1.,1.,1.,1.,1.,1.,1.,1.,1.,1.,1.,1.,1.,1.,1.,1.))
REPRESENTATION_ITEM('')
);
#187=(
BOUNDED_CURVE()
B_SPLINE_CURVE(5,(#95970,#95971,#95972,#95973,#95974,#95975,#95976,#95977,
#95978,#95979,#95980,#95981,#95982,#95983,#95984,#95985,#95986,#95987,#95988,
#95989,#95990,#95991,#95992,#95993,#95994,#95995,#95996,#95997,#95998,#95999,
#96000,#96001,#96002,#96003,#96004),.UNSPECIFIED.,.F.,.F.)
B_SPLINE_CURVE_WITH_KNOTS((6,1,1,1,1,1,1,1,1,1,1,1,1,1,1,1,1,1,1,1,1,1,
1,1,1,1,1,1,1,1,6),(0.,0.0333333333333333,0.0666666666666667,0.1,0.133333333333333,
0.166666666666667,0.2,0.233333333333333,0.266666666666667,0.3,0.333333333333333,
0.366666666666667,0.4,0.433333333333333,0.466666666666667,0.5,0.533333333333333,
0.566666666666667,0.6,0.633333333333333,0.666666666666667,0.7,0.733333333333333,
0.766666666666667,0.8,0.833333333333333,0.866666666666667,0.9,0.933333333333333,
0.966666666666667,1.),.UNSPECIFIED.)
CURVE()
GEOMETRIC_REPRESENTATION_ITEM()
RATIONAL_B_SPLINE_CURVE((1.,1.,1.,1.,1.,1.,1.,1.,1.,1.,1.,1.,1.,1.,1.,1.,
1.,1.,1.,1.,1.,1.,1.,1.,1.,1.,1.,1.,1.,1.,1.,1.,1.,1.,1.))
REPRESENTATION_ITEM('')
);
#188=(
BOUNDED_CURVE()
B_SPLINE_CURVE(5,(#96006,#96007,#96008,#96009,#96010,#96011,#96012,#96013,
#96014,#96015,#96016,#96017,#96018,#96019,#96020,#96021,#96022,#96023,#96024,
#96025,#96026,#96027,#96028,#96029,#96030,#96031,#96032,#96033,#96034,#96035,
#96036,#96037,#96038,#96039,#96040),.UNSPECIFIED.,.F.,.F.)
B_SPLINE_CURVE_WITH_KNOTS((6,1,1,1,1,1,1,1,1,1,1,1,1,1,1,1,1,1,1,1,1,1,
1,1,1,1,1,1,1,1,6),(-1.,-0.966666666666667,-0.933333333333333,-0.9,-0.866666666666667,
-0.833333333333333,-0.8,-0.766666666666667,-0.733333333333333,-0.7,-0.666666666666667,
-0.633333333333333,-0.6,-0.566666666666667,-0.533333333333333,-0.5,-0.466666666666667,
-0.433333333333333,-0.4,-0.366666666666667,-0.333333333333333,-0.3,-0.266666666666667,
-0.233333333333333,-0.2,-0.166666666666667,-0.133333333333333,-0.1,-0.0666666666666667,
-0.0333333333333333,0.),.UNSPECIFIED.)
CURVE()
GEOMETRIC_REPRESENTATION_ITEM()
RATIONAL_B_SPLINE_CURVE((1.,1.,1.,1.,1.,1.,1.,1.,1.,1.,1.,1.,1.,1.,1.,1.,
1.,1.,1.,1.,1.,1.,1.,1.,1.,1.,1.,1.,1.,1.,1.,1.,1.,1.,1.))
REPRESENTATION_ITEM('')
);
#189=(
BOUNDED_CURVE()
B_SPLINE_CURVE(5,(#96118,#96119,#96120,#96121,#96122,#96123,#96124,#96125,
#96126,#96127,#96128,#96129,#96130,#96131,#96132,#96133,#96134,#96135,#96136,
#96137,#96138,#96139,#96140,#96141,#96142,#96143,#96144,#96145,#96146,#96147,
#96148,#96149,#96150,#96151,#96152),.UNSPECIFIED.,.F.,.F.)
B_SPLINE_CURVE_WITH_KNOTS((6,1,1,1,1,1,1,1,1,1,1,1,1,1,1,1,1,1,1,1,1,1,
1,1,1,1,1,1,1,1,6),(0.,0.0333333333333333,0.0666666666666667,0.1,0.133333333333333,
0.166666666666667,0.2,0.233333333333333,0.266666666666667,0.3,0.333333333333333,
0.366666666666667,0.4,0.433333333333333,0.466666666666667,0.5,0.533333333333333,
0.566666666666667,0.6,0.633333333333333,0.666666666666667,0.7,0.733333333333333,
0.766666666666667,0.8,0.833333333333333,0.866666666666667,0.9,0.933333333333333,
0.966666666666667,1.),.UNSPECIFIED.)
CURVE()
GEOMETRIC_REPRESENTATION_ITEM()
RATIONAL_B_SPLINE_CURVE((1.,1.,1.,1.,1.,1.,1.,1.,1.,1.,1.,1.,1.,1.,1.,1.,
1.,1.,1.,1.,1.,1.,1.,1.,1.,1.,1.,1.,1.,1.,1.,1.,1.,1.,1.))
REPRESENTATION_ITEM('')
);
#190=(
BOUNDED_CURVE()
B_SPLINE_CURVE(5,(#96153,#96154,#96155,#96156,#96157,#96158,#96159,#96160,
#96161,#96162,#96163,#96164,#96165,#96166,#96167,#96168,#96169,#96170,#96171,
#96172,#96173,#96174,#96175,#96176,#96177,#96178,#96179,#96180,#96181,#96182,
#96183,#96184,#96185,#96186,#96187),.UNSPECIFIED.,.F.,.F.)
B_SPLINE_CURVE_WITH_KNOTS((6,1,1,1,1,1,1,1,1,1,1,1,1,1,1,1,1,1,1,1,1,1,
1,1,1,1,1,1,1,1,6),(0.,0.0333333333333333,0.0666666666666667,0.1,0.133333333333333,
0.166666666666667,0.2,0.233333333333333,0.266666666666667,0.3,0.333333333333333,
0.366666666666667,0.4,0.433333333333333,0.466666666666667,0.5,0.533333333333333,
0.566666666666667,0.6,0.633333333333333,0.666666666666667,0.7,0.733333333333333,
0.766666666666667,0.8,0.833333333333333,0.866666666666667,0.9,0.933333333333333,
0.966666666666667,1.),.UNSPECIFIED.)
CURVE()
GEOMETRIC_REPRESENTATION_ITEM()
RATIONAL_B_SPLINE_CURVE((1.,1.,1.,1.,1.,1.,1.,1.,1.,1.,1.,1.,1.,1.,1.,1.,
1.,1.,1.,1.,1.,1.,1.,1.,1.,1.,1.,1.,1.,1.,1.,1.,1.,1.,1.))
REPRESENTATION_ITEM('')
);
#191=(
BOUNDED_CURVE()
B_SPLINE_CURVE(5,(#96272,#96273,#96274,#96275,#96276,#96277,#96278,#96279,
#96280,#96281,#96282,#96283,#96284,#96285,#96286,#96287,#96288,#96289,#96290,
#96291,#96292,#96293,#96294,#96295,#96296,#96297,#96298,#96299,#96300,#96301,
#96302,#96303,#96304,#96305,#96306),.UNSPECIFIED.,.F.,.F.)
B_SPLINE_CURVE_WITH_KNOTS((6,1,1,1,1,1,1,1,1,1,1,1,1,1,1,1,1,1,1,1,1,1,
1,1,1,1,1,1,1,1,6),(0.,0.0333333333333333,0.0666666666666667,0.1,0.133333333333333,
0.166666666666667,0.2,0.233333333333333,0.266666666666667,0.3,0.333333333333333,
0.366666666666667,0.4,0.433333333333333,0.466666666666667,0.5,0.533333333333333,
0.566666666666667,0.6,0.633333333333333,0.666666666666667,0.7,0.733333333333333,
0.766666666666667,0.8,0.833333333333333,0.866666666666667,0.9,0.933333333333333,
0.966666666666667,1.),.UNSPECIFIED.)
CURVE()
GEOMETRIC_REPRESENTATION_ITEM()
RATIONAL_B_SPLINE_CURVE((1.,1.,1.,1.,1.,1.,1.,1.,1.,1.,1.,1.,1.,1.,1.,1.,
1.,1.,1.,1.,1.,1.,1.,1.,1.,1.,1.,1.,1.,1.,1.,1.,1.,1.,1.))
REPRESENTATION_ITEM('')
);
#192=(
BOUNDED_CURVE()
B_SPLINE_CURVE(5,(#96308,#96309,#96310,#96311,#96312,#96313,#96314,#96315,
#96316,#96317,#96318,#96319,#96320,#96321,#96322,#96323,#96324,#96325,#96326,
#96327,#96328,#96329,#96330,#96331,#96332,#96333,#96334,#96335,#96336,#96337,
#96338,#96339,#96340,#96341,#96342),.UNSPECIFIED.,.F.,.F.)
B_SPLINE_CURVE_WITH_KNOTS((6,1,1,1,1,1,1,1,1,1,1,1,1,1,1,1,1,1,1,1,1,1,
1,1,1,1,1,1,1,1,6),(-1.,-0.966666666666667,-0.933333333333333,-0.9,-0.866666666666667,
-0.833333333333333,-0.8,-0.766666666666667,-0.733333333333333,-0.7,-0.666666666666667,
-0.633333333333333,-0.6,-0.566666666666667,-0.533333333333333,-0.5,-0.466666666666667,
-0.433333333333333,-0.4,-0.366666666666667,-0.333333333333333,-0.3,-0.266666666666667,
-0.233333333333333,-0.2,-0.166666666666667,-0.133333333333333,-0.1,-0.0666666666666667,
-0.0333333333333333,0.),.UNSPECIFIED.)
CURVE()
GEOMETRIC_REPRESENTATION_ITEM()
RATIONAL_B_SPLINE_CURVE((1.,1.,1.,1.,1.,1.,1.,1.,1.,1.,1.,1.,1.,1.,1.,1.,
1.,1.,1.,1.,1.,1.,1.,1.,1.,1.,1.,1.,1.,1.,1.,1.,1.,1.,1.))
REPRESENTATION_ITEM('')
);
#193=(
BOUNDED_CURVE()
B_SPLINE_CURVE(5,(#96420,#96421,#96422,#96423,#96424,#96425,#96426,#96427,
#96428,#96429,#96430,#96431,#96432,#96433,#96434,#96435,#96436,#96437,#96438,
#96439,#96440,#96441,#96442,#96443,#96444,#96445,#96446,#96447,#96448,#96449,
#96450,#96451,#96452,#96453,#96454),.UNSPECIFIED.,.F.,.F.)
B_SPLINE_CURVE_WITH_KNOTS((6,1,1,1,1,1,1,1,1,1,1,1,1,1,1,1,1,1,1,1,1,1,
1,1,1,1,1,1,1,1,6),(0.,0.0333333333333333,0.0666666666666667,0.1,0.133333333333333,
0.166666666666667,0.2,0.233333333333333,0.266666666666667,0.3,0.333333333333333,
0.366666666666667,0.4,0.433333333333333,0.466666666666667,0.5,0.533333333333333,
0.566666666666667,0.6,0.633333333333333,0.666666666666667,0.7,0.733333333333333,
0.766666666666667,0.8,0.833333333333333,0.866666666666667,0.9,0.933333333333333,
0.966666666666667,1.),.UNSPECIFIED.)
CURVE()
GEOMETRIC_REPRESENTATION_ITEM()
RATIONAL_B_SPLINE_CURVE((1.,1.,1.,1.,1.,1.,1.,1.,1.,1.,1.,1.,1.,1.,1.,1.,
1.,1.,1.,1.,1.,1.,1.,1.,1.,1.,1.,1.,1.,1.,1.,1.,1.,1.,1.))
REPRESENTATION_ITEM('')
);
#194=(
BOUNDED_CURVE()
B_SPLINE_CURVE(5,(#96455,#96456,#96457,#96458,#96459,#96460,#96461,#96462,
#96463,#96464,#96465,#96466,#96467,#96468,#96469,#96470,#96471,#96472,#96473,
#96474,#96475,#96476,#96477,#96478,#96479,#96480,#96481,#96482,#96483,#96484,
#96485,#96486,#96487,#96488,#96489),.UNSPECIFIED.,.F.,.F.)
B_SPLINE_CURVE_WITH_KNOTS((6,1,1,1,1,1,1,1,1,1,1,1,1,1,1,1,1,1,1,1,1,1,
1,1,1,1,1,1,1,1,6),(0.,0.0333333333333333,0.0666666666666667,0.1,0.133333333333333,
0.166666666666667,0.2,0.233333333333333,0.266666666666667,0.3,0.333333333333333,
0.366666666666667,0.4,0.433333333333333,0.466666666666667,0.5,0.533333333333333,
0.566666666666667,0.6,0.633333333333333,0.666666666666667,0.7,0.733333333333333,
0.766666666666667,0.8,0.833333333333333,0.866666666666667,0.9,0.933333333333333,
0.966666666666667,1.),.UNSPECIFIED.)
CURVE()
GEOMETRIC_REPRESENTATION_ITEM()
RATIONAL_B_SPLINE_CURVE((1.,1.,1.,1.,1.,1.,1.,1.,1.,1.,1.,1.,1.,1.,1.,1.,
1.,1.,1.,1.,1.,1.,1.,1.,1.,1.,1.,1.,1.,1.,1.,1.,1.,1.,1.))
REPRESENTATION_ITEM('')
);
#195=(
BOUNDED_CURVE()
B_SPLINE_CURVE(5,(#96574,#96575,#96576,#96577,#96578,#96579,#96580,#96581,
#96582,#96583,#96584,#96585,#96586,#96587,#96588,#96589,#96590,#96591,#96592,
#96593,#96594,#96595,#96596,#96597,#96598,#96599,#96600,#96601,#96602,#96603,
#96604,#96605,#96606,#96607,#96608),.UNSPECIFIED.,.F.,.F.)
B_SPLINE_CURVE_WITH_KNOTS((6,1,1,1,1,1,1,1,1,1,1,1,1,1,1,1,1,1,1,1,1,1,
1,1,1,1,1,1,1,1,6),(0.,0.0333333333333333,0.0666666666666667,0.1,0.133333333333333,
0.166666666666667,0.2,0.233333333333333,0.266666666666667,0.3,0.333333333333333,
0.366666666666667,0.4,0.433333333333333,0.466666666666667,0.5,0.533333333333333,
0.566666666666667,0.6,0.633333333333333,0.666666666666667,0.7,0.733333333333333,
0.766666666666667,0.8,0.833333333333333,0.866666666666667,0.9,0.933333333333333,
0.966666666666667,1.),.UNSPECIFIED.)
CURVE()
GEOMETRIC_REPRESENTATION_ITEM()
RATIONAL_B_SPLINE_CURVE((1.,1.,1.,1.,1.,1.,1.,1.,1.,1.,1.,1.,1.,1.,1.,1.,
1.,1.,1.,1.,1.,1.,1.,1.,1.,1.,1.,1.,1.,1.,1.,1.,1.,1.,1.))
REPRESENTATION_ITEM('')
);
#196=(
BOUNDED_CURVE()
B_SPLINE_CURVE(5,(#96610,#96611,#96612,#96613,#96614,#96615,#96616,#96617,
#96618,#96619,#96620,#96621,#96622,#96623,#96624,#96625,#96626,#96627,#96628,
#96629,#96630,#96631,#96632,#96633,#96634,#96635,#96636,#96637,#96638,#96639,
#96640,#96641,#96642,#96643,#96644),.UNSPECIFIED.,.F.,.F.)
B_SPLINE_CURVE_WITH_KNOTS((6,1,1,1,1,1,1,1,1,1,1,1,1,1,1,1,1,1,1,1,1,1,
1,1,1,1,1,1,1,1,6),(-1.,-0.966666666666667,-0.933333333333333,-0.9,-0.866666666666667,
-0.833333333333333,-0.8,-0.766666666666667,-0.733333333333333,-0.7,-0.666666666666667,
-0.633333333333333,-0.6,-0.566666666666667,-0.533333333333333,-0.5,-0.466666666666667,
-0.433333333333333,-0.4,-0.366666666666667,-0.333333333333333,-0.3,-0.266666666666667,
-0.233333333333333,-0.2,-0.166666666666667,-0.133333333333333,-0.1,-0.0666666666666667,
-0.0333333333333333,0.),.UNSPECIFIED.)
CURVE()
GEOMETRIC_REPRESENTATION_ITEM()
RATIONAL_B_SPLINE_CURVE((1.,1.,1.,1.,1.,1.,1.,1.,1.,1.,1.,1.,1.,1.,1.,1.,
1.,1.,1.,1.,1.,1.,1.,1.,1.,1.,1.,1.,1.,1.,1.,1.,1.,1.,1.))
REPRESENTATION_ITEM('')
);
#197=(
BOUNDED_CURVE()
B_SPLINE_CURVE(5,(#96722,#96723,#96724,#96725,#96726,#96727,#96728,#96729,
#96730,#96731,#96732,#96733,#96734,#96735,#96736,#96737,#96738,#96739,#96740,
#96741,#96742,#96743,#96744,#96745,#96746,#96747,#96748,#96749,#96750,#96751,
#96752,#96753,#96754,#96755,#96756),.UNSPECIFIED.,.F.,.F.)
B_SPLINE_CURVE_WITH_KNOTS((6,1,1,1,1,1,1,1,1,1,1,1,1,1,1,1,1,1,1,1,1,1,
1,1,1,1,1,1,1,1,6),(0.,0.0333333333333333,0.0666666666666667,0.1,0.133333333333333,
0.166666666666667,0.2,0.233333333333333,0.266666666666667,0.3,0.333333333333333,
0.366666666666667,0.4,0.433333333333333,0.466666666666667,0.5,0.533333333333333,
0.566666666666667,0.6,0.633333333333333,0.666666666666667,0.7,0.733333333333333,
0.766666666666667,0.8,0.833333333333333,0.866666666666667,0.9,0.933333333333333,
0.966666666666667,1.),.UNSPECIFIED.)
CURVE()
GEOMETRIC_REPRESENTATION_ITEM()
RATIONAL_B_SPLINE_CURVE((1.,1.,1.,1.,1.,1.,1.,1.,1.,1.,1.,1.,1.,1.,1.,1.,
1.,1.,1.,1.,1.,1.,1.,1.,1.,1.,1.,1.,1.,1.,1.,1.,1.,1.,1.))
REPRESENTATION_ITEM('')
);
#198=(
BOUNDED_CURVE()
B_SPLINE_CURVE(5,(#96757,#96758,#96759,#96760,#96761,#96762,#96763,#96764,
#96765,#96766,#96767,#96768,#96769,#96770,#96771,#96772,#96773,#96774,#96775,
#96776,#96777,#96778,#96779,#96780,#96781,#96782,#96783,#96784,#96785,#96786,
#96787,#96788,#96789,#96790,#96791),.UNSPECIFIED.,.F.,.F.)
B_SPLINE_CURVE_WITH_KNOTS((6,1,1,1,1,1,1,1,1,1,1,1,1,1,1,1,1,1,1,1,1,1,
1,1,1,1,1,1,1,1,6),(0.,0.0333333333333333,0.0666666666666667,0.1,0.133333333333333,
0.166666666666667,0.2,0.233333333333333,0.266666666666667,0.3,0.333333333333333,
0.366666666666667,0.4,0.433333333333333,0.466666666666667,0.5,0.533333333333333,
0.566666666666667,0.6,0.633333333333333,0.666666666666667,0.7,0.733333333333333,
0.766666666666667,0.8,0.833333333333333,0.866666666666667,0.9,0.933333333333333,
0.966666666666667,1.),.UNSPECIFIED.)
CURVE()
GEOMETRIC_REPRESENTATION_ITEM()
RATIONAL_B_SPLINE_CURVE((1.,1.,1.,1.,1.,1.,1.,1.,1.,1.,1.,1.,1.,1.,1.,1.,
1.,1.,1.,1.,1.,1.,1.,1.,1.,1.,1.,1.,1.,1.,1.,1.,1.,1.,1.))
REPRESENTATION_ITEM('')
);
#199=(
BOUNDED_CURVE()
B_SPLINE_CURVE(5,(#96876,#96877,#96878,#96879,#96880,#96881,#96882,#96883,
#96884,#96885,#96886,#96887,#96888,#96889,#96890,#96891,#96892,#96893,#96894,
#96895,#96896,#96897,#96898,#96899,#96900,#96901,#96902,#96903,#96904,#96905,
#96906,#96907,#96908,#96909,#96910),.UNSPECIFIED.,.F.,.F.)
B_SPLINE_CURVE_WITH_KNOTS((6,1,1,1,1,1,1,1,1,1,1,1,1,1,1,1,1,1,1,1,1,1,
1,1,1,1,1,1,1,1,6),(0.,0.0333333333333333,0.0666666666666667,0.1,0.133333333333333,
0.166666666666667,0.2,0.233333333333333,0.266666666666667,0.3,0.333333333333333,
0.366666666666667,0.4,0.433333333333333,0.466666666666667,0.5,0.533333333333333,
0.566666666666667,0.6,0.633333333333333,0.666666666666667,0.7,0.733333333333333,
0.766666666666667,0.8,0.833333333333333,0.866666666666667,0.9,0.933333333333333,
0.966666666666667,1.),.UNSPECIFIED.)
CURVE()
GEOMETRIC_REPRESENTATION_ITEM()
RATIONAL_B_SPLINE_CURVE((1.,1.,1.,1.,1.,1.,1.,1.,1.,1.,1.,1.,1.,1.,1.,1.,
1.,1.,1.,1.,1.,1.,1.,1.,1.,1.,1.,1.,1.,1.,1.,1.,1.,1.,1.))
REPRESENTATION_ITEM('')
);
#200=(
BOUNDED_CURVE()
B_SPLINE_CURVE(5,(#96912,#96913,#96914,#96915,#96916,#96917,#96918,#96919,
#96920,#96921,#96922,#96923,#96924,#96925,#96926,#96927,#96928,#96929,#96930,
#96931,#96932,#96933,#96934,#96935,#96936,#96937,#96938,#96939,#96940,#96941,
#96942,#96943,#96944,#96945,#96946),.UNSPECIFIED.,.F.,.F.)
B_SPLINE_CURVE_WITH_KNOTS((6,1,1,1,1,1,1,1,1,1,1,1,1,1,1,1,1,1,1,1,1,1,
1,1,1,1,1,1,1,1,6),(-1.,-0.966666666666667,-0.933333333333333,-0.9,-0.866666666666667,
-0.833333333333333,-0.8,-0.766666666666667,-0.733333333333333,-0.7,-0.666666666666667,
-0.633333333333333,-0.6,-0.566666666666667,-0.533333333333333,-0.5,-0.466666666666667,
-0.433333333333333,-0.4,-0.366666666666667,-0.333333333333333,-0.3,-0.266666666666667,
-0.233333333333333,-0.2,-0.166666666666667,-0.133333333333333,-0.1,-0.0666666666666667,
-0.0333333333333333,0.),.UNSPECIFIED.)
CURVE()
GEOMETRIC_REPRESENTATION_ITEM()
RATIONAL_B_SPLINE_CURVE((1.,1.,1.,1.,1.,1.,1.,1.,1.,1.,1.,1.,1.,1.,1.,1.,
1.,1.,1.,1.,1.,1.,1.,1.,1.,1.,1.,1.,1.,1.,1.,1.,1.,1.,1.))
REPRESENTATION_ITEM('')
);
#201=(
BOUNDED_CURVE()
B_SPLINE_CURVE(5,(#97024,#97025,#97026,#97027,#97028,#97029,#97030,#97031,
#97032,#97033,#97034,#97035,#97036,#97037,#97038,#97039,#97040,#97041,#97042,
#97043,#97044,#97045,#97046,#97047,#97048,#97049,#97050,#97051,#97052,#97053,
#97054,#97055,#97056,#97057,#97058),.UNSPECIFIED.,.F.,.F.)
B_SPLINE_CURVE_WITH_KNOTS((6,1,1,1,1,1,1,1,1,1,1,1,1,1,1,1,1,1,1,1,1,1,
1,1,1,1,1,1,1,1,6),(0.,0.0333333333333333,0.0666666666666667,0.1,0.133333333333333,
0.166666666666667,0.2,0.233333333333333,0.266666666666667,0.3,0.333333333333333,
0.366666666666667,0.4,0.433333333333333,0.466666666666667,0.5,0.533333333333333,
0.566666666666667,0.6,0.633333333333333,0.666666666666667,0.7,0.733333333333333,
0.766666666666667,0.8,0.833333333333333,0.866666666666667,0.9,0.933333333333333,
0.966666666666667,1.),.UNSPECIFIED.)
CURVE()
GEOMETRIC_REPRESENTATION_ITEM()
RATIONAL_B_SPLINE_CURVE((1.,1.,1.,1.,1.,1.,1.,1.,1.,1.,1.,1.,1.,1.,1.,1.,
1.,1.,1.,1.,1.,1.,1.,1.,1.,1.,1.,1.,1.,1.,1.,1.,1.,1.,1.))
REPRESENTATION_ITEM('')
);
#202=(
BOUNDED_CURVE()
B_SPLINE_CURVE(5,(#97059,#97060,#97061,#97062,#97063,#97064,#97065,#97066,
#97067,#97068,#97069,#97070,#97071,#97072,#97073,#97074,#97075,#97076,#97077,
#97078,#97079,#97080,#97081,#97082,#97083,#97084,#97085,#97086,#97087,#97088,
#97089,#97090,#97091,#97092,#97093),.UNSPECIFIED.,.F.,.F.)
B_SPLINE_CURVE_WITH_KNOTS((6,1,1,1,1,1,1,1,1,1,1,1,1,1,1,1,1,1,1,1,1,1,
1,1,1,1,1,1,1,1,6),(0.,0.0333333333333333,0.0666666666666667,0.1,0.133333333333333,
0.166666666666667,0.2,0.233333333333333,0.266666666666667,0.3,0.333333333333333,
0.366666666666667,0.4,0.433333333333333,0.466666666666667,0.5,0.533333333333333,
0.566666666666667,0.6,0.633333333333333,0.666666666666667,0.7,0.733333333333333,
0.766666666666667,0.8,0.833333333333333,0.866666666666667,0.9,0.933333333333333,
0.966666666666667,1.),.UNSPECIFIED.)
CURVE()
GEOMETRIC_REPRESENTATION_ITEM()
RATIONAL_B_SPLINE_CURVE((1.,1.,1.,1.,1.,1.,1.,1.,1.,1.,1.,1.,1.,1.,1.,1.,
1.,1.,1.,1.,1.,1.,1.,1.,1.,1.,1.,1.,1.,1.,1.,1.,1.,1.,1.))
REPRESENTATION_ITEM('')
);
#203=(
BOUNDED_CURVE()
B_SPLINE_CURVE(5,(#97178,#97179,#97180,#97181,#97182,#97183,#97184,#97185,
#97186,#97187,#97188,#97189,#97190,#97191,#97192,#97193,#97194,#97195,#97196,
#97197,#97198,#97199,#97200,#97201,#97202,#97203,#97204,#97205,#97206,#97207,
#97208,#97209,#97210,#97211,#97212),.UNSPECIFIED.,.F.,.F.)
B_SPLINE_CURVE_WITH_KNOTS((6,1,1,1,1,1,1,1,1,1,1,1,1,1,1,1,1,1,1,1,1,1,
1,1,1,1,1,1,1,1,6),(0.,0.0333333333333333,0.0666666666666667,0.1,0.133333333333333,
0.166666666666667,0.2,0.233333333333333,0.266666666666667,0.3,0.333333333333333,
0.366666666666667,0.4,0.433333333333333,0.466666666666667,0.5,0.533333333333333,
0.566666666666667,0.6,0.633333333333333,0.666666666666667,0.7,0.733333333333333,
0.766666666666667,0.8,0.833333333333333,0.866666666666667,0.9,0.933333333333333,
0.966666666666667,1.),.UNSPECIFIED.)
CURVE()
GEOMETRIC_REPRESENTATION_ITEM()
RATIONAL_B_SPLINE_CURVE((1.,1.,1.,1.,1.,1.,1.,1.,1.,1.,1.,1.,1.,1.,1.,1.,
1.,1.,1.,1.,1.,1.,1.,1.,1.,1.,1.,1.,1.,1.,1.,1.,1.,1.,1.))
REPRESENTATION_ITEM('')
);
#204=(
BOUNDED_CURVE()
B_SPLINE_CURVE(5,(#97214,#97215,#97216,#97217,#97218,#97219,#97220,#97221,
#97222,#97223,#97224,#97225,#97226,#97227,#97228,#97229,#97230,#97231,#97232,
#97233,#97234,#97235,#97236,#97237,#97238,#97239,#97240,#97241,#97242,#97243,
#97244,#97245,#97246,#97247,#97248),.UNSPECIFIED.,.F.,.F.)
B_SPLINE_CURVE_WITH_KNOTS((6,1,1,1,1,1,1,1,1,1,1,1,1,1,1,1,1,1,1,1,1,1,
1,1,1,1,1,1,1,1,6),(-1.,-0.966666666666667,-0.933333333333333,-0.9,-0.866666666666667,
-0.833333333333333,-0.8,-0.766666666666667,-0.733333333333333,-0.7,-0.666666666666667,
-0.633333333333333,-0.6,-0.566666666666667,-0.533333333333333,-0.5,-0.466666666666667,
-0.433333333333333,-0.4,-0.366666666666667,-0.333333333333333,-0.3,-0.266666666666667,
-0.233333333333333,-0.2,-0.166666666666667,-0.133333333333333,-0.1,-0.0666666666666667,
-0.0333333333333333,0.),.UNSPECIFIED.)
CURVE()
GEOMETRIC_REPRESENTATION_ITEM()
RATIONAL_B_SPLINE_CURVE((1.,1.,1.,1.,1.,1.,1.,1.,1.,1.,1.,1.,1.,1.,1.,1.,
1.,1.,1.,1.,1.,1.,1.,1.,1.,1.,1.,1.,1.,1.,1.,1.,1.,1.,1.))
REPRESENTATION_ITEM('')
);
#205=(
BOUNDED_CURVE()
B_SPLINE_CURVE(5,(#97326,#97327,#97328,#97329,#97330,#97331,#97332,#97333,
#97334,#97335,#97336,#97337,#97338,#97339,#97340,#97341,#97342,#97343,#97344,
#97345,#97346,#97347,#97348,#97349,#97350,#97351,#97352,#97353,#97354,#97355,
#97356,#97357,#97358,#97359,#97360),.UNSPECIFIED.,.F.,.F.)
B_SPLINE_CURVE_WITH_KNOTS((6,1,1,1,1,1,1,1,1,1,1,1,1,1,1,1,1,1,1,1,1,1,
1,1,1,1,1,1,1,1,6),(0.,0.0333333333333333,0.0666666666666667,0.1,0.133333333333333,
0.166666666666667,0.2,0.233333333333333,0.266666666666667,0.3,0.333333333333333,
0.366666666666667,0.4,0.433333333333333,0.466666666666667,0.5,0.533333333333333,
0.566666666666667,0.6,0.633333333333333,0.666666666666667,0.7,0.733333333333333,
0.766666666666667,0.8,0.833333333333333,0.866666666666667,0.9,0.933333333333333,
0.966666666666667,1.),.UNSPECIFIED.)
CURVE()
GEOMETRIC_REPRESENTATION_ITEM()
RATIONAL_B_SPLINE_CURVE((1.,1.,1.,1.,1.,1.,1.,1.,1.,1.,1.,1.,1.,1.,1.,1.,
1.,1.,1.,1.,1.,1.,1.,1.,1.,1.,1.,1.,1.,1.,1.,1.,1.,1.,1.))
REPRESENTATION_ITEM('')
);
#206=(
BOUNDED_CURVE()
B_SPLINE_CURVE(5,(#97361,#97362,#97363,#97364,#97365,#97366,#97367,#97368,
#97369,#97370,#97371,#97372,#97373,#97374,#97375,#97376,#97377,#97378,#97379,
#97380,#97381,#97382,#97383,#97384,#97385,#97386,#97387,#97388,#97389,#97390,
#97391,#97392,#97393,#97394,#97395),.UNSPECIFIED.,.F.,.F.)
B_SPLINE_CURVE_WITH_KNOTS((6,1,1,1,1,1,1,1,1,1,1,1,1,1,1,1,1,1,1,1,1,1,
1,1,1,1,1,1,1,1,6),(0.,0.0333333333333333,0.0666666666666667,0.1,0.133333333333333,
0.166666666666667,0.2,0.233333333333333,0.266666666666667,0.3,0.333333333333333,
0.366666666666667,0.4,0.433333333333333,0.466666666666667,0.5,0.533333333333333,
0.566666666666667,0.6,0.633333333333333,0.666666666666667,0.7,0.733333333333333,
0.766666666666667,0.8,0.833333333333333,0.866666666666667,0.9,0.933333333333333,
0.966666666666667,1.),.UNSPECIFIED.)
CURVE()
GEOMETRIC_REPRESENTATION_ITEM()
RATIONAL_B_SPLINE_CURVE((1.,1.,1.,1.,1.,1.,1.,1.,1.,1.,1.,1.,1.,1.,1.,1.,
1.,1.,1.,1.,1.,1.,1.,1.,1.,1.,1.,1.,1.,1.,1.,1.,1.,1.,1.))
REPRESENTATION_ITEM('')
);
#207=(
BOUNDED_CURVE()
B_SPLINE_CURVE(5,(#97474,#97475,#97476,#97477,#97478,#97479,#97480,#97481,
#97482,#97483,#97484,#97485,#97486,#97487,#97488,#97489,#97490,#97491,#97492,
#97493,#97494,#97495,#97496,#97497,#97498,#97499,#97500,#97501,#97502,#97503,
#97504,#97505,#97506,#97507,#97508),.UNSPECIFIED.,.F.,.F.)
B_SPLINE_CURVE_WITH_KNOTS((6,1,1,1,1,1,1,1,1,1,1,1,1,1,1,1,1,1,1,1,1,1,
1,1,1,1,1,1,1,1,6),(0.,0.0333333333333333,0.0666666666666667,0.1,0.133333333333333,
0.166666666666667,0.2,0.233333333333333,0.266666666666667,0.3,0.333333333333333,
0.366666666666667,0.4,0.433333333333333,0.466666666666667,0.5,0.533333333333333,
0.566666666666667,0.6,0.633333333333333,0.666666666666667,0.7,0.733333333333333,
0.766666666666667,0.8,0.833333333333333,0.866666666666667,0.9,0.933333333333333,
0.966666666666667,1.),.UNSPECIFIED.)
CURVE()
GEOMETRIC_REPRESENTATION_ITEM()
RATIONAL_B_SPLINE_CURVE((1.,1.,1.,1.,1.,1.,1.,1.,1.,1.,1.,1.,1.,1.,1.,1.,
1.,1.,1.,1.,1.,1.,1.,1.,1.,1.,1.,1.,1.,1.,1.,1.,1.,1.,1.))
REPRESENTATION_ITEM('')
);
#208=(
BOUNDED_CURVE()
B_SPLINE_CURVE(5,(#97510,#97511,#97512,#97513,#97514,#97515,#97516,#97517,
#97518,#97519,#97520,#97521,#97522,#97523,#97524,#97525,#97526,#97527,#97528,
#97529,#97530,#97531,#97532,#97533,#97534,#97535,#97536,#97537,#97538,#97539,
#97540,#97541,#97542,#97543,#97544),.UNSPECIFIED.,.F.,.F.)
B_SPLINE_CURVE_WITH_KNOTS((6,1,1,1,1,1,1,1,1,1,1,1,1,1,1,1,1,1,1,1,1,1,
1,1,1,1,1,1,1,1,6),(-1.,-0.966666666666667,-0.933333333333333,-0.9,-0.866666666666667,
-0.833333333333333,-0.8,-0.766666666666667,-0.733333333333333,-0.7,-0.666666666666667,
-0.633333333333333,-0.6,-0.566666666666667,-0.533333333333333,-0.5,-0.466666666666667,
-0.433333333333333,-0.4,-0.366666666666667,-0.333333333333333,-0.3,-0.266666666666667,
-0.233333333333333,-0.2,-0.166666666666667,-0.133333333333333,-0.1,-0.0666666666666667,
-0.0333333333333333,0.),.UNSPECIFIED.)
CURVE()
GEOMETRIC_REPRESENTATION_ITEM()
RATIONAL_B_SPLINE_CURVE((1.,1.,1.,1.,1.,1.,1.,1.,1.,1.,1.,1.,1.,1.,1.,1.,
1.,1.,1.,1.,1.,1.,1.,1.,1.,1.,1.,1.,1.,1.,1.,1.,1.,1.,1.))
REPRESENTATION_ITEM('')
);
#209=(
BOUNDED_CURVE()
B_SPLINE_CURVE(5,(#97623,#97624,#97625,#97626,#97627,#97628,#97629,#97630,
#97631,#97632,#97633,#97634,#97635,#97636,#97637,#97638,#97639,#97640,#97641,
#97642,#97643,#97644,#97645,#97646,#97647,#97648,#97649,#97650,#97651,#97652,
#97653,#97654,#97655,#97656,#97657),.UNSPECIFIED.,.F.,.F.)
B_SPLINE_CURVE_WITH_KNOTS((6,1,1,1,1,1,1,1,1,1,1,1,1,1,1,1,1,1,1,1,1,1,
1,1,1,1,1,1,1,1,6),(0.,0.0333333333333333,0.0666666666666667,0.1,0.133333333333333,
0.166666666666667,0.2,0.233333333333333,0.266666666666667,0.3,0.333333333333333,
0.366666666666667,0.4,0.433333333333333,0.466666666666667,0.5,0.533333333333333,
0.566666666666667,0.6,0.633333333333333,0.666666666666667,0.7,0.733333333333333,
0.766666666666667,0.8,0.833333333333333,0.866666666666667,0.9,0.933333333333333,
0.966666666666667,1.),.UNSPECIFIED.)
CURVE()
GEOMETRIC_REPRESENTATION_ITEM()
RATIONAL_B_SPLINE_CURVE((1.,1.,1.,1.,1.,1.,1.,1.,1.,1.,1.,1.,1.,1.,1.,1.,
1.,1.,1.,1.,1.,1.,1.,1.,1.,1.,1.,1.,1.,1.,1.,1.,1.,1.,1.))
REPRESENTATION_ITEM('')
);
#210=(
BOUNDED_CURVE()
B_SPLINE_CURVE(5,(#97659,#97660,#97661,#97662,#97663,#97664,#97665,#97666,
#97667,#97668,#97669,#97670,#97671,#97672,#97673,#97674,#97675,#97676,#97677,
#97678,#97679,#97680,#97681,#97682,#97683,#97684,#97685,#97686,#97687,#97688,
#97689,#97690,#97691,#97692,#97693),.UNSPECIFIED.,.F.,.F.)
B_SPLINE_CURVE_WITH_KNOTS((6,1,1,1,1,1,1,1,1,1,1,1,1,1,1,1,1,1,1,1,1,1,
1,1,1,1,1,1,1,1,6),(0.,0.0333333333333333,0.0666666666666667,0.1,0.133333333333333,
0.166666666666667,0.2,0.233333333333333,0.266666666666667,0.3,0.333333333333333,
0.366666666666667,0.4,0.433333333333333,0.466666666666667,0.5,0.533333333333333,
0.566666666666667,0.6,0.633333333333333,0.666666666666667,0.7,0.733333333333333,
0.766666666666667,0.8,0.833333333333333,0.866666666666667,0.9,0.933333333333333,
0.966666666666667,1.),.UNSPECIFIED.)
CURVE()
GEOMETRIC_REPRESENTATION_ITEM()
RATIONAL_B_SPLINE_CURVE((1.,1.,1.,1.,1.,1.,1.,1.,1.,1.,1.,1.,1.,1.,1.,1.,
1.,1.,1.,1.,1.,1.,1.,1.,1.,1.,1.,1.,1.,1.,1.,1.,1.,1.,1.))
REPRESENTATION_ITEM('')
);
#519=SHAPE_REPRESENTATION_RELATIONSHIP('SRR','None',#114056,#537);
#537=ADVANCED_BREP_SHAPE_REPRESENTATION('',(#573),#113970);
#555=STYLED_ITEM('',(#114303),#573);
#573=MANIFOLD_SOLID_BREP('Spur Pinion m0.5 z16 with Hub',#60396);
#636=CYLINDRICAL_SURFACE('',#61992,1.05);
#637=CYLINDRICAL_SURFACE('',#61998,4.50000000000305);
#638=CYLINDRICAL_SURFACE('',#62003,3.375);
#639=CYLINDRICAL_SURFACE('',#62039,4.50000000000305);
#640=CYLINDRICAL_SURFACE('',#62045,4.50000000000305);
#641=CYLINDRICAL_SURFACE('',#62051,4.50000000000305);
#642=CYLINDRICAL_SURFACE('',#62057,4.50000000000305);
#643=CYLINDRICAL_SURFACE('',#62063,4.50000000000305);
#644=CYLINDRICAL_SURFACE('',#62069,4.50000000000305);
#645=CYLINDRICAL_SURFACE('',#62075,4.50000000000305);
#646=CYLINDRICAL_SURFACE('',#62081,4.50000000000305);
#647=CYLINDRICAL_SURFACE('',#62087,4.50000000000305);
#648=CYLINDRICAL_SURFACE('',#62093,4.50000000000305);
#649=CYLINDRICAL_SURFACE('',#62099,4.50000000000305);
#650=CYLINDRICAL_SURFACE('',#62105,4.50000000000305);
#651=CYLINDRICAL_SURFACE('',#62111,4.50000000000305);
#652=CYLINDRICAL_SURFACE('',#62117,4.50000000000305);
#653=CYLINDRICAL_SURFACE('',#62122,4.50000000000305);
#654=CYLINDRICAL_SURFACE('',#62127,2.5);
#655=CYLINDRICAL_SURFACE('',#62133,4.49999999999999);
#913=CONICAL_SURFACE('',#62135,4.34999999999999,0.785398163397448);
#1063=CIRCLE('',#61991,1.05);
#1064=CIRCLE('',#61993,1.05);
#1065=CIRCLE('',#61994,1.05);
#1066=CIRCLE('',#61999,4.50000000000305);
#1067=CIRCLE('',#62000,4.50000000000305);
#1068=CIRCLE('',#62002,3.375);
#1069=CIRCLE('',#62004,3.375);
#1070=CIRCLE('',#62005,3.375);
#1071=CIRCLE('',#62006,3.375);
#1072=CIRCLE('',#62007,3.375);
#1073=CIRCLE('',#62008,3.375);
#1074=CIRCLE('',#62009,3.375);
#1075=CIRCLE('',#62010,3.375);
#1076=CIRCLE('',#62011,3.375);
#1077=CIRCLE('',#62012,3.375);
#1078=CIRCLE('',#62013,3.375);
#1079=CIRCLE('',#62014,3.375);
#1080=CIRCLE('',#62015,3.375);
#1081=CIRCLE('',#62016,3.375);
#1082=CIRCLE('',#62017,3.375);
#1083=CIRCLE('',#62018,3.375);
#1084=CIRCLE('',#62019,3.375);
#1085=CIRCLE('',#62020,3.375);
#1086=CIRCLE('',#62021,3.375);
#1087=CIRCLE('',#62022,3.375);
#1088=CIRCLE('',#62023,3.375);
#1089=CIRCLE('',#62024,3.375);
#1090=CIRCLE('',#62025,3.375);
#1091=CIRCLE('',#62026,3.375);
#1092=CIRCLE('',#62027,3.375);
#1093=CIRCLE('',#62028,3.375);
#1094=CIRCLE('',#62029,3.375);
#1095=CIRCLE('',#62030,3.375);
#1096=CIRCLE('',#62031,3.375);
#1097=CIRCLE('',#62032,3.375);
#1098=CIRCLE('',#62033,3.375);
#1099=CIRCLE('',#62034,3.375);
#1100=CIRCLE('',#62035,3.375);
#1101=CIRCLE('',#62036,3.375);
#1102=CIRCLE('',#62040,4.50000000000305);
#1103=CIRCLE('',#62041,4.50000000000305);
#1104=CIRCLE('',#62046,4.50000000000305);
#1105=CIRCLE('',#62047,4.50000000000305);
#1106=CIRCLE('',#62052,4.50000000000305);
#1107=CIRCLE('',#62053,4.50000000000305);
#1108=CIRCLE('',#62058,4.50000000000305);
#1109=CIRCLE('',#62059,4.50000000000305);
#1110=CIRCLE('',#62064,4.50000000000305);
#1111=CIRCLE('',#62065,4.50000000000305);
#1112=CIRCLE('',#62070,4.50000000000305);
#1113=CIRCLE('',#62071,4.50000000000305);
#1114=CIRCLE('',#62076,4.50000000000305);
#1115=CIRCLE('',#62077,4.50000000000305);
#1116=CIRCLE('',#62082,4.50000000000305);
#1117=CIRCLE('',#62083,4.50000000000305);
#1118=CIRCLE('',#62088,4.50000000000305);
#1119=CIRCLE('',#62089,4.50000000000305);
#1120=CIRCLE('',#62094,4.50000000000305);
#1121=CIRCLE('',#62095,4.50000000000305);
#1122=CIRCLE('',#62100,4.50000000000305);
#1123=CIRCLE('',#62101,4.50000000000305);
#1124=CIRCLE('',#62106,4.50000000000305);
#1125=CIRCLE('',#62107,4.50000000000305);
#1126=CIRCLE('',#62112,4.50000000000305);
#1127=CIRCLE('',#62113,4.50000000000305);
#1128=CIRCLE('',#62118,4.50000000000305);
#1129=CIRCLE('',#62119,4.50000000000305);
#1130=CIRCLE('',#62123,4.50000000000305);
#1131=CIRCLE('',#62124,4.50000000000305);
#1132=CIRCLE('',#62128,2.5);
#1133=CIRCLE('',#62129,2.5);
#1134=CIRCLE('',#62132,4.49999999999999);
#1135=CIRCLE('',#62134,4.49999999999999);
#1136=CIRCLE('',#62136,4.2);
#1827=FACE_BOUND('',#9631,.T.);
#1828=FACE_BOUND('',#9633,.T.);
#1829=FACE_BOUND('',#9635,.T.);
#1830=FACE_BOUND('',#9637,.T.);
#1831=FACE_BOUND('',#9640,.T.);
#3043=PLANE('',#61990);
#3044=PLANE('',#61995);
#3045=PLANE('',#61996);
#3046=PLANE('',#61997);
#3047=PLANE('',#62001);
#3048=PLANE('',#62037);
#3049=PLANE('',#62038);
#3050=PLANE('',#62042);
#3051=PLANE('',#62043);
#3052=PLANE('',#62044);
#3053=PLANE('',#62048);
#3054=PLANE('',#62049);
#3055=PLANE('',#62050);
#3056=PLANE('',#62054);
#3057=PLANE('',#62055);
#3058=PLANE('',#62056);
#3059=PLANE('',#62060);
#3060=PLANE('',#62061);
#3061=PLANE('',#62062);
#3062=PLANE('',#62066);
#3063=PLANE('',#62067);
#3064=PLANE('',#62068);
#3065=PLANE('',#62072);
#3066=PLANE('',#62073);
#3067=PLANE('',#62074);
#3068=PLANE('',#62078);
#3069=PLANE('',#62079);
#3070=PLANE('',#62080);
#3071=PLANE('',#62084);
#3072=PLANE('',#62085);
#3073=PLANE('',#62086);
#3074=PLANE('',#62090);
#3075=PLANE('',#62091);
#3076=PLANE('',#62092);
#3077=PLANE('',#62096);
#3078=PLANE('',#62097);
#3079=PLANE('',#62098);
#3080=PLANE('',#62102);
#3081=PLANE('',#62103);
#3082=PLANE('',#62104);
#3083=PLANE('',#62108);
#3084=PLANE('',#62109);
#3085=PLANE('',#62110);
#3086=PLANE('',#62114);
#3087=PLANE('',#62115);
#3088=PLANE('',#62116);
#3089=PLANE('',#62120);
#3090=PLANE('',#62121);
#3091=PLANE('',#62125);
#3092=PLANE('',#62126);
#3093=PLANE('',#62130);
#3094=PLANE('',#62131);
#3095=PLANE('',#62137);
#5978=FACE_OUTER_BOUND('',#9530,.T.);
#5979=FACE_OUTER_BOUND('',#9531,.T.);
#5980=FACE_OUTER_BOUND('',#9532,.T.);
#5981=FACE_OUTER_BOUND('',#9533,.T.);
#5982=FACE_OUTER_BOUND('',#9534,.T.);
#5983=FACE_OUTER_BOUND('',#9535,.T.);
#5984=FACE_OUTER_BOUND('',#9536,.T.);
#5985=FACE_OUTER_BOUND('',#9537,.T.);
#5986=FACE_OUTER_BOUND('',#9538,.T.);
#5987=FACE_OUTER_BOUND('',#9539,.T.);
#5988=FACE_OUTER_BOUND('',#9540,.T.);
#5989=FACE_OUTER_BOUND('',#9541,.T.);
#5990=FACE_OUTER_BOUND('',#9542,.T.);
#5991=FACE_OUTER_BOUND('',#9543,.T.);
#5992=FACE_OUTER_BOUND('',#9544,.T.);
#5993=FACE_OUTER_BOUND('',#9545,.T.);
#5994=FACE_OUTER_BOUND('',#9546,.T.);
#5995=FACE_OUTER_BOUND('',#9547,.T.);
#5996=FACE_OUTER_BOUND('',#9548,.T.);
#5997=FACE_OUTER_BOUND('',#9549,.T.);
#5998=FACE_OUTER_BOUND('',#9550,.T.);
#5999=FACE_OUTER_BOUND('',#9551,.T.);
#6000=FACE_OUTER_BOUND('',#9552,.T.);
#6001=FACE_OUTER_BOUND('',#9553,.T.);
#6002=FACE_OUTER_BOUND('',#9554,.T.);
#6003=FACE_OUTER_BOUND('',#9555,.T.);
#6004=FACE_OUTER_BOUND('',#9556,.T.);
#6005=FACE_OUTER_BOUND('',#9557,.T.);
#6006=FACE_OUTER_BOUND('',#9558,.T.);
#6007=FACE_OUTER_BOUND('',#9559,.T.);
#6008=FACE_OUTER_BOUND('',#9560,.T.);
#6009=FACE_OUTER_BOUND('',#9561,.T.);
#6010=FACE_OUTER_BOUND('',#9562,.T.);
#6011=FACE_OUTER_BOUND('',#9563,.T.);
#6012=FACE_OUTER_BOUND('',#9564,.T.);
#6013=FACE_OUTER_BOUND('',#9565,.T.);
#6014=FACE_OUTER_BOUND('',#9566,.T.);
#6015=FACE_OUTER_BOUND('',#9567,.T.);
#6016=FACE_OUTER_BOUND('',#9568,.T.);
#6017=FACE_OUTER_BOUND('',#9569,.T.);
#6018=FACE_OUTER_BOUND('',#9570,.T.);
#6019=FACE_OUTER_BOUND('',#9571,.T.);
#6020=FACE_OUTER_BOUND('',#9572,.T.);
#6021=FACE_OUTER_BOUND('',#9573,.T.);
#6022=FACE_OUTER_BOUND('',#9574,.T.);
#6023=FACE_OUTER_BOUND('',#9575,.T.);
#6024=FACE_OUTER_BOUND('',#9576,.T.);
#6025=FACE_OUTER_BOUND('',#9577,.T.);
#6026=FACE_OUTER_BOUND('',#9578,.T.);
#6027=FACE_OUTER_BOUND('',#9579,.T.);
#6028=FACE_OUTER_BOUND('',#9580,.T.);
#6029=FACE_OUTER_BOUND('',#9581,.T.);
#6030=FACE_OUTER_BOUND('',#9582,.T.);
#6031=FACE_OUTER_BOUND('',#9583,.T.);
#6032=FACE_OUTER_BOUND('',#9584,.T.);
#6033=FACE_OUTER_BOUND('',#9585,.T.);
#6034=FACE_OUTER_BOUND('',#9586,.T.);
#6035=FACE_OUTER_BOUND('',#9587,.T.);
#6036=FACE_OUTER_BOUND('',#9588,.T.);
#6037=FACE_OUTER_BOUND('',#9589,.T.);
#6038=FACE_OUTER_BOUND('',#9590,.T.);
#6039=FACE_OUTER_BOUND('',#9591,.T.);
#6040=FACE_OUTER_BOUND('',#9592,.T.);
#6041=FACE_OUTER_BOUND('',#9593,.T.);
#6042=FACE_OUTER_BOUND('',#9594,.T.);
#6043=FACE_OUTER_BOUND('',#9595,.T.);
#6044=FACE_OUTER_BOUND('',#9596,.T.);
#6045=FACE_OUTER_BOUND('',#9597,.T.);
#6046=FACE_OUTER_BOUND('',#9598,.T.);
#6047=FACE_OUTER_BOUND('',#9599,.T.);
#6048=FACE_OUTER_BOUND('',#9600,.T.);
#6049=FACE_OUTER_BOUND('',#9601,.T.);
#6050=FACE_OUTER_BOUND('',#9602,.T.);
#6051=FACE_OUTER_BOUND('',#9603,.T.);
#6052=FACE_OUTER_BOUND('',#9604,.T.);
#6053=FACE_OUTER_BOUND('',#9605,.T.);
#6054=FACE_OUTER_BOUND('',#9606,.T.);
#6055=FACE_OUTER_BOUND('',#9607,.T.);
#6056=FACE_OUTER_BOUND('',#9608,.T.);
#6057=FACE_OUTER_BOUND('',#9609,.T.);
#6058=FACE_OUTER_BOUND('',#9610,.T.);
#6059=FACE_OUTER_BOUND('',#9611,.T.);
#6060=FACE_OUTER_BOUND('',#9612,.T.);
#6061=FACE_OUTER_BOUND('',#9613,.T.);
#6062=FACE_OUTER_BOUND('',#9614,.T.);
#6063=FACE_OUTER_BOUND('',#9615,.T.);
#6064=FACE_OUTER_BOUND('',#9616,.T.);
#6065=FACE_OUTER_BOUND('',#9617,.T.);
#6066=FACE_OUTER_BOUND('',#9618,.T.);
#6067=FACE_OUTER_BOUND('',#9619,.T.);
#6068=FACE_OUTER_BOUND('',#9620,.T.);
#6069=FACE_OUTER_BOUND('',#9621,.T.);
#6070=FACE_OUTER_BOUND('',#9622,.T.);
#6071=FACE_OUTER_BOUND('',#9623,.T.);
#6072=FACE_OUTER_BOUND('',#9624,.T.);
#6073=FACE_OUTER_BOUND('',#9625,.T.);
#6074=FACE_OUTER_BOUND('',#9626,.T.);
#6075=FACE_OUTER_BOUND('',#9627,.T.);
#6076=FACE_OUTER_BOUND('',#9628,.T.);
#6077=FACE_OUTER_BOUND('',#9629,.T.);
#6078=FACE_OUTER_BOUND('',#9630,.T.);
#6079=FACE_OUTER_BOUND('',#9632,.T.);
#6080=FACE_OUTER_BOUND('',#9634,.T.);
#6081=FACE_OUTER_BOUND('',#9636,.T.);
#6082=FACE_OUTER_BOUND('',#9638,.T.);
#6083=FACE_OUTER_BOUND('',#9639,.T.);
#9530=EDGE_LOOP('',(#48987,#48988));
#9531=EDGE_LOOP('',(#48989,#48990,#48991,#48992,#48993,#48994,#48995,#48996,
#48997,#48998));
#9532=EDGE_LOOP('',(#48999,#49000,#49001));
#9533=EDGE_LOOP('',(#49002,#49003,#49004,#49005));
#9534=EDGE_LOOP('',(#49006,#49007,#49008,#49009));
#9535=EDGE_LOOP('',(#49010,#49011,#49012,#49013));
#9536=EDGE_LOOP('',(#49014,#49015,#49016,#49017));
#9537=EDGE_LOOP('',(#49018,#49019,#49020,#49021));
#9538=EDGE_LOOP('',(#49022,#49023,#49024,#49025,#49026,#49027));
#9539=EDGE_LOOP('',(#49028,#49029,#49030,#49031,#49032,#49033,#49034,#49035,
#49036,#49037,#49038,#49039,#49040,#49041,#49042,#49043,#49044,#49045,#49046,
#49047,#49048,#49049,#49050,#49051,#49052,#49053,#49054,#49055,#49056,#49057,
#49058,#49059,#49060,#49061,#49062,#49063,#49064,#49065,#49066,#49067,#49068,
#49069,#49070,#49071,#49072,#49073,#49074,#49075,#49076,#49077,#49078,#49079,
#49080,#49081,#49082,#49083,#49084,#49085,#49086,#49087,#49088,#49089,#49090,
#49091,#49092,#49093,#49094,#49095));
#9540=EDGE_LOOP('',(#49096,#49097,#49098,#49099));
#9541=EDGE_LOOP('',(#49100,#49101,#49102,#49103));
#9542=EDGE_LOOP('',(#49104,#49105,#49106,#49107));
#9543=EDGE_LOOP('',(#49108,#49109,#49110,#49111));
#9544=EDGE_LOOP('',(#49112,#49113,#49114,#49115));
#9545=EDGE_LOOP('',(#49116,#49117,#49118,#49119,#49120,#49121));
#9546=EDGE_LOOP('',(#49122,#49123,#49124,#49125));
#9547=EDGE_LOOP('',(#49126,#49127,#49128,#49129));
#9548=EDGE_LOOP('',(#49130,#49131,#49132,#49133));
#9549=EDGE_LOOP('',(#49134,#49135,#49136,#49137));
#9550=EDGE_LOOP('',(#49138,#49139,#49140,#49141));
#9551=EDGE_LOOP('',(#49142,#49143,#49144,#49145,#49146,#49147));
#9552=EDGE_LOOP('',(#49148,#49149,#49150,#49151));
#9553=EDGE_LOOP('',(#49152,#49153,#49154,#49155));
#9554=EDGE_LOOP('',(#49156,#49157,#49158,#49159));
#9555=EDGE_LOOP('',(#49160,#49161,#49162,#49163));
#9556=EDGE_LOOP('',(#49164,#49165,#49166,#49167));
#9557=EDGE_LOOP('',(#49168,#49169,#49170,#49171,#49172,#49173,#49174));
#9558=EDGE_LOOP('',(#49175,#49176,#49177,#49178));
#9559=EDGE_LOOP('',(#49179,#49180,#49181,#49182));
#9560=EDGE_LOOP('',(#49183,#49184,#49185,#49186));
#9561=EDGE_LOOP('',(#49187,#49188,#49189,#49190));
#9562=EDGE_LOOP('',(#49191,#49192,#49193,#49194));
#9563=EDGE_LOOP('',(#49195,#49196,#49197,#49198,#49199,#49200));
#9564=EDGE_LOOP('',(#49201,#49202,#49203,#49204));
#9565=EDGE_LOOP('',(#49205,#49206,#49207,#49208));
#9566=EDGE_LOOP('',(#49209,#49210,#49211,#49212));
#9567=EDGE_LOOP('',(#49213,#49214,#49215,#49216));
#9568=EDGE_LOOP('',(#49217,#49218,#49219,#49220));
#9569=EDGE_LOOP('',(#49221,#49222,#49223,#49224,#49225,#49226));
#9570=EDGE_LOOP('',(#49227,#49228,#49229,#49230));
#9571=EDGE_LOOP('',(#49231,#49232,#49233,#49234));
#9572=EDGE_LOOP('',(#49235,#49236,#49237,#49238));
#9573=EDGE_LOOP('',(#49239,#49240,#49241,#49242));
#9574=EDGE_LOOP('',(#49243,#49244,#49245,#49246));
#9575=EDGE_LOOP('',(#49247,#49248,#49249,#49250,#49251,#49252));
#9576=EDGE_LOOP('',(#49253,#49254,#49255,#49256));
#9577=EDGE_LOOP('',(#49257,#49258,#49259,#49260));
#9578=EDGE_LOOP('',(#49261,#49262,#49263,#49264));
#9579=EDGE_LOOP('',(#49265,#49266,#49267,#49268));
#9580=EDGE_LOOP('',(#49269,#49270,#49271,#49272));
#9581=EDGE_LOOP('',(#49273,#49274,#49275,#49276,#49277,#49278));
#9582=EDGE_LOOP('',(#49279,#49280,#49281,#49282));
#9583=EDGE_LOOP('',(#49283,#49284,#49285,#49286));
#9584=EDGE_LOOP('',(#49287,#49288,#49289,#49290));
#9585=EDGE_LOOP('',(#49291,#49292,#49293,#49294));
#9586=EDGE_LOOP('',(#49295,#49296,#49297,#49298));
#9587=EDGE_LOOP('',(#49299,#49300,#49301,#49302,#49303,#49304));
#9588=EDGE_LOOP('',(#49305,#49306,#49307,#49308));
#9589=EDGE_LOOP('',(#49309,#49310,#49311,#49312));
#9590=EDGE_LOOP('',(#49313,#49314,#49315,#49316));
#9591=EDGE_LOOP('',(#49317,#49318,#49319,#49320));
#9592=EDGE_LOOP('',(#49321,#49322,#49323,#49324));
#9593=EDGE_LOOP('',(#49325,#49326,#49327,#49328,#49329,#49330));
#9594=EDGE_LOOP('',(#49331,#49332,#49333,#49334));
#9595=EDGE_LOOP('',(#49335,#49336,#49337,#49338));
#9596=EDGE_LOOP('',(#49339,#49340,#49341,#49342));
#9597=EDGE_LOOP('',(#49343,#49344,#49345,#49346));
#9598=EDGE_LOOP('',(#49347,#49348,#49349,#49350));
#9599=EDGE_LOOP('',(#49351,#49352,#49353,#49354,#49355,#49356));
#9600=EDGE_LOOP('',(#49357,#49358,#49359,#49360));
#9601=EDGE_LOOP('',(#49361,#49362,#49363,#49364));
#9602=EDGE_LOOP('',(#49365,#49366,#49367,#49368));
#9603=EDGE_LOOP('',(#49369,#49370,#49371,#49372));
#9604=EDGE_LOOP('',(#49373,#49374,#49375,#49376));
#9605=EDGE_LOOP('',(#49377,#49378,#49379,#49380,#49381,#49382));
#9606=EDGE_LOOP('',(#49383,#49384,#49385,#49386));
#9607=EDGE_LOOP('',(#49387,#49388,#49389,#49390));
#9608=EDGE_LOOP('',(#49391,#49392,#49393,#49394));
#9609=EDGE_LOOP('',(#49395,#49396,#49397,#49398));
#9610=EDGE_LOOP('',(#49399,#49400,#49401,#49402));
#9611=EDGE_LOOP('',(#49403,#49404,#49405,#49406,#49407,#49408));
#9612=EDGE_LOOP('',(#49409,#49410,#49411,#49412));
#9613=EDGE_LOOP('',(#49413,#49414,#49415,#49416));
#9614=EDGE_LOOP('',(#49417,#49418,#49419,#49420));
#9615=EDGE_LOOP('',(#49421,#49422,#49423,#49424));
#9616=EDGE_LOOP('',(#49425,#49426,#49427,#49428));
#9617=EDGE_LOOP('',(#49429,#49430,#49431,#49432,#49433,#49434));
#9618=EDGE_LOOP('',(#49435,#49436,#49437,#49438));
#9619=EDGE_LOOP('',(#49439,#49440,#49441,#49442));
#9620=EDGE_LOOP('',(#49443,#49444,#49445,#49446));
#9621=EDGE_LOOP('',(#49447,#49448,#49449,#49450));
#9622=EDGE_LOOP('',(#49451,#49452,#49453,#49454));
#9623=EDGE_LOOP('',(#49455,#49456,#49457,#49458,#49459,#49460));
#9624=EDGE_LOOP('',(#49461,#49462,#49463,#49464));
#9625=EDGE_LOOP('',(#49465,#49466,#49467,#49468));
#9626=EDGE_LOOP('',(#49469,#49470,#49471,#49472));
#9627=EDGE_LOOP('',(#49473,#49474,#49475,#49476));
#9628=EDGE_LOOP('',(#49477,#49478,#49479,#49480));
#9629=EDGE_LOOP('',(#49481,#49482,#49483,#49484,#49485,#49486));
#9630=EDGE_LOOP('',(#49487,#49488,#49489,#49490));
#9631=EDGE_LOOP('',(#49491,#49492,#49493,#49494));
#9632=EDGE_LOOP('',(#49495,#49496,#49497,#49498,#49499,#49500,#49501,#49502,
#49503,#49504,#49505,#49506,#49507,#49508,#49509,#49510,#49511,#49512,#49513,
#49514,#49515,#49516,#49517,#49518,#49519,#49520,#49521,#49522,#49523,#49524,
#49525,#49526,#49527,#49528,#49529,#49530,#49531,#49532,#49533,#49534,#49535,
#49536,#49537,#49538,#49539,#49540,#49541,#49542,#49543,#49544,#49545,#49546,
#49547,#49548,#49549,#49550,#49551,#49552,#49553,#49554,#49555,#49556,#49557,
#49558,#49559,#49560,#49561,#49562,#49563,#49564,#49565,#49566,#49567,#49568,
#49569,#49570,#49571,#49572,#49573,#49574,#49575,#49576,#49577,#49578,#49579,
#49580,#49581,#49582,#49583,#49584,#49585,#49586,#49587,#49588,#49589,#49590));
#9633=EDGE_LOOP('',(#49591));
#9634=EDGE_LOOP('',(#49592));
#9635=EDGE_LOOP('',(#49593));
#9636=EDGE_LOOP('',(#49594,#49595,#49596,#49597));
#9637=EDGE_LOOP('',(#49598,#49599,#49600));
#9638=EDGE_LOOP('',(#49601,#49602,#49603,#49604));
#9639=EDGE_LOOP('',(#49605));
#9640=EDGE_LOOP('',(#49606));
#14329=LINE('',#92660,#20363);
#14330=LINE('',#92706,#20364);
#14331=LINE('',#92732,#20365);
#14332=LINE('',#92736,#20366);
#14333=LINE('',#92738,#20367);
#14334=LINE('',#92740,#20368);
#14335=LINE('',#92741,#20369);
#14336=LINE('',#92745,#20370);
#14337=LINE('',#92747,#20371);
#14338=LINE('',#92749,#20372);
#14339=LINE('',#92750,#20373);
#14340=LINE('',#92893,#20374);
#14341=LINE('',#92899,#20375);
#14342=LINE('',#93046,#20376);
#14343=LINE('',#93050,#20377);
#14344=LINE('',#93054,#20378);
#14345=LINE('',#93058,#20379);
#14346=LINE('',#93062,#20380);
#14347=LINE('',#93066,#20381);
#14348=LINE('',#93071,#20382);
#14349=LINE('',#93075,#20383);
#14350=LINE('',#93079,#20384);
#14351=LINE('',#93083,#20385);
#14352=LINE('',#93087,#20386);
#14353=LINE('',#93091,#20387);
#14354=LINE('',#93095,#20388);
#14355=LINE('',#93099,#20389);
#14356=LINE('',#93103,#20390);
#14357=LINE('',#93107,#20391);
#14358=LINE('',#93111,#20392);
#14359=LINE('',#93115,#20393);
#14360=LINE('',#93119,#20394);
#14361=LINE('',#93123,#20395);
#14362=LINE('',#93127,#20396);
#14363=LINE('',#93131,#20397);
#14364=LINE('',#93135,#20398);
#14365=LINE('',#93139,#20399);
#14366=LINE('',#93143,#20400);
#14367=LINE('',#93147,#20401);
#14368=LINE('',#93151,#20402);
#14369=LINE('',#93155,#20403);
#14370=LINE('',#93159,#20404);
#14371=LINE('',#93163,#20405);
#14372=LINE('',#93167,#20406);
#14373=LINE('',#93171,#20407);
#14374=LINE('',#93173,#20408);
#14375=LINE('',#93174,#20409);
#14376=LINE('',#93177,#20410);
#14377=LINE('',#93179,#20411);
#14378=LINE('',#93180,#20412);
#14379=LINE('',#93323,#20413);
#14380=LINE('',#93329,#20414);
#14381=LINE('',#93473,#20415);
#14382=LINE('',#93475,#20416);
#14383=LINE('',#93476,#20417);
#14384=LINE('',#93479,#20418);
#14385=LINE('',#93481,#20419);
#14386=LINE('',#93482,#20420);
#14387=LINE('',#93625,#20421);
#14388=LINE('',#93631,#20422);
#14389=LINE('',#93775,#20423);
#14390=LINE('',#93777,#20424);
#14391=LINE('',#93778,#20425);
#14392=LINE('',#93781,#20426);
#14393=LINE('',#93783,#20427);
#14394=LINE('',#93784,#20428);
#14395=LINE('',#93927,#20429);
#14396=LINE('',#93933,#20430);
#14397=LINE('',#94077,#20431);
#14398=LINE('',#94079,#20432);
#14399=LINE('',#94080,#20433);
#14400=LINE('',#94083,#20434);
#14401=LINE('',#94085,#20435);
#14402=LINE('',#94086,#20436);
#14403=LINE('',#94229,#20437);
#14404=LINE('',#94235,#20438);
#14405=LINE('',#94379,#20439);
#14406=LINE('',#94381,#20440);
#14407=LINE('',#94382,#20441);
#14408=LINE('',#94385,#20442);
#14409=LINE('',#94387,#20443);
#14410=LINE('',#94388,#20444);
#14411=LINE('',#94531,#20445);
#14412=LINE('',#94537,#20446);
#14413=LINE('',#94681,#20447);
#14414=LINE('',#94683,#20448);
#14415=LINE('',#94684,#20449);
#14416=LINE('',#94687,#20450);
#14417=LINE('',#94689,#20451);
#14418=LINE('',#94690,#20452);
#14419=LINE('',#94833,#20453);
#14420=LINE('',#94839,#20454);
#14421=LINE('',#94983,#20455);
#14422=LINE('',#94985,#20456);
#14423=LINE('',#94986,#20457);
#14424=LINE('',#94989,#20458);
#14425=LINE('',#94991,#20459);
#14426=LINE('',#94992,#20460);
#14427=LINE('',#95135,#20461);
#14428=LINE('',#95141,#20462);
#14429=LINE('',#95285,#20463);
#14430=LINE('',#95287,#20464);
#14431=LINE('',#95288,#20465);
#14432=LINE('',#95291,#20466);
#14433=LINE('',#95293,#20467);
#14434=LINE('',#95294,#20468);
#14435=LINE('',#95437,#20469);
#14436=LINE('',#95443,#20470);
#14437=LINE('',#95587,#20471);
#14438=LINE('',#95589,#20472);
#14439=LINE('',#95590,#20473);
#14440=LINE('',#95593,#20474);
#14441=LINE('',#95595,#20475);
#14442=LINE('',#95596,#20476);
#14443=LINE('',#95739,#20477);
#14444=LINE('',#95745,#20478);
#14445=LINE('',#95889,#20479);
#14446=LINE('',#95891,#20480);
#14447=LINE('',#95892,#20481);
#14448=LINE('',#95895,#20482);
#14449=LINE('',#95897,#20483);
#14450=LINE('',#95898,#20484);
#14451=LINE('',#96041,#20485);
#14452=LINE('',#96047,#20486);
#14453=LINE('',#96191,#20487);
#14454=LINE('',#96193,#20488);
#14455=LINE('',#96194,#20489);
#14456=LINE('',#96197,#20490);
#14457=LINE('',#96199,#20491);
#14458=LINE('',#96200,#20492);
#14459=LINE('',#96343,#20493);
#14460=LINE('',#96349,#20494);
#14461=LINE('',#96493,#20495);
#14462=LINE('',#96495,#20496);
#14463=LINE('',#96496,#20497);
#14464=LINE('',#96499,#20498);
#14465=LINE('',#96501,#20499);
#14466=LINE('',#96502,#20500);
#14467=LINE('',#96645,#20501);
#14468=LINE('',#96651,#20502);
#14469=LINE('',#96795,#20503);
#14470=LINE('',#96797,#20504);
#14471=LINE('',#96798,#20505);
#14472=LINE('',#96801,#20506);
#14473=LINE('',#96803,#20507);
#14474=LINE('',#96804,#20508);
#14475=LINE('',#96947,#20509);
#14476=LINE('',#96953,#20510);
#14477=LINE('',#97097,#20511);
#14478=LINE('',#97099,#20512);
#14479=LINE('',#97100,#20513);
#14480=LINE('',#97103,#20514);
#14481=LINE('',#97105,#20515);
#14482=LINE('',#97106,#20516);
#14483=LINE('',#97249,#20517);
#14484=LINE('',#97255,#20518);
#14485=LINE('',#97399,#20519);
#14486=LINE('',#97401,#20520);
#14487=LINE('',#97402,#20521);
#14488=LINE('',#97545,#20522);
#14489=LINE('',#97551,#20523);
#14490=LINE('',#97694,#20524);
#14491=LINE('',#97696,#20525);
#14492=LINE('',#97697,#20526);
#14493=LINE('',#97703,#20527);
#14494=LINE('',#97712,#20528);
#14495=LINE('',#97716,#20529);
#20363=VECTOR('',#69993,10.);
#20364=VECTOR('',#69998,1.05);
#20365=VECTOR('',#70005,10.);
#20366=VECTOR('',#70008,10.);
#20367=VECTOR('',#70009,10.);
#20368=VECTOR('',#70010,10.);
#20369=VECTOR('',#70011,10.);
#20370=VECTOR('',#70014,10.);
#20371=VECTOR('',#70015,10.);
#20372=VECTOR('',#70016,10.);
#20373=VECTOR('',#70017,10.);
#20374=VECTOR('',#70018,10.);
#20375=VECTOR('',#70025,10.);
#20376=VECTOR('',#70034,3.375);
#20377=VECTOR('',#70037,10.);
#20378=VECTOR('',#70040,10.);
#20379=VECTOR('',#70043,10.);
#20380=VECTOR('',#70046,10.);
#20381=VECTOR('',#70049,10.);
#20382=VECTOR('',#70054,10.);
#20383=VECTOR('',#70057,10.);
#20384=VECTOR('',#70060,10.);
#20385=VECTOR('',#70063,10.);
#20386=VECTOR('',#70066,10.);
#20387=VECTOR('',#70069,10.);
#20388=VECTOR('',#70072,10.);
#20389=VECTOR('',#70075,10.);
#20390=VECTOR('',#70078,10.);
#20391=VECTOR('',#70081,10.);
#20392=VECTOR('',#70084,10.);
#20393=VECTOR('',#70087,10.);
#20394=VECTOR('',#70090,10.);
#20395=VECTOR('',#70093,10.);
#20396=VECTOR('',#70096,10.);
#20397=VECTOR('',#70099,10.);
#20398=VECTOR('',#70102,10.);
#20399=VECTOR('',#70105,10.);
#20400=VECTOR('',#70108,10.);
#20401=VECTOR('',#70111,10.);
#20402=VECTOR('',#70114,10.);
#20403=VECTOR('',#70117,10.);
#20404=VECTOR('',#70120,10.);
#20405=VECTOR('',#70123,10.);
#20406=VECTOR('',#70126,10.);
#20407=VECTOR('',#70131,10.);
#20408=VECTOR('',#70132,10.);
#20409=VECTOR('',#70133,10.);
#20410=VECTOR('',#70136,10.);
#20411=VECTOR('',#70137,10.);
#20412=VECTOR('',#70138,10.);
#20413=VECTOR('',#70139,10.);
#20414=VECTOR('',#70146,10.);
#20415=VECTOR('',#70151,10.);
#20416=VECTOR('',#70152,10.);
#20417=VECTOR('',#70153,10.);
#20418=VECTOR('',#70156,10.);
#20419=VECTOR('',#70157,10.);
#20420=VECTOR('',#70158,10.);
#20421=VECTOR('',#70159,10.);
#20422=VECTOR('',#70166,10.);
#20423=VECTOR('',#70171,10.);
#20424=VECTOR('',#70172,10.);
#20425=VECTOR('',#70173,10.);
#20426=VECTOR('',#70176,10.);
#20427=VECTOR('',#70177,10.);
#20428=VECTOR('',#70178,10.);
#20429=VECTOR('',#70179,10.);
#20430=VECTOR('',#70186,10.);
#20431=VECTOR('',#70191,10.);
#20432=VECTOR('',#70192,10.);
#20433=VECTOR('',#70193,10.);
#20434=VECTOR('',#70196,10.);
#20435=VECTOR('',#70197,10.);
#20436=VECTOR('',#70198,10.);
#20437=VECTOR('',#70199,10.);
#20438=VECTOR('',#70206,10.);
#20439=VECTOR('',#70211,10.);
#20440=VECTOR('',#70212,10.);
#20441=VECTOR('',#70213,10.);
#20442=VECTOR('',#70216,10.);
#20443=VECTOR('',#70217,10.);
#20444=VECTOR('',#70218,10.);
#20445=VECTOR('',#70219,10.);
#20446=VECTOR('',#70226,10.);
#20447=VECTOR('',#70231,10.);
#20448=VECTOR('',#70232,10.);
#20449=VECTOR('',#70233,10.);
#20450=VECTOR('',#70236,10.);
#20451=VECTOR('',#70237,10.);
#20452=VECTOR('',#70238,10.);
#20453=VECTOR('',#70239,10.);
#20454=VECTOR('',#70246,10.);
#20455=VECTOR('',#70251,10.);
#20456=VECTOR('',#70252,10.);
#20457=VECTOR('',#70253,10.);
#20458=VECTOR('',#70256,10.);
#20459=VECTOR('',#70257,10.);
#20460=VECTOR('',#70258,10.);
#20461=VECTOR('',#70259,10.);
#20462=VECTOR('',#70266,10.);
#20463=VECTOR('',#70271,10.);
#20464=VECTOR('',#70272,10.);
#20465=VECTOR('',#70273,10.);
#20466=VECTOR('',#70276,10.);
#20467=VECTOR('',#70277,10.);
#20468=VECTOR('',#70278,10.);
#20469=VECTOR('',#70279,10.);
#20470=VECTOR('',#70286,10.);
#20471=VECTOR('',#70291,10.);
#20472=VECTOR('',#70292,10.);
#20473=VECTOR('',#70293,10.);
#20474=VECTOR('',#70296,10.);
#20475=VECTOR('',#70297,10.);
#20476=VECTOR('',#70298,10.);
#20477=VECTOR('',#70299,10.);
#20478=VECTOR('',#70306,10.);
#20479=VECTOR('',#70311,10.);
#20480=VECTOR('',#70312,10.);
#20481=VECTOR('',#70313,10.);
#20482=VECTOR('',#70316,10.);
#20483=VECTOR('',#70317,10.);
#20484=VECTOR('',#70318,10.);
#20485=VECTOR('',#70319,10.);
#20486=VECTOR('',#70326,10.);
#20487=VECTOR('',#70331,10.);
#20488=VECTOR('',#70332,10.);
#20489=VECTOR('',#70333,10.);
#20490=VECTOR('',#70336,10.);
#20491=VECTOR('',#70337,10.);
#20492=VECTOR('',#70338,10.);
#20493=VECTOR('',#70339,10.);
#20494=VECTOR('',#70346,10.);
#20495=VECTOR('',#70351,10.);
#20496=VECTOR('',#70352,10.);
#20497=VECTOR('',#70353,10.);
#20498=VECTOR('',#70356,10.);
#20499=VECTOR('',#70357,10.);
#20500=VECTOR('',#70358,10.);
#20501=VECTOR('',#70359,10.);
#20502=VECTOR('',#70366,10.);
#20503=VECTOR('',#70371,10.);
#20504=VECTOR('',#70372,10.);
#20505=VECTOR('',#70373,10.);
#20506=VECTOR('',#70376,10.);
#20507=VECTOR('',#70377,10.);
#20508=VECTOR('',#70378,10.);
#20509=VECTOR('',#70379,10.);
#20510=VECTOR('',#70386,10.);
#20511=VECTOR('',#70391,10.);
#20512=VECTOR('',#70392,10.);
#20513=VECTOR('',#70393,10.);
#20514=VECTOR('',#70396,10.);
#20515=VECTOR('',#70397,10.);
#20516=VECTOR('',#70398,10.);
#20517=VECTOR('',#70399,10.);
#20518=VECTOR('',#70406,10.);
#20519=VECTOR('',#70411,10.);
#20520=VECTOR('',#70412,10.);
#20521=VECTOR('',#70413,10.);
#20522=VECTOR('',#70414,10.);
#20523=VECTOR('',#70421,10.);
#20524=VECTOR('',#70422,10.);
#20525=VECTOR('',#70425,10.);
#20526=VECTOR('',#70426,10.);
#20527=VECTOR('',#70433,2.5);
#20528=VECTOR('',#70446,4.49999999999999);
#20529=VECTOR('',#70451,4.34999999999999);
#24340=B_SPLINE_CURVE_WITH_KNOTS('',3,(#92665,#92666,#92667,#92668,#92669,
#92670,#92671,#92672,#92673,#92674),.UNSPECIFIED.,.F.,.F.,(4,2,2,2,4),(0.15884064059446,
0.198548710500137,0.238256780405813,0.277969030797367,0.317681281188921),
 .UNSPECIFIED.);
#24341=B_SPLINE_CURVE_WITH_KNOTS('',3,(#92676,#92677,#92678,#92679,#92680,
#92681,#92682,#92683,#92684,#92685,#92686,#92687,#92688,#92689,#92690,#92691,
#92692,#92693,#92694),.UNSPECIFIED.,.F.,.F.,(4,2,2,2,3,2,2,2,4),(0.476521921783381,
0.516229991689058,0.555938061594734,0.595650311986288,0.635362562377842,
0.675074812769396,0.71478706316095,0.754495133066626,0.794203202972302),
 .UNSPECIFIED.);
#24342=B_SPLINE_CURVE_WITH_KNOTS('',3,(#92695,#92696,#92697,#92698,#92699,
#92700,#92701,#92702,#92703,#92704),.UNSPECIFIED.,.F.,.F.,(4,2,2,2,4),(0.317681281188921,
0.357393531580475,0.397105781972029,0.436813851877705,0.476521921783381),
 .UNSPECIFIED.);
#24343=B_SPLINE_CURVE_WITH_KNOTS('',3,(#92709,#92710,#92711,#92712,#92713,
#92714,#92715,#92716,#92717,#92718),.UNSPECIFIED.,.F.,.F.,(4,2,2,2,4),(0.0861737376724399,
0.1203210472132,0.160394592890574,0.200468138567948,0.234615448108708),
 .UNSPECIFIED.);
#24344=B_SPLINE_CURVE_WITH_KNOTS('',3,(#92720,#92721,#92722,#92723,#92724,
#92725,#92726,#92727,#92728,#92729),.UNSPECIFIED.,.F.,.F.,(4,2,2,2,4),(0.406962923453589,
0.441110232994348,0.481183778671723,0.521257324349097,0.555404633889854),
 .UNSPECIFIED.);
#27911=VERTEX_POINT('',#92658);
#27912=VERTEX_POINT('',#92659);
#27913=VERTEX_POINT('',#92663);
#27914=VERTEX_POINT('',#92664);
#27915=VERTEX_POINT('',#92675);
#27916=VERTEX_POINT('',#92705);
#27917=VERTEX_POINT('',#92707);
#27918=VERTEX_POINT('',#92719);
#27919=VERTEX_POINT('',#92734);
#27920=VERTEX_POINT('',#92735);
#27921=VERTEX_POINT('',#92737);
#27922=VERTEX_POINT('',#92739);
#27923=VERTEX_POINT('',#92743);
#27924=VERTEX_POINT('',#92744);
#27925=VERTEX_POINT('',#92746);
#27926=VERTEX_POINT('',#92748);
#27927=VERTEX_POINT('',#92821);
#27928=VERTEX_POINT('',#92857);
#27929=VERTEX_POINT('',#92895);
#27930=VERTEX_POINT('',#92897);
#27931=VERTEX_POINT('',#93043);
#27932=VERTEX_POINT('',#93045);
#27933=VERTEX_POINT('',#93047);
#27934=VERTEX_POINT('',#93049);
#27935=VERTEX_POINT('',#93051);
#27936=VERTEX_POINT('',#93053);
#27937=VERTEX_POINT('',#93055);
#27938=VERTEX_POINT('',#93057);
#27939=VERTEX_POINT('',#93059);
#27940=VERTEX_POINT('',#93061);
#27941=VERTEX_POINT('',#93063);
#27942=VERTEX_POINT('',#93065);
#27943=VERTEX_POINT('',#93068);
#27944=VERTEX_POINT('',#93070);
#27945=VERTEX_POINT('',#93072);
#27946=VERTEX_POINT('',#93074);
#27947=VERTEX_POINT('',#93076);
#27948=VERTEX_POINT('',#93078);
#27949=VERTEX_POINT('',#93080);
#27950=VERTEX_POINT('',#93082);
#27951=VERTEX_POINT('',#93084);
#27952=VERTEX_POINT('',#93086);
#27953=VERTEX_POINT('',#93088);
#27954=VERTEX_POINT('',#93090);
#27955=VERTEX_POINT('',#93092);
#27956=VERTEX_POINT('',#93094);
#27957=VERTEX_POINT('',#93096);
#27958=VERTEX_POINT('',#93098);
#27959=VERTEX_POINT('',#93100);
#27960=VERTEX_POINT('',#93102);
#27961=VERTEX_POINT('',#93104);
#27962=VERTEX_POINT('',#93106);
#27963=VERTEX_POINT('',#93108);
#27964=VERTEX_POINT('',#93110);
#27965=VERTEX_POINT('',#93112);
#27966=VERTEX_POINT('',#93114);
#27967=VERTEX_POINT('',#93116);
#27968=VERTEX_POINT('',#93118);
#27969=VERTEX_POINT('',#93120);
#27970=VERTEX_POINT('',#93122);
#27971=VERTEX_POINT('',#93124);
#27972=VERTEX_POINT('',#93126);
#27973=VERTEX_POINT('',#93128);
#27974=VERTEX_POINT('',#93130);
#27975=VERTEX_POINT('',#93132);
#27976=VERTEX_POINT('',#93134);
#27977=VERTEX_POINT('',#93136);
#27978=VERTEX_POINT('',#93138);
#27979=VERTEX_POINT('',#93140);
#27980=VERTEX_POINT('',#93142);
#27981=VERTEX_POINT('',#93144);
#27982=VERTEX_POINT('',#93146);
#27983=VERTEX_POINT('',#93148);
#27984=VERTEX_POINT('',#93150);
#27985=VERTEX_POINT('',#93152);
#27986=VERTEX_POINT('',#93154);
#27987=VERTEX_POINT('',#93156);
#27988=VERTEX_POINT('',#93158);
#27989=VERTEX_POINT('',#93160);
#27990=VERTEX_POINT('',#93162);
#27991=VERTEX_POINT('',#93164);
#27992=VERTEX_POINT('',#93166);
#27993=VERTEX_POINT('',#93170);
#27994=VERTEX_POINT('',#93172);
#27995=VERTEX_POINT('',#93176);
#27996=VERTEX_POINT('',#93178);
#27997=VERTEX_POINT('',#93251);
#27998=VERTEX_POINT('',#93287);
#27999=VERTEX_POINT('',#93325);
#28000=VERTEX_POINT('',#93327);
#28001=VERTEX_POINT('',#93472);
#28002=VERTEX_POINT('',#93474);
#28003=VERTEX_POINT('',#93478);
#28004=VERTEX_POINT('',#93480);
#28005=VERTEX_POINT('',#93553);
#28006=VERTEX_POINT('',#93589);
#28007=VERTEX_POINT('',#93627);
#28008=VERTEX_POINT('',#93629);
#28009=VERTEX_POINT('',#93774);
#28010=VERTEX_POINT('',#93776);
#28011=VERTEX_POINT('',#93780);
#28012=VERTEX_POINT('',#93782);
#28013=VERTEX_POINT('',#93855);
#28014=VERTEX_POINT('',#93891);
#28015=VERTEX_POINT('',#93929);
#28016=VERTEX_POINT('',#93931);
#28017=VERTEX_POINT('',#94076);
#28018=VERTEX_POINT('',#94078);
#28019=VERTEX_POINT('',#94082);
#28020=VERTEX_POINT('',#94084);
#28021=VERTEX_POINT('',#94157);
#28022=VERTEX_POINT('',#94193);
#28023=VERTEX_POINT('',#94231);
#28024=VERTEX_POINT('',#94233);
#28025=VERTEX_POINT('',#94378);
#28026=VERTEX_POINT('',#94380);
#28027=VERTEX_POINT('',#94384);
#28028=VERTEX_POINT('',#94386);
#28029=VERTEX_POINT('',#94459);
#28030=VERTEX_POINT('',#94495);
#28031=VERTEX_POINT('',#94533);
#28032=VERTEX_POINT('',#94535);
#28033=VERTEX_POINT('',#94680);
#28034=VERTEX_POINT('',#94682);
#28035=VERTEX_POINT('',#94686);
#28036=VERTEX_POINT('',#94688);
#28037=VERTEX_POINT('',#94761);
#28038=VERTEX_POINT('',#94797);
#28039=VERTEX_POINT('',#94835);
#28040=VERTEX_POINT('',#94837);
#28041=VERTEX_POINT('',#94982);
#28042=VERTEX_POINT('',#94984);
#28043=VERTEX_POINT('',#94988);
#28044=VERTEX_POINT('',#94990);
#28045=VERTEX_POINT('',#95063);
#28046=VERTEX_POINT('',#95099);
#28047=VERTEX_POINT('',#95137);
#28048=VERTEX_POINT('',#95139);
#28049=VERTEX_POINT('',#95284);
#28050=VERTEX_POINT('',#95286);
#28051=VERTEX_POINT('',#95290);
#28052=VERTEX_POINT('',#95292);
#28053=VERTEX_POINT('',#95365);
#28054=VERTEX_POINT('',#95401);
#28055=VERTEX_POINT('',#95439);
#28056=VERTEX_POINT('',#95441);
#28057=VERTEX_POINT('',#95586);
#28058=VERTEX_POINT('',#95588);
#28059=VERTEX_POINT('',#95592);
#28060=VERTEX_POINT('',#95594);
#28061=VERTEX_POINT('',#95667);
#28062=VERTEX_POINT('',#95703);
#28063=VERTEX_POINT('',#95741);
#28064=VERTEX_POINT('',#95743);
#28065=VERTEX_POINT('',#95888);
#28066=VERTEX_POINT('',#95890);
#28067=VERTEX_POINT('',#95894);
#28068=VERTEX_POINT('',#95896);
#28069=VERTEX_POINT('',#95969);
#28070=VERTEX_POINT('',#96005);
#28071=VERTEX_POINT('',#96043);
#28072=VERTEX_POINT('',#96045);
#28073=VERTEX_POINT('',#96190);
#28074=VERTEX_POINT('',#96192);
#28075=VERTEX_POINT('',#96196);
#28076=VERTEX_POINT('',#96198);
#28077=VERTEX_POINT('',#96271);
#28078=VERTEX_POINT('',#96307);
#28079=VERTEX_POINT('',#96345);
#28080=VERTEX_POINT('',#96347);
#28081=VERTEX_POINT('',#96492);
#28082=VERTEX_POINT('',#96494);
#28083=VERTEX_POINT('',#96498);
#28084=VERTEX_POINT('',#96500);
#28085=VERTEX_POINT('',#96573);
#28086=VERTEX_POINT('',#96609);
#28087=VERTEX_POINT('',#96647);
#28088=VERTEX_POINT('',#96649);
#28089=VERTEX_POINT('',#96794);
#28090=VERTEX_POINT('',#96796);
#28091=VERTEX_POINT('',#96800);
#28092=VERTEX_POINT('',#96802);
#28093=VERTEX_POINT('',#96875);
#28094=VERTEX_POINT('',#96911);
#28095=VERTEX_POINT('',#96949);
#28096=VERTEX_POINT('',#96951);
#28097=VERTEX_POINT('',#97096);
#28098=VERTEX_POINT('',#97098);
#28099=VERTEX_POINT('',#97102);
#28100=VERTEX_POINT('',#97104);
#28101=VERTEX_POINT('',#97177);
#28102=VERTEX_POINT('',#97213);
#28103=VERTEX_POINT('',#97251);
#28104=VERTEX_POINT('',#97253);
#28105=VERTEX_POINT('',#97398);
#28106=VERTEX_POINT('',#97400);
#28107=VERTEX_POINT('',#97473);
#28108=VERTEX_POINT('',#97509);
#28109=VERTEX_POINT('',#97547);
#28110=VERTEX_POINT('',#97549);
#28111=VERTEX_POINT('',#97622);
#28112=VERTEX_POINT('',#97658);
#28113=VERTEX_POINT('',#97700);
#28114=VERTEX_POINT('',#97702);
#28115=VERTEX_POINT('',#97707);
#28116=VERTEX_POINT('',#97710);
#28117=VERTEX_POINT('',#97714);
#35326=EDGE_CURVE('',#27911,#27912,#14329,.T.);
#35327=EDGE_CURVE('',#27912,#27911,#1063,.T.);
#35328=EDGE_CURVE('',#27913,#27914,#24340,.T.);
#35329=EDGE_CURVE('',#27915,#27913,#24341,.T.);
#35330=EDGE_CURVE('',#27914,#27915,#24342,.T.);
#35331=EDGE_CURVE('',#27914,#27916,#14330,.T.);
#35332=EDGE_CURVE('',#27916,#27917,#1064,.T.);
#35333=EDGE_CURVE('',#27912,#27917,#24343,.T.);
#35334=EDGE_CURVE('',#27918,#27911,#24344,.T.);
#35335=EDGE_CURVE('',#27918,#27916,#1065,.T.);
#35336=EDGE_CURVE('',#27917,#27918,#14331,.T.);
#35337=EDGE_CURVE('',#27919,#27920,#14332,.T.);
#35338=EDGE_CURVE('',#27921,#27919,#14333,.T.);
#35339=EDGE_CURVE('',#27921,#27922,#14334,.T.);
#35340=EDGE_CURVE('',#27920,#27922,#14335,.T.);
#35341=EDGE_CURVE('',#27923,#27924,#14336,.T.);
#35342=EDGE_CURVE('',#27925,#27923,#14337,.T.);
#35343=EDGE_CURVE('',#27926,#27925,#14338,.T.);
#35344=EDGE_CURVE('',#27924,#27926,#14339,.T.);
#35345=EDGE_CURVE('',#27926,#27927,#147,.T.);
#35346=EDGE_CURVE('',#27928,#27925,#148,.T.);
#35347=EDGE_CURVE('',#27927,#27928,#14340,.T.);
#35348=EDGE_CURVE('',#27927,#27929,#1066,.T.);
#35349=EDGE_CURVE('',#27930,#27928,#1067,.T.);
#35350=EDGE_CURVE('',#27929,#27930,#14341,.T.);
#35351=EDGE_CURVE('',#27921,#27929,#149,.T.);
#35352=EDGE_CURVE('',#27922,#27930,#150,.T.);
#35353=EDGE_CURVE('',#27924,#27919,#1068,.T.);
#35354=EDGE_CURVE('',#27931,#27931,#1069,.T.);
#35355=EDGE_CURVE('',#27931,#27932,#14342,.T.);
#35356=EDGE_CURVE('',#27932,#27933,#1070,.T.);
#35357=EDGE_CURVE('',#27933,#27934,#14343,.T.);
#35358=EDGE_CURVE('',#27934,#27935,#1071,.T.);
#35359=EDGE_CURVE('',#27935,#27936,#14344,.T.);
#35360=EDGE_CURVE('',#27936,#27937,#1072,.T.);
#35361=EDGE_CURVE('',#27937,#27938,#14345,.T.);
#35362=EDGE_CURVE('',#27938,#27939,#1073,.T.);
#35363=EDGE_CURVE('',#27939,#27940,#14346,.T.);
#35364=EDGE_CURVE('',#27940,#27941,#1074,.T.);
#35365=EDGE_CURVE('',#27941,#27942,#14347,.T.);
#35366=EDGE_CURVE('',#27942,#27923,#1075,.T.);
#35367=EDGE_CURVE('',#27920,#27943,#1076,.T.);
#35368=EDGE_CURVE('',#27943,#27944,#14348,.T.);
#35369=EDGE_CURVE('',#27944,#27945,#1077,.T.);
#35370=EDGE_CURVE('',#27945,#27946,#14349,.T.);
#35371=EDGE_CURVE('',#27946,#27947,#1078,.T.);
#35372=EDGE_CURVE('',#27947,#27948,#14350,.T.);
#35373=EDGE_CURVE('',#27948,#27949,#1079,.T.);
#35374=EDGE_CURVE('',#27949,#27950,#14351,.T.);
#35375=EDGE_CURVE('',#27950,#27951,#1080,.T.);
#35376=EDGE_CURVE('',#27951,#27952,#14352,.T.);
#35377=EDGE_CURVE('',#27952,#27953,#1081,.T.);
#35378=EDGE_CURVE('',#27953,#27954,#14353,.T.);
#35379=EDGE_CURVE('',#27954,#27955,#1082,.T.);
#35380=EDGE_CURVE('',#27955,#27956,#14354,.T.);
#35381=EDGE_CURVE('',#27956,#27957,#1083,.T.);
#35382=EDGE_CURVE('',#27957,#27958,#14355,.T.);
#35383=EDGE_CURVE('',#27958,#27959,#1084,.T.);
#35384=EDGE_CURVE('',#27959,#27960,#14356,.T.);
#35385=EDGE_CURVE('',#27960,#27961,#1085,.T.);
#35386=EDGE_CURVE('',#27961,#27962,#14357,.T.);
#35387=EDGE_CURVE('',#27962,#27963,#1086,.T.);
#35388=EDGE_CURVE('',#27963,#27964,#14358,.T.);
#35389=EDGE_CURVE('',#27964,#27965,#1087,.T.);
#35390=EDGE_CURVE('',#27965,#27966,#14359,.T.);
#35391=EDGE_CURVE('',#27966,#27967,#1088,.T.);
#35392=EDGE_CURVE('',#27967,#27968,#14360,.T.);
#35393=EDGE_CURVE('',#27968,#27969,#1089,.T.);
#35394=EDGE_CURVE('',#27969,#27970,#14361,.T.);
#35395=EDGE_CURVE('',#27970,#27971,#1090,.T.);
#35396=EDGE_CURVE('',#27971,#27972,#14362,.T.);
#35397=EDGE_CURVE('',#27972,#27973,#1091,.T.);
#35398=EDGE_CURVE('',#27973,#27974,#14363,.T.);
#35399=EDGE_CURVE('',#27974,#27975,#1092,.T.);
#35400=EDGE_CURVE('',#27975,#27976,#14364,.T.);
#35401=EDGE_CURVE('',#27976,#27977,#1093,.T.);
#35402=EDGE_CURVE('',#27977,#27978,#14365,.T.);
#35403=EDGE_CURVE('',#27978,#27979,#1094,.T.);
#35404=EDGE_CURVE('',#27979,#27980,#14366,.T.);
#35405=EDGE_CURVE('',#27980,#27981,#1095,.T.);
#35406=EDGE_CURVE('',#27981,#27982,#14367,.T.);
#35407=EDGE_CURVE('',#27982,#27983,#1096,.T.);
#35408=EDGE_CURVE('',#27983,#27984,#14368,.T.);
#35409=EDGE_CURVE('',#27984,#27985,#1097,.T.);
#35410=EDGE_CURVE('',#27985,#27986,#14369,.T.);
#35411=EDGE_CURVE('',#27986,#27987,#1098,.T.);
#35412=EDGE_CURVE('',#27987,#27988,#14370,.T.);
#35413=EDGE_CURVE('',#27988,#27989,#1099,.T.);
#35414=EDGE_CURVE('',#27989,#27990,#14371,.T.);
#35415=EDGE_CURVE('',#27990,#27991,#1100,.T.);
#35416=EDGE_CURVE('',#27991,#27992,#14372,.T.);
#35417=EDGE_CURVE('',#27992,#27932,#1101,.T.);
#35418=EDGE_CURVE('',#27993,#27941,#14373,.T.);
#35419=EDGE_CURVE('',#27993,#27994,#14374,.T.);
#35420=EDGE_CURVE('',#27942,#27994,#14375,.T.);
#35421=EDGE_CURVE('',#27995,#27939,#14376,.T.);
#35422=EDGE_CURVE('',#27996,#27995,#14377,.T.);
#35423=EDGE_CURVE('',#27940,#27996,#14378,.T.);
#35424=EDGE_CURVE('',#27996,#27997,#151,.T.);
#35425=EDGE_CURVE('',#27998,#27995,#152,.T.);
#35426=EDGE_CURVE('',#27997,#27998,#14379,.T.);
#35427=EDGE_CURVE('',#27997,#27999,#1102,.T.);
#35428=EDGE_CURVE('',#28000,#27998,#1103,.T.);
#35429=EDGE_CURVE('',#27999,#28000,#14380,.T.);
#35430=EDGE_CURVE('',#27993,#27999,#153,.T.);
#35431=EDGE_CURVE('',#27994,#28000,#154,.T.);
#35432=EDGE_CURVE('',#28001,#27937,#14381,.T.);
#35433=EDGE_CURVE('',#28001,#28002,#14382,.T.);
#35434=EDGE_CURVE('',#27938,#28002,#14383,.T.);
#35435=EDGE_CURVE('',#28003,#27935,#14384,.T.);
#35436=EDGE_CURVE('',#28004,#28003,#14385,.T.);
#35437=EDGE_CURVE('',#27936,#28004,#14386,.T.);
#35438=EDGE_CURVE('',#28004,#28005,#155,.T.);
#35439=EDGE_CURVE('',#28006,#28003,#156,.T.);
#35440=EDGE_CURVE('',#28005,#28006,#14387,.T.);
#35441=EDGE_CURVE('',#28005,#28007,#1104,.T.);
#35442=EDGE_CURVE('',#28008,#28006,#1105,.T.);
#35443=EDGE_CURVE('',#28007,#28008,#14388,.T.);
#35444=EDGE_CURVE('',#28001,#28007,#157,.T.);
#35445=EDGE_CURVE('',#28002,#28008,#158,.T.);
#35446=EDGE_CURVE('',#28009,#27933,#14389,.T.);
#35447=EDGE_CURVE('',#28009,#28010,#14390,.T.);
#35448=EDGE_CURVE('',#27934,#28010,#14391,.T.);
#35449=EDGE_CURVE('',#28011,#27991,#14392,.T.);
#35450=EDGE_CURVE('',#28012,#28011,#14393,.T.);
#35451=EDGE_CURVE('',#27992,#28012,#14394,.T.);
#35452=EDGE_CURVE('',#28012,#28013,#159,.T.);
#35453=EDGE_CURVE('',#28014,#28011,#160,.T.);
#35454=EDGE_CURVE('',#28013,#28014,#14395,.T.);
#35455=EDGE_CURVE('',#28013,#28015,#1106,.T.);
#35456=EDGE_CURVE('',#28016,#28014,#1107,.T.);
#35457=EDGE_CURVE('',#28015,#28016,#14396,.T.);
#35458=EDGE_CURVE('',#28009,#28015,#161,.T.);
#35459=EDGE_CURVE('',#28010,#28016,#162,.T.);
#35460=EDGE_CURVE('',#28017,#27989,#14397,.T.);
#35461=EDGE_CURVE('',#28017,#28018,#14398,.T.);
#35462=EDGE_CURVE('',#27990,#28018,#14399,.T.);
#35463=EDGE_CURVE('',#28019,#27987,#14400,.T.);
#35464=EDGE_CURVE('',#28020,#28019,#14401,.T.);
#35465=EDGE_CURVE('',#27988,#28020,#14402,.T.);
#35466=EDGE_CURVE('',#28020,#28021,#163,.T.);
#35467=EDGE_CURVE('',#28022,#28019,#164,.T.);
#35468=EDGE_CURVE('',#28021,#28022,#14403,.T.);
#35469=EDGE_CURVE('',#28021,#28023,#1108,.T.);
#35470=EDGE_CURVE('',#28024,#28022,#1109,.T.);
#35471=EDGE_CURVE('',#28023,#28024,#14404,.T.);
#35472=EDGE_CURVE('',#28017,#28023,#165,.T.);
#35473=EDGE_CURVE('',#28018,#28024,#166,.T.);
#35474=EDGE_CURVE('',#28025,#27985,#14405,.T.);
#35475=EDGE_CURVE('',#28025,#28026,#14406,.T.);
#35476=EDGE_CURVE('',#27986,#28026,#14407,.T.);
#35477=EDGE_CURVE('',#28027,#27983,#14408,.T.);
#35478=EDGE_CURVE('',#28028,#28027,#14409,.T.);
#35479=EDGE_CURVE('',#27984,#28028,#14410,.T.);
#35480=EDGE_CURVE('',#28028,#28029,#167,.T.);
#35481=EDGE_CURVE('',#28030,#28027,#168,.T.);
#35482=EDGE_CURVE('',#28029,#28030,#14411,.T.);
#35483=EDGE_CURVE('',#28029,#28031,#1110,.T.);
#35484=EDGE_CURVE('',#28032,#28030,#1111,.T.);
#35485=EDGE_CURVE('',#28031,#28032,#14412,.T.);
#35486=EDGE_CURVE('',#28025,#28031,#169,.T.);
#35487=EDGE_CURVE('',#28026,#28032,#170,.T.);
#35488=EDGE_CURVE('',#28033,#27981,#14413,.T.);
#35489=EDGE_CURVE('',#28033,#28034,#14414,.T.);
#35490=EDGE_CURVE('',#27982,#28034,#14415,.T.);
#35491=EDGE_CURVE('',#28035,#27979,#14416,.T.);
#35492=EDGE_CURVE('',#28036,#28035,#14417,.T.);
#35493=EDGE_CURVE('',#27980,#28036,#14418,.T.);
#35494=EDGE_CURVE('',#28036,#28037,#171,.T.);
#35495=EDGE_CURVE('',#28038,#28035,#172,.T.);
#35496=EDGE_CURVE('',#28037,#28038,#14419,.T.);
#35497=EDGE_CURVE('',#28037,#28039,#1112,.T.);
#35498=EDGE_CURVE('',#28040,#28038,#1113,.T.);
#35499=EDGE_CURVE('',#28039,#28040,#14420,.T.);
#35500=EDGE_CURVE('',#28033,#28039,#173,.T.);
#35501=EDGE_CURVE('',#28034,#28040,#174,.T.);
#35502=EDGE_CURVE('',#28041,#27977,#14421,.T.);
#35503=EDGE_CURVE('',#28041,#28042,#14422,.T.);
#35504=EDGE_CURVE('',#27978,#28042,#14423,.T.);
#35505=EDGE_CURVE('',#28043,#27975,#14424,.T.);
#35506=EDGE_CURVE('',#28044,#28043,#14425,.T.);
#35507=EDGE_CURVE('',#27976,#28044,#14426,.T.);
#35508=EDGE_CURVE('',#28044,#28045,#175,.T.);
#35509=EDGE_CURVE('',#28046,#28043,#176,.T.);
#35510=EDGE_CURVE('',#28045,#28046,#14427,.T.);
#35511=EDGE_CURVE('',#28045,#28047,#1114,.T.);
#35512=EDGE_CURVE('',#28048,#28046,#1115,.T.);
#35513=EDGE_CURVE('',#28047,#28048,#14428,.T.);
#35514=EDGE_CURVE('',#28041,#28047,#177,.T.);
#35515=EDGE_CURVE('',#28042,#28048,#178,.T.);
#35516=EDGE_CURVE('',#28049,#27973,#14429,.T.);
#35517=EDGE_CURVE('',#28049,#28050,#14430,.T.);
#35518=EDGE_CURVE('',#27974,#28050,#14431,.T.);
#35519=EDGE_CURVE('',#28051,#27971,#14432,.T.);
#35520=EDGE_CURVE('',#28052,#28051,#14433,.T.);
#35521=EDGE_CURVE('',#27972,#28052,#14434,.T.);
#35522=EDGE_CURVE('',#28052,#28053,#179,.T.);
#35523=EDGE_CURVE('',#28054,#28051,#180,.T.);
#35524=EDGE_CURVE('',#28053,#28054,#14435,.T.);
#35525=EDGE_CURVE('',#28053,#28055,#1116,.T.);
#35526=EDGE_CURVE('',#28056,#28054,#1117,.T.);
#35527=EDGE_CURVE('',#28055,#28056,#14436,.T.);
#35528=EDGE_CURVE('',#28049,#28055,#181,.T.);
#35529=EDGE_CURVE('',#28050,#28056,#182,.T.);
#35530=EDGE_CURVE('',#28057,#27969,#14437,.T.);
#35531=EDGE_CURVE('',#28057,#28058,#14438,.T.);
#35532=EDGE_CURVE('',#27970,#28058,#14439,.T.);
#35533=EDGE_CURVE('',#28059,#27967,#14440,.T.);
#35534=EDGE_CURVE('',#28060,#28059,#14441,.T.);
#35535=EDGE_CURVE('',#27968,#28060,#14442,.T.);
#35536=EDGE_CURVE('',#28060,#28061,#183,.T.);
#35537=EDGE_CURVE('',#28062,#28059,#184,.T.);
#35538=EDGE_CURVE('',#28061,#28062,#14443,.T.);
#35539=EDGE_CURVE('',#28061,#28063,#1118,.T.);
#35540=EDGE_CURVE('',#28064,#28062,#1119,.T.);
#35541=EDGE_CURVE('',#28063,#28064,#14444,.T.);
#35542=EDGE_CURVE('',#28057,#28063,#185,.T.);
#35543=EDGE_CURVE('',#28058,#28064,#186,.T.);
#35544=EDGE_CURVE('',#28065,#27965,#14445,.T.);
#35545=EDGE_CURVE('',#28065,#28066,#14446,.T.);
#35546=EDGE_CURVE('',#27966,#28066,#14447,.T.);
#35547=EDGE_CURVE('',#28067,#27963,#14448,.T.);
#35548=EDGE_CURVE('',#28068,#28067,#14449,.T.);
#35549=EDGE_CURVE('',#27964,#28068,#14450,.T.);
#35550=EDGE_CURVE('',#28068,#28069,#187,.T.);
#35551=EDGE_CURVE('',#28070,#28067,#188,.T.);
#35552=EDGE_CURVE('',#28069,#28070,#14451,.T.);
#35553=EDGE_CURVE('',#28069,#28071,#1120,.T.);
#35554=EDGE_CURVE('',#28072,#28070,#1121,.T.);
#35555=EDGE_CURVE('',#28071,#28072,#14452,.T.);
#35556=EDGE_CURVE('',#28065,#28071,#189,.T.);
#35557=EDGE_CURVE('',#28066,#28072,#190,.T.);
#35558=EDGE_CURVE('',#28073,#27961,#14453,.T.);
#35559=EDGE_CURVE('',#28073,#28074,#14454,.T.);
#35560=EDGE_CURVE('',#27962,#28074,#14455,.T.);
#35561=EDGE_CURVE('',#28075,#27959,#14456,.T.);
#35562=EDGE_CURVE('',#28076,#28075,#14457,.T.);
#35563=EDGE_CURVE('',#27960,#28076,#14458,.T.);
#35564=EDGE_CURVE('',#28076,#28077,#191,.T.);
#35565=EDGE_CURVE('',#28078,#28075,#192,.T.);
#35566=EDGE_CURVE('',#28077,#28078,#14459,.T.);
#35567=EDGE_CURVE('',#28077,#28079,#1122,.T.);
#35568=EDGE_CURVE('',#28080,#28078,#1123,.T.);
#35569=EDGE_CURVE('',#28079,#28080,#14460,.T.);
#35570=EDGE_CURVE('',#28073,#28079,#193,.T.);
#35571=EDGE_CURVE('',#28074,#28080,#194,.T.);
#35572=EDGE_CURVE('',#28081,#27957,#14461,.T.);
#35573=EDGE_CURVE('',#28081,#28082,#14462,.T.);
#35574=EDGE_CURVE('',#27958,#28082,#14463,.T.);
#35575=EDGE_CURVE('',#28083,#27955,#14464,.T.);
#35576=EDGE_CURVE('',#28084,#28083,#14465,.T.);
#35577=EDGE_CURVE('',#27956,#28084,#14466,.T.);
#35578=EDGE_CURVE('',#28084,#28085,#195,.T.);
#35579=EDGE_CURVE('',#28086,#28083,#196,.T.);
#35580=EDGE_CURVE('',#28085,#28086,#14467,.T.);
#35581=EDGE_CURVE('',#28085,#28087,#1124,.T.);
#35582=EDGE_CURVE('',#28088,#28086,#1125,.T.);
#35583=EDGE_CURVE('',#28087,#28088,#14468,.T.);
#35584=EDGE_CURVE('',#28081,#28087,#197,.T.);
#35585=EDGE_CURVE('',#28082,#28088,#198,.T.);
#35586=EDGE_CURVE('',#28089,#27953,#14469,.T.);
#35587=EDGE_CURVE('',#28089,#28090,#14470,.T.);
#35588=EDGE_CURVE('',#27954,#28090,#14471,.T.);
#35589=EDGE_CURVE('',#28091,#27951,#14472,.T.);
#35590=EDGE_CURVE('',#28092,#28091,#14473,.T.);
#35591=EDGE_CURVE('',#27952,#28092,#14474,.T.);
#35592=EDGE_CURVE('',#28092,#28093,#199,.T.);
#35593=EDGE_CURVE('',#28094,#28091,#200,.T.);
#35594=EDGE_CURVE('',#28093,#28094,#14475,.T.);
#35595=EDGE_CURVE('',#28093,#28095,#1126,.T.);
#35596=EDGE_CURVE('',#28096,#28094,#1127,.T.);
#35597=EDGE_CURVE('',#28095,#28096,#14476,.T.);
#35598=EDGE_CURVE('',#28089,#28095,#201,.T.);
#35599=EDGE_CURVE('',#28090,#28096,#202,.T.);
#35600=EDGE_CURVE('',#28097,#27949,#14477,.T.);
#35601=EDGE_CURVE('',#28097,#28098,#14478,.T.);
#35602=EDGE_CURVE('',#27950,#28098,#14479,.T.);
#35603=EDGE_CURVE('',#28099,#27947,#14480,.T.);
#35604=EDGE_CURVE('',#28100,#28099,#14481,.T.);
#35605=EDGE_CURVE('',#27948,#28100,#14482,.T.);
#35606=EDGE_CURVE('',#28100,#28101,#203,.T.);
#35607=EDGE_CURVE('',#28102,#28099,#204,.T.);
#35608=EDGE_CURVE('',#28101,#28102,#14483,.T.);
#35609=EDGE_CURVE('',#28101,#28103,#1128,.T.);
#35610=EDGE_CURVE('',#28104,#28102,#1129,.T.);
#35611=EDGE_CURVE('',#28103,#28104,#14484,.T.);
#35612=EDGE_CURVE('',#28097,#28103,#205,.T.);
#35613=EDGE_CURVE('',#28098,#28104,#206,.T.);
#35614=EDGE_CURVE('',#28105,#27943,#14485,.T.);
#35615=EDGE_CURVE('',#28106,#28105,#14486,.T.);
#35616=EDGE_CURVE('',#27944,#28106,#14487,.T.);
#35617=EDGE_CURVE('',#28106,#28107,#207,.T.);
#35618=EDGE_CURVE('',#28108,#28105,#208,.T.);
#35619=EDGE_CURVE('',#28107,#28108,#14488,.T.);
#35620=EDGE_CURVE('',#28107,#28109,#1130,.T.);
#35621=EDGE_CURVE('',#28110,#28108,#1131,.T.);
#35622=EDGE_CURVE('',#28109,#28110,#14489,.T.);
#35623=EDGE_CURVE('',#28111,#28109,#209,.T.);
#35624=EDGE_CURVE('',#28112,#28110,#210,.T.);
#35625=EDGE_CURVE('',#28111,#28112,#14490,.T.);
#35626=EDGE_CURVE('',#28111,#27945,#14491,.T.);
#35627=EDGE_CURVE('',#27946,#28112,#14492,.T.);
#35628=EDGE_CURVE('',#28113,#28113,#1132,.T.);
#35629=EDGE_CURVE('',#28113,#28114,#14493,.T.);
#35630=EDGE_CURVE('',#28114,#28114,#1133,.T.);
#35631=EDGE_CURVE('',#28115,#28115,#1134,.T.);
#35632=EDGE_CURVE('',#28116,#28116,#1135,.T.);
#35633=EDGE_CURVE('',#28116,#28115,#14494,.T.);
#35634=EDGE_CURVE('',#28117,#28117,#1136,.T.);
#35635=EDGE_CURVE('',#28117,#28116,#14495,.T.);
#48987=ORIENTED_EDGE('',*,*,#35326,.F.);
#48988=ORIENTED_EDGE('',*,*,#35327,.F.);
#48989=ORIENTED_EDGE('',*,*,#35328,.F.);
#48990=ORIENTED_EDGE('',*,*,#35329,.F.);
#48991=ORIENTED_EDGE('',*,*,#35330,.F.);
#48992=ORIENTED_EDGE('',*,*,#35331,.T.);
#48993=ORIENTED_EDGE('',*,*,#35332,.T.);
#48994=ORIENTED_EDGE('',*,*,#35333,.F.);
#48995=ORIENTED_EDGE('',*,*,#35327,.T.);
#48996=ORIENTED_EDGE('',*,*,#35334,.F.);
#48997=ORIENTED_EDGE('',*,*,#35335,.T.);
#48998=ORIENTED_EDGE('',*,*,#35331,.F.);
#48999=ORIENTED_EDGE('',*,*,#35336,.F.);
#49000=ORIENTED_EDGE('',*,*,#35332,.F.);
#49001=ORIENTED_EDGE('',*,*,#35335,.F.);
#49002=ORIENTED_EDGE('',*,*,#35337,.F.);
#49003=ORIENTED_EDGE('',*,*,#35338,.F.);
#49004=ORIENTED_EDGE('',*,*,#35339,.T.);
#49005=ORIENTED_EDGE('',*,*,#35340,.F.);
#49006=ORIENTED_EDGE('',*,*,#35341,.F.);
#49007=ORIENTED_EDGE('',*,*,#35342,.F.);
#49008=ORIENTED_EDGE('',*,*,#35343,.F.);
#49009=ORIENTED_EDGE('',*,*,#35344,.F.);
#49010=ORIENTED_EDGE('',*,*,#35345,.F.);
#49011=ORIENTED_EDGE('',*,*,#35343,.T.);
#49012=ORIENTED_EDGE('',*,*,#35346,.F.);
#49013=ORIENTED_EDGE('',*,*,#35347,.F.);
#49014=ORIENTED_EDGE('',*,*,#35348,.F.);
#49015=ORIENTED_EDGE('',*,*,#35347,.T.);
#49016=ORIENTED_EDGE('',*,*,#35349,.F.);
#49017=ORIENTED_EDGE('',*,*,#35350,.F.);
#49018=ORIENTED_EDGE('',*,*,#35351,.T.);
#49019=ORIENTED_EDGE('',*,*,#35350,.T.);
#49020=ORIENTED_EDGE('',*,*,#35352,.F.);
#49021=ORIENTED_EDGE('',*,*,#35339,.F.);
#49022=ORIENTED_EDGE('',*,*,#35353,.F.);
#49023=ORIENTED_EDGE('',*,*,#35344,.T.);
#49024=ORIENTED_EDGE('',*,*,#35345,.T.);
#49025=ORIENTED_EDGE('',*,*,#35348,.T.);
#49026=ORIENTED_EDGE('',*,*,#35351,.F.);
#49027=ORIENTED_EDGE('',*,*,#35338,.T.);
#49028=ORIENTED_EDGE('',*,*,#35354,.F.);
#49029=ORIENTED_EDGE('',*,*,#35355,.T.);
#49030=ORIENTED_EDGE('',*,*,#35356,.T.);
#49031=ORIENTED_EDGE('',*,*,#35357,.T.);
#49032=ORIENTED_EDGE('',*,*,#35358,.T.);
#49033=ORIENTED_EDGE('',*,*,#35359,.T.);
#49034=ORIENTED_EDGE('',*,*,#35360,.T.);
#49035=ORIENTED_EDGE('',*,*,#35361,.T.);
#49036=ORIENTED_EDGE('',*,*,#35362,.T.);
#49037=ORIENTED_EDGE('',*,*,#35363,.T.);
#49038=ORIENTED_EDGE('',*,*,#35364,.T.);
#49039=ORIENTED_EDGE('',*,*,#35365,.T.);
#49040=ORIENTED_EDGE('',*,*,#35366,.T.);
#49041=ORIENTED_EDGE('',*,*,#35341,.T.);
#49042=ORIENTED_EDGE('',*,*,#35353,.T.);
#49043=ORIENTED_EDGE('',*,*,#35337,.T.);
#49044=ORIENTED_EDGE('',*,*,#35367,.T.);
#49045=ORIENTED_EDGE('',*,*,#35368,.T.);
#49046=ORIENTED_EDGE('',*,*,#35369,.T.);
#49047=ORIENTED_EDGE('',*,*,#35370,.T.);
#49048=ORIENTED_EDGE('',*,*,#35371,.T.);
#49049=ORIENTED_EDGE('',*,*,#35372,.T.);
#49050=ORIENTED_EDGE('',*,*,#35373,.T.);
#49051=ORIENTED_EDGE('',*,*,#35374,.T.);
#49052=ORIENTED_EDGE('',*,*,#35375,.T.);
#49053=ORIENTED_EDGE('',*,*,#35376,.T.);
#49054=ORIENTED_EDGE('',*,*,#35377,.T.);
#49055=ORIENTED_EDGE('',*,*,#35378,.T.);
#49056=ORIENTED_EDGE('',*,*,#35379,.T.);
#49057=ORIENTED_EDGE('',*,*,#35380,.T.);
#49058=ORIENTED_EDGE('',*,*,#35381,.T.);
#49059=ORIENTED_EDGE('',*,*,#35382,.T.);
#49060=ORIENTED_EDGE('',*,*,#35383,.T.);
#49061=ORIENTED_EDGE('',*,*,#35384,.T.);
#49062=ORIENTED_EDGE('',*,*,#35385,.T.);
#49063=ORIENTED_EDGE('',*,*,#35386,.T.);
#49064=ORIENTED_EDGE('',*,*,#35387,.T.);
#49065=ORIENTED_EDGE('',*,*,#35388,.T.);
#49066=ORIENTED_EDGE('',*,*,#35389,.T.);
#49067=ORIENTED_EDGE('',*,*,#35390,.T.);
#49068=ORIENTED_EDGE('',*,*,#35391,.T.);
#49069=ORIENTED_EDGE('',*,*,#35392,.T.);
#49070=ORIENTED_EDGE('',*,*,#35393,.T.);
#49071=ORIENTED_EDGE('',*,*,#35394,.T.);
#49072=ORIENTED_EDGE('',*,*,#35395,.T.);
#49073=ORIENTED_EDGE('',*,*,#35396,.T.);
#49074=ORIENTED_EDGE('',*,*,#35397,.T.);
#49075=ORIENTED_EDGE('',*,*,#35398,.T.);
#49076=ORIENTED_EDGE('',*,*,#35399,.T.);
#49077=ORIENTED_EDGE('',*,*,#35400,.T.);
#49078=ORIENTED_EDGE('',*,*,#35401,.T.);
#49079=ORIENTED_EDGE('',*,*,#35402,.T.);
#49080=ORIENTED_EDGE('',*,*,#35403,.T.);
#49081=ORIENTED_EDGE('',*,*,#35404,.T.);
#49082=ORIENTED_EDGE('',*,*,#35405,.T.);
#49083=ORIENTED_EDGE('',*,*,#35406,.T.);
#49084=ORIENTED_EDGE('',*,*,#35407,.T.);
#49085=ORIENTED_EDGE('',*,*,#35408,.T.);
#49086=ORIENTED_EDGE('',*,*,#35409,.T.);
#49087=ORIENTED_EDGE('',*,*,#35410,.T.);
#49088=ORIENTED_EDGE('',*,*,#35411,.T.);
#49089=ORIENTED_EDGE('',*,*,#35412,.T.);
#49090=ORIENTED_EDGE('',*,*,#35413,.T.);
#49091=ORIENTED_EDGE('',*,*,#35414,.T.);
#49092=ORIENTED_EDGE('',*,*,#35415,.T.);
#49093=ORIENTED_EDGE('',*,*,#35416,.T.);
#49094=ORIENTED_EDGE('',*,*,#35417,.T.);
#49095=ORIENTED_EDGE('',*,*,#35355,.F.);
#49096=ORIENTED_EDGE('',*,*,#35365,.F.);
#49097=ORIENTED_EDGE('',*,*,#35418,.F.);
#49098=ORIENTED_EDGE('',*,*,#35419,.T.);
#49099=ORIENTED_EDGE('',*,*,#35420,.F.);
#49100=ORIENTED_EDGE('',*,*,#35363,.F.);
#49101=ORIENTED_EDGE('',*,*,#35421,.F.);
#49102=ORIENTED_EDGE('',*,*,#35422,.F.);
#49103=ORIENTED_EDGE('',*,*,#35423,.F.);
#49104=ORIENTED_EDGE('',*,*,#35424,.F.);
#49105=ORIENTED_EDGE('',*,*,#35422,.T.);
#49106=ORIENTED_EDGE('',*,*,#35425,.F.);
#49107=ORIENTED_EDGE('',*,*,#35426,.F.);
#49108=ORIENTED_EDGE('',*,*,#35427,.F.);
#49109=ORIENTED_EDGE('',*,*,#35426,.T.);
#49110=ORIENTED_EDGE('',*,*,#35428,.F.);
#49111=ORIENTED_EDGE('',*,*,#35429,.F.);
#49112=ORIENTED_EDGE('',*,*,#35430,.T.);
#49113=ORIENTED_EDGE('',*,*,#35429,.T.);
#49114=ORIENTED_EDGE('',*,*,#35431,.F.);
#49115=ORIENTED_EDGE('',*,*,#35419,.F.);
#49116=ORIENTED_EDGE('',*,*,#35364,.F.);
#49117=ORIENTED_EDGE('',*,*,#35423,.T.);
#49118=ORIENTED_EDGE('',*,*,#35424,.T.);
#49119=ORIENTED_EDGE('',*,*,#35427,.T.);
#49120=ORIENTED_EDGE('',*,*,#35430,.F.);
#49121=ORIENTED_EDGE('',*,*,#35418,.T.);
#49122=ORIENTED_EDGE('',*,*,#35361,.F.);
#49123=ORIENTED_EDGE('',*,*,#35432,.F.);
#49124=ORIENTED_EDGE('',*,*,#35433,.T.);
#49125=ORIENTED_EDGE('',*,*,#35434,.F.);
#49126=ORIENTED_EDGE('',*,*,#35359,.F.);
#49127=ORIENTED_EDGE('',*,*,#35435,.F.);
#49128=ORIENTED_EDGE('',*,*,#35436,.F.);
#49129=ORIENTED_EDGE('',*,*,#35437,.F.);
#49130=ORIENTED_EDGE('',*,*,#35438,.F.);
#49131=ORIENTED_EDGE('',*,*,#35436,.T.);
#49132=ORIENTED_EDGE('',*,*,#35439,.F.);
#49133=ORIENTED_EDGE('',*,*,#35440,.F.);
#49134=ORIENTED_EDGE('',*,*,#35441,.F.);
#49135=ORIENTED_EDGE('',*,*,#35440,.T.);
#49136=ORIENTED_EDGE('',*,*,#35442,.F.);
#49137=ORIENTED_EDGE('',*,*,#35443,.F.);
#49138=ORIENTED_EDGE('',*,*,#35444,.T.);
#49139=ORIENTED_EDGE('',*,*,#35443,.T.);
#49140=ORIENTED_EDGE('',*,*,#35445,.F.);
#49141=ORIENTED_EDGE('',*,*,#35433,.F.);
#49142=ORIENTED_EDGE('',*,*,#35360,.F.);
#49143=ORIENTED_EDGE('',*,*,#35437,.T.);
#49144=ORIENTED_EDGE('',*,*,#35438,.T.);
#49145=ORIENTED_EDGE('',*,*,#35441,.T.);
#49146=ORIENTED_EDGE('',*,*,#35444,.F.);
#49147=ORIENTED_EDGE('',*,*,#35432,.T.);
#49148=ORIENTED_EDGE('',*,*,#35357,.F.);
#49149=ORIENTED_EDGE('',*,*,#35446,.F.);
#49150=ORIENTED_EDGE('',*,*,#35447,.T.);
#49151=ORIENTED_EDGE('',*,*,#35448,.F.);
#49152=ORIENTED_EDGE('',*,*,#35416,.F.);
#49153=ORIENTED_EDGE('',*,*,#35449,.F.);
#49154=ORIENTED_EDGE('',*,*,#35450,.F.);
#49155=ORIENTED_EDGE('',*,*,#35451,.F.);
#49156=ORIENTED_EDGE('',*,*,#35452,.F.);
#49157=ORIENTED_EDGE('',*,*,#35450,.T.);
#49158=ORIENTED_EDGE('',*,*,#35453,.F.);
#49159=ORIENTED_EDGE('',*,*,#35454,.F.);
#49160=ORIENTED_EDGE('',*,*,#35455,.F.);
#49161=ORIENTED_EDGE('',*,*,#35454,.T.);
#49162=ORIENTED_EDGE('',*,*,#35456,.F.);
#49163=ORIENTED_EDGE('',*,*,#35457,.F.);
#49164=ORIENTED_EDGE('',*,*,#35458,.T.);
#49165=ORIENTED_EDGE('',*,*,#35457,.T.);
#49166=ORIENTED_EDGE('',*,*,#35459,.F.);
#49167=ORIENTED_EDGE('',*,*,#35447,.F.);
#49168=ORIENTED_EDGE('',*,*,#35417,.F.);
#49169=ORIENTED_EDGE('',*,*,#35451,.T.);
#49170=ORIENTED_EDGE('',*,*,#35452,.T.);
#49171=ORIENTED_EDGE('',*,*,#35455,.T.);
#49172=ORIENTED_EDGE('',*,*,#35458,.F.);
#49173=ORIENTED_EDGE('',*,*,#35446,.T.);
#49174=ORIENTED_EDGE('',*,*,#35356,.F.);
#49175=ORIENTED_EDGE('',*,*,#35414,.F.);
#49176=ORIENTED_EDGE('',*,*,#35460,.F.);
#49177=ORIENTED_EDGE('',*,*,#35461,.T.);
#49178=ORIENTED_EDGE('',*,*,#35462,.F.);
#49179=ORIENTED_EDGE('',*,*,#35412,.F.);
#49180=ORIENTED_EDGE('',*,*,#35463,.F.);
#49181=ORIENTED_EDGE('',*,*,#35464,.F.);
#49182=ORIENTED_EDGE('',*,*,#35465,.F.);
#49183=ORIENTED_EDGE('',*,*,#35466,.F.);
#49184=ORIENTED_EDGE('',*,*,#35464,.T.);
#49185=ORIENTED_EDGE('',*,*,#35467,.F.);
#49186=ORIENTED_EDGE('',*,*,#35468,.F.);
#49187=ORIENTED_EDGE('',*,*,#35469,.F.);
#49188=ORIENTED_EDGE('',*,*,#35468,.T.);
#49189=ORIENTED_EDGE('',*,*,#35470,.F.);
#49190=ORIENTED_EDGE('',*,*,#35471,.F.);
#49191=ORIENTED_EDGE('',*,*,#35472,.T.);
#49192=ORIENTED_EDGE('',*,*,#35471,.T.);
#49193=ORIENTED_EDGE('',*,*,#35473,.F.);
#49194=ORIENTED_EDGE('',*,*,#35461,.F.);
#49195=ORIENTED_EDGE('',*,*,#35413,.F.);
#49196=ORIENTED_EDGE('',*,*,#35465,.T.);
#49197=ORIENTED_EDGE('',*,*,#35466,.T.);
#49198=ORIENTED_EDGE('',*,*,#35469,.T.);
#49199=ORIENTED_EDGE('',*,*,#35472,.F.);
#49200=ORIENTED_EDGE('',*,*,#35460,.T.);
#49201=ORIENTED_EDGE('',*,*,#35410,.F.);
#49202=ORIENTED_EDGE('',*,*,#35474,.F.);
#49203=ORIENTED_EDGE('',*,*,#35475,.T.);
#49204=ORIENTED_EDGE('',*,*,#35476,.F.);
#49205=ORIENTED_EDGE('',*,*,#35408,.F.);
#49206=ORIENTED_EDGE('',*,*,#35477,.F.);
#49207=ORIENTED_EDGE('',*,*,#35478,.F.);
#49208=ORIENTED_EDGE('',*,*,#35479,.F.);
#49209=ORIENTED_EDGE('',*,*,#35480,.F.);
#49210=ORIENTED_EDGE('',*,*,#35478,.T.);
#49211=ORIENTED_EDGE('',*,*,#35481,.F.);
#49212=ORIENTED_EDGE('',*,*,#35482,.F.);
#49213=ORIENTED_EDGE('',*,*,#35483,.F.);
#49214=ORIENTED_EDGE('',*,*,#35482,.T.);
#49215=ORIENTED_EDGE('',*,*,#35484,.F.);
#49216=ORIENTED_EDGE('',*,*,#35485,.F.);
#49217=ORIENTED_EDGE('',*,*,#35486,.T.);
#49218=ORIENTED_EDGE('',*,*,#35485,.T.);
#49219=ORIENTED_EDGE('',*,*,#35487,.F.);
#49220=ORIENTED_EDGE('',*,*,#35475,.F.);
#49221=ORIENTED_EDGE('',*,*,#35409,.F.);
#49222=ORIENTED_EDGE('',*,*,#35479,.T.);
#49223=ORIENTED_EDGE('',*,*,#35480,.T.);
#49224=ORIENTED_EDGE('',*,*,#35483,.T.);
#49225=ORIENTED_EDGE('',*,*,#35486,.F.);
#49226=ORIENTED_EDGE('',*,*,#35474,.T.);
#49227=ORIENTED_EDGE('',*,*,#35406,.F.);
#49228=ORIENTED_EDGE('',*,*,#35488,.F.);
#49229=ORIENTED_EDGE('',*,*,#35489,.T.);
#49230=ORIENTED_EDGE('',*,*,#35490,.F.);
#49231=ORIENTED_EDGE('',*,*,#35404,.F.);
#49232=ORIENTED_EDGE('',*,*,#35491,.F.);
#49233=ORIENTED_EDGE('',*,*,#35492,.F.);
#49234=ORIENTED_EDGE('',*,*,#35493,.F.);
#49235=ORIENTED_EDGE('',*,*,#35494,.F.);
#49236=ORIENTED_EDGE('',*,*,#35492,.T.);
#49237=ORIENTED_EDGE('',*,*,#35495,.F.);
#49238=ORIENTED_EDGE('',*,*,#35496,.F.);
#49239=ORIENTED_EDGE('',*,*,#35497,.F.);
#49240=ORIENTED_EDGE('',*,*,#35496,.T.);
#49241=ORIENTED_EDGE('',*,*,#35498,.F.);
#49242=ORIENTED_EDGE('',*,*,#35499,.F.);
#49243=ORIENTED_EDGE('',*,*,#35500,.T.);
#49244=ORIENTED_EDGE('',*,*,#35499,.T.);
#49245=ORIENTED_EDGE('',*,*,#35501,.F.);
#49246=ORIENTED_EDGE('',*,*,#35489,.F.);
#49247=ORIENTED_EDGE('',*,*,#35405,.F.);
#49248=ORIENTED_EDGE('',*,*,#35493,.T.);
#49249=ORIENTED_EDGE('',*,*,#35494,.T.);
#49250=ORIENTED_EDGE('',*,*,#35497,.T.);
#49251=ORIENTED_EDGE('',*,*,#35500,.F.);
#49252=ORIENTED_EDGE('',*,*,#35488,.T.);
#49253=ORIENTED_EDGE('',*,*,#35402,.F.);
#49254=ORIENTED_EDGE('',*,*,#35502,.F.);
#49255=ORIENTED_EDGE('',*,*,#35503,.T.);
#49256=ORIENTED_EDGE('',*,*,#35504,.F.);
#49257=ORIENTED_EDGE('',*,*,#35400,.F.);
#49258=ORIENTED_EDGE('',*,*,#35505,.F.);
#49259=ORIENTED_EDGE('',*,*,#35506,.F.);
#49260=ORIENTED_EDGE('',*,*,#35507,.F.);
#49261=ORIENTED_EDGE('',*,*,#35508,.F.);
#49262=ORIENTED_EDGE('',*,*,#35506,.T.);
#49263=ORIENTED_EDGE('',*,*,#35509,.F.);
#49264=ORIENTED_EDGE('',*,*,#35510,.F.);
#49265=ORIENTED_EDGE('',*,*,#35511,.F.);
#49266=ORIENTED_EDGE('',*,*,#35510,.T.);
#49267=ORIENTED_EDGE('',*,*,#35512,.F.);
#49268=ORIENTED_EDGE('',*,*,#35513,.F.);
#49269=ORIENTED_EDGE('',*,*,#35514,.T.);
#49270=ORIENTED_EDGE('',*,*,#35513,.T.);
#49271=ORIENTED_EDGE('',*,*,#35515,.F.);
#49272=ORIENTED_EDGE('',*,*,#35503,.F.);
#49273=ORIENTED_EDGE('',*,*,#35401,.F.);
#49274=ORIENTED_EDGE('',*,*,#35507,.T.);
#49275=ORIENTED_EDGE('',*,*,#35508,.T.);
#49276=ORIENTED_EDGE('',*,*,#35511,.T.);
#49277=ORIENTED_EDGE('',*,*,#35514,.F.);
#49278=ORIENTED_EDGE('',*,*,#35502,.T.);
#49279=ORIENTED_EDGE('',*,*,#35398,.F.);
#49280=ORIENTED_EDGE('',*,*,#35516,.F.);
#49281=ORIENTED_EDGE('',*,*,#35517,.T.);
#49282=ORIENTED_EDGE('',*,*,#35518,.F.);
#49283=ORIENTED_EDGE('',*,*,#35396,.F.);
#49284=ORIENTED_EDGE('',*,*,#35519,.F.);
#49285=ORIENTED_EDGE('',*,*,#35520,.F.);
#49286=ORIENTED_EDGE('',*,*,#35521,.F.);
#49287=ORIENTED_EDGE('',*,*,#35522,.F.);
#49288=ORIENTED_EDGE('',*,*,#35520,.T.);
#49289=ORIENTED_EDGE('',*,*,#35523,.F.);
#49290=ORIENTED_EDGE('',*,*,#35524,.F.);
#49291=ORIENTED_EDGE('',*,*,#35525,.F.);
#49292=ORIENTED_EDGE('',*,*,#35524,.T.);
#49293=ORIENTED_EDGE('',*,*,#35526,.F.);
#49294=ORIENTED_EDGE('',*,*,#35527,.F.);
#49295=ORIENTED_EDGE('',*,*,#35528,.T.);
#49296=ORIENTED_EDGE('',*,*,#35527,.T.);
#49297=ORIENTED_EDGE('',*,*,#35529,.F.);
#49298=ORIENTED_EDGE('',*,*,#35517,.F.);
#49299=ORIENTED_EDGE('',*,*,#35397,.F.);
#49300=ORIENTED_EDGE('',*,*,#35521,.T.);
#49301=ORIENTED_EDGE('',*,*,#35522,.T.);
#49302=ORIENTED_EDGE('',*,*,#35525,.T.);
#49303=ORIENTED_EDGE('',*,*,#35528,.F.);
#49304=ORIENTED_EDGE('',*,*,#35516,.T.);
#49305=ORIENTED_EDGE('',*,*,#35394,.F.);
#49306=ORIENTED_EDGE('',*,*,#35530,.F.);
#49307=ORIENTED_EDGE('',*,*,#35531,.T.);
#49308=ORIENTED_EDGE('',*,*,#35532,.F.);
#49309=ORIENTED_EDGE('',*,*,#35392,.F.);
#49310=ORIENTED_EDGE('',*,*,#35533,.F.);
#49311=ORIENTED_EDGE('',*,*,#35534,.F.);
#49312=ORIENTED_EDGE('',*,*,#35535,.F.);
#49313=ORIENTED_EDGE('',*,*,#35536,.F.);
#49314=ORIENTED_EDGE('',*,*,#35534,.T.);
#49315=ORIENTED_EDGE('',*,*,#35537,.F.);
#49316=ORIENTED_EDGE('',*,*,#35538,.F.);
#49317=ORIENTED_EDGE('',*,*,#35539,.F.);
#49318=ORIENTED_EDGE('',*,*,#35538,.T.);
#49319=ORIENTED_EDGE('',*,*,#35540,.F.);
#49320=ORIENTED_EDGE('',*,*,#35541,.F.);
#49321=ORIENTED_EDGE('',*,*,#35542,.T.);
#49322=ORIENTED_EDGE('',*,*,#35541,.T.);
#49323=ORIENTED_EDGE('',*,*,#35543,.F.);
#49324=ORIENTED_EDGE('',*,*,#35531,.F.);
#49325=ORIENTED_EDGE('',*,*,#35393,.F.);
#49326=ORIENTED_EDGE('',*,*,#35535,.T.);
#49327=ORIENTED_EDGE('',*,*,#35536,.T.);
#49328=ORIENTED_EDGE('',*,*,#35539,.T.);
#49329=ORIENTED_EDGE('',*,*,#35542,.F.);
#49330=ORIENTED_EDGE('',*,*,#35530,.T.);
#49331=ORIENTED_EDGE('',*,*,#35390,.F.);
#49332=ORIENTED_EDGE('',*,*,#35544,.F.);
#49333=ORIENTED_EDGE('',*,*,#35545,.T.);
#49334=ORIENTED_EDGE('',*,*,#35546,.F.);
#49335=ORIENTED_EDGE('',*,*,#35388,.F.);
#49336=ORIENTED_EDGE('',*,*,#35547,.F.);
#49337=ORIENTED_EDGE('',*,*,#35548,.F.);
#49338=ORIENTED_EDGE('',*,*,#35549,.F.);
#49339=ORIENTED_EDGE('',*,*,#35550,.F.);
#49340=ORIENTED_EDGE('',*,*,#35548,.T.);
#49341=ORIENTED_EDGE('',*,*,#35551,.F.);
#49342=ORIENTED_EDGE('',*,*,#35552,.F.);
#49343=ORIENTED_EDGE('',*,*,#35553,.F.);
#49344=ORIENTED_EDGE('',*,*,#35552,.T.);
#49345=ORIENTED_EDGE('',*,*,#35554,.F.);
#49346=ORIENTED_EDGE('',*,*,#35555,.F.);
#49347=ORIENTED_EDGE('',*,*,#35556,.T.);
#49348=ORIENTED_EDGE('',*,*,#35555,.T.);
#49349=ORIENTED_EDGE('',*,*,#35557,.F.);
#49350=ORIENTED_EDGE('',*,*,#35545,.F.);
#49351=ORIENTED_EDGE('',*,*,#35389,.F.);
#49352=ORIENTED_EDGE('',*,*,#35549,.T.);
#49353=ORIENTED_EDGE('',*,*,#35550,.T.);
#49354=ORIENTED_EDGE('',*,*,#35553,.T.);
#49355=ORIENTED_EDGE('',*,*,#35556,.F.);
#49356=ORIENTED_EDGE('',*,*,#35544,.T.);
#49357=ORIENTED_EDGE('',*,*,#35386,.F.);
#49358=ORIENTED_EDGE('',*,*,#35558,.F.);
#49359=ORIENTED_EDGE('',*,*,#35559,.T.);
#49360=ORIENTED_EDGE('',*,*,#35560,.F.);
#49361=ORIENTED_EDGE('',*,*,#35384,.F.);
#49362=ORIENTED_EDGE('',*,*,#35561,.F.);
#49363=ORIENTED_EDGE('',*,*,#35562,.F.);
#49364=ORIENTED_EDGE('',*,*,#35563,.F.);
#49365=ORIENTED_EDGE('',*,*,#35564,.F.);
#49366=ORIENTED_EDGE('',*,*,#35562,.T.);
#49367=ORIENTED_EDGE('',*,*,#35565,.F.);
#49368=ORIENTED_EDGE('',*,*,#35566,.F.);
#49369=ORIENTED_EDGE('',*,*,#35567,.F.);
#49370=ORIENTED_EDGE('',*,*,#35566,.T.);
#49371=ORIENTED_EDGE('',*,*,#35568,.F.);
#49372=ORIENTED_EDGE('',*,*,#35569,.F.);
#49373=ORIENTED_EDGE('',*,*,#35570,.T.);
#49374=ORIENTED_EDGE('',*,*,#35569,.T.);
#49375=ORIENTED_EDGE('',*,*,#35571,.F.);
#49376=ORIENTED_EDGE('',*,*,#35559,.F.);
#49377=ORIENTED_EDGE('',*,*,#35385,.F.);
#49378=ORIENTED_EDGE('',*,*,#35563,.T.);
#49379=ORIENTED_EDGE('',*,*,#35564,.T.);
#49380=ORIENTED_EDGE('',*,*,#35567,.T.);
#49381=ORIENTED_EDGE('',*,*,#35570,.F.);
#49382=ORIENTED_EDGE('',*,*,#35558,.T.);
#49383=ORIENTED_EDGE('',*,*,#35382,.F.);
#49384=ORIENTED_EDGE('',*,*,#35572,.F.);
#49385=ORIENTED_EDGE('',*,*,#35573,.T.);
#49386=ORIENTED_EDGE('',*,*,#35574,.F.);
#49387=ORIENTED_EDGE('',*,*,#35380,.F.);
#49388=ORIENTED_EDGE('',*,*,#35575,.F.);
#49389=ORIENTED_EDGE('',*,*,#35576,.F.);
#49390=ORIENTED_EDGE('',*,*,#35577,.F.);
#49391=ORIENTED_EDGE('',*,*,#35578,.F.);
#49392=ORIENTED_EDGE('',*,*,#35576,.T.);
#49393=ORIENTED_EDGE('',*,*,#35579,.F.);
#49394=ORIENTED_EDGE('',*,*,#35580,.F.);
#49395=ORIENTED_EDGE('',*,*,#35581,.F.);
#49396=ORIENTED_EDGE('',*,*,#35580,.T.);
#49397=ORIENTED_EDGE('',*,*,#35582,.F.);
#49398=ORIENTED_EDGE('',*,*,#35583,.F.);
#49399=ORIENTED_EDGE('',*,*,#35584,.T.);
#49400=ORIENTED_EDGE('',*,*,#35583,.T.);
#49401=ORIENTED_EDGE('',*,*,#35585,.F.);
#49402=ORIENTED_EDGE('',*,*,#35573,.F.);
#49403=ORIENTED_EDGE('',*,*,#35381,.F.);
#49404=ORIENTED_EDGE('',*,*,#35577,.T.);
#49405=ORIENTED_EDGE('',*,*,#35578,.T.);
#49406=ORIENTED_EDGE('',*,*,#35581,.T.);
#49407=ORIENTED_EDGE('',*,*,#35584,.F.);
#49408=ORIENTED_EDGE('',*,*,#35572,.T.);
#49409=ORIENTED_EDGE('',*,*,#35378,.F.);
#49410=ORIENTED_EDGE('',*,*,#35586,.F.);
#49411=ORIENTED_EDGE('',*,*,#35587,.T.);
#49412=ORIENTED_EDGE('',*,*,#35588,.F.);
#49413=ORIENTED_EDGE('',*,*,#35376,.F.);
#49414=ORIENTED_EDGE('',*,*,#35589,.F.);
#49415=ORIENTED_EDGE('',*,*,#35590,.F.);
#49416=ORIENTED_EDGE('',*,*,#35591,.F.);
#49417=ORIENTED_EDGE('',*,*,#35592,.F.);
#49418=ORIENTED_EDGE('',*,*,#35590,.T.);
#49419=ORIENTED_EDGE('',*,*,#35593,.F.);
#49420=ORIENTED_EDGE('',*,*,#35594,.F.);
#49421=ORIENTED_EDGE('',*,*,#35595,.F.);
#49422=ORIENTED_EDGE('',*,*,#35594,.T.);
#49423=ORIENTED_EDGE('',*,*,#35596,.F.);
#49424=ORIENTED_EDGE('',*,*,#35597,.F.);
#49425=ORIENTED_EDGE('',*,*,#35598,.T.);
#49426=ORIENTED_EDGE('',*,*,#35597,.T.);
#49427=ORIENTED_EDGE('',*,*,#35599,.F.);
#49428=ORIENTED_EDGE('',*,*,#35587,.F.);
#49429=ORIENTED_EDGE('',*,*,#35377,.F.);
#49430=ORIENTED_EDGE('',*,*,#35591,.T.);
#49431=ORIENTED_EDGE('',*,*,#35592,.T.);
#49432=ORIENTED_EDGE('',*,*,#35595,.T.);
#49433=ORIENTED_EDGE('',*,*,#35598,.F.);
#49434=ORIENTED_EDGE('',*,*,#35586,.T.);
#49435=ORIENTED_EDGE('',*,*,#35374,.F.);
#49436=ORIENTED_EDGE('',*,*,#35600,.F.);
#49437=ORIENTED_EDGE('',*,*,#35601,.T.);
#49438=ORIENTED_EDGE('',*,*,#35602,.F.);
#49439=ORIENTED_EDGE('',*,*,#35372,.F.);
#49440=ORIENTED_EDGE('',*,*,#35603,.F.);
#49441=ORIENTED_EDGE('',*,*,#35604,.F.);
#49442=ORIENTED_EDGE('',*,*,#35605,.F.);
#49443=ORIENTED_EDGE('',*,*,#35606,.F.);
#49444=ORIENTED_EDGE('',*,*,#35604,.T.);
#49445=ORIENTED_EDGE('',*,*,#35607,.F.);
#49446=ORIENTED_EDGE('',*,*,#35608,.F.);
#49447=ORIENTED_EDGE('',*,*,#35609,.F.);
#49448=ORIENTED_EDGE('',*,*,#35608,.T.);
#49449=ORIENTED_EDGE('',*,*,#35610,.F.);
#49450=ORIENTED_EDGE('',*,*,#35611,.F.);
#49451=ORIENTED_EDGE('',*,*,#35612,.T.);
#49452=ORIENTED_EDGE('',*,*,#35611,.T.);
#49453=ORIENTED_EDGE('',*,*,#35613,.F.);
#49454=ORIENTED_EDGE('',*,*,#35601,.F.);
#49455=ORIENTED_EDGE('',*,*,#35373,.F.);
#49456=ORIENTED_EDGE('',*,*,#35605,.T.);
#49457=ORIENTED_EDGE('',*,*,#35606,.T.);
#49458=ORIENTED_EDGE('',*,*,#35609,.T.);
#49459=ORIENTED_EDGE('',*,*,#35612,.F.);
#49460=ORIENTED_EDGE('',*,*,#35600,.T.);
#49461=ORIENTED_EDGE('',*,*,#35368,.F.);
#49462=ORIENTED_EDGE('',*,*,#35614,.F.);
#49463=ORIENTED_EDGE('',*,*,#35615,.F.);
#49464=ORIENTED_EDGE('',*,*,#35616,.F.);
#49465=ORIENTED_EDGE('',*,*,#35617,.F.);
#49466=ORIENTED_EDGE('',*,*,#35615,.T.);
#49467=ORIENTED_EDGE('',*,*,#35618,.F.);
#49468=ORIENTED_EDGE('',*,*,#35619,.F.);
#49469=ORIENTED_EDGE('',*,*,#35620,.F.);
#49470=ORIENTED_EDGE('',*,*,#35619,.T.);
#49471=ORIENTED_EDGE('',*,*,#35621,.F.);
#49472=ORIENTED_EDGE('',*,*,#35622,.F.);
#49473=ORIENTED_EDGE('',*,*,#35623,.T.);
#49474=ORIENTED_EDGE('',*,*,#35622,.T.);
#49475=ORIENTED_EDGE('',*,*,#35624,.F.);
#49476=ORIENTED_EDGE('',*,*,#35625,.F.);
#49477=ORIENTED_EDGE('',*,*,#35370,.F.);
#49478=ORIENTED_EDGE('',*,*,#35626,.F.);
#49479=ORIENTED_EDGE('',*,*,#35625,.T.);
#49480=ORIENTED_EDGE('',*,*,#35627,.F.);
#49481=ORIENTED_EDGE('',*,*,#35369,.F.);
#49482=ORIENTED_EDGE('',*,*,#35616,.T.);
#49483=ORIENTED_EDGE('',*,*,#35617,.T.);
#49484=ORIENTED_EDGE('',*,*,#35620,.T.);
#49485=ORIENTED_EDGE('',*,*,#35623,.F.);
#49486=ORIENTED_EDGE('',*,*,#35626,.T.);
#49487=ORIENTED_EDGE('',*,*,#35628,.T.);
#49488=ORIENTED_EDGE('',*,*,#35629,.T.);
#49489=ORIENTED_EDGE('',*,*,#35630,.F.);
#49490=ORIENTED_EDGE('',*,*,#35629,.F.);
#49491=ORIENTED_EDGE('',*,*,#35333,.T.);
#49492=ORIENTED_EDGE('',*,*,#35336,.T.);
#49493=ORIENTED_EDGE('',*,*,#35334,.T.);
#49494=ORIENTED_EDGE('',*,*,#35326,.T.);
#49495=ORIENTED_EDGE('',*,*,#35366,.F.);
#49496=ORIENTED_EDGE('',*,*,#35420,.T.);
#49497=ORIENTED_EDGE('',*,*,#35431,.T.);
#49498=ORIENTED_EDGE('',*,*,#35428,.T.);
#49499=ORIENTED_EDGE('',*,*,#35425,.T.);
#49500=ORIENTED_EDGE('',*,*,#35421,.T.);
#49501=ORIENTED_EDGE('',*,*,#35362,.F.);
#49502=ORIENTED_EDGE('',*,*,#35434,.T.);
#49503=ORIENTED_EDGE('',*,*,#35445,.T.);
#49504=ORIENTED_EDGE('',*,*,#35442,.T.);
#49505=ORIENTED_EDGE('',*,*,#35439,.T.);
#49506=ORIENTED_EDGE('',*,*,#35435,.T.);
#49507=ORIENTED_EDGE('',*,*,#35358,.F.);
#49508=ORIENTED_EDGE('',*,*,#35448,.T.);
#49509=ORIENTED_EDGE('',*,*,#35459,.T.);
#49510=ORIENTED_EDGE('',*,*,#35456,.T.);
#49511=ORIENTED_EDGE('',*,*,#35453,.T.);
#49512=ORIENTED_EDGE('',*,*,#35449,.T.);
#49513=ORIENTED_EDGE('',*,*,#35415,.F.);
#49514=ORIENTED_EDGE('',*,*,#35462,.T.);
#49515=ORIENTED_EDGE('',*,*,#35473,.T.);
#49516=ORIENTED_EDGE('',*,*,#35470,.T.);
#49517=ORIENTED_EDGE('',*,*,#35467,.T.);
#49518=ORIENTED_EDGE('',*,*,#35463,.T.);
#49519=ORIENTED_EDGE('',*,*,#35411,.F.);
#49520=ORIENTED_EDGE('',*,*,#35476,.T.);
#49521=ORIENTED_EDGE('',*,*,#35487,.T.);
#49522=ORIENTED_EDGE('',*,*,#35484,.T.);
#49523=ORIENTED_EDGE('',*,*,#35481,.T.);
#49524=ORIENTED_EDGE('',*,*,#35477,.T.);
#49525=ORIENTED_EDGE('',*,*,#35407,.F.);
#49526=ORIENTED_EDGE('',*,*,#35490,.T.);
#49527=ORIENTED_EDGE('',*,*,#35501,.T.);
#49528=ORIENTED_EDGE('',*,*,#35498,.T.);
#49529=ORIENTED_EDGE('',*,*,#35495,.T.);
#49530=ORIENTED_EDGE('',*,*,#35491,.T.);
#49531=ORIENTED_EDGE('',*,*,#35403,.F.);
#49532=ORIENTED_EDGE('',*,*,#35504,.T.);
#49533=ORIENTED_EDGE('',*,*,#35515,.T.);
#49534=ORIENTED_EDGE('',*,*,#35512,.T.);
#49535=ORIENTED_EDGE('',*,*,#35509,.T.);
#49536=ORIENTED_EDGE('',*,*,#35505,.T.);
#49537=ORIENTED_EDGE('',*,*,#35399,.F.);
#49538=ORIENTED_EDGE('',*,*,#35518,.T.);
#49539=ORIENTED_EDGE('',*,*,#35529,.T.);
#49540=ORIENTED_EDGE('',*,*,#35526,.T.);
#49541=ORIENTED_EDGE('',*,*,#35523,.T.);
#49542=ORIENTED_EDGE('',*,*,#35519,.T.);
#49543=ORIENTED_EDGE('',*,*,#35395,.F.);
#49544=ORIENTED_EDGE('',*,*,#35532,.T.);
#49545=ORIENTED_EDGE('',*,*,#35543,.T.);
#49546=ORIENTED_EDGE('',*,*,#35540,.T.);
#49547=ORIENTED_EDGE('',*,*,#35537,.T.);
#49548=ORIENTED_EDGE('',*,*,#35533,.T.);
#49549=ORIENTED_EDGE('',*,*,#35391,.F.);
#49550=ORIENTED_EDGE('',*,*,#35546,.T.);
#49551=ORIENTED_EDGE('',*,*,#35557,.T.);
#49552=ORIENTED_EDGE('',*,*,#35554,.T.);
#49553=ORIENTED_EDGE('',*,*,#35551,.T.);
#49554=ORIENTED_EDGE('',*,*,#35547,.T.);
#49555=ORIENTED_EDGE('',*,*,#35387,.F.);
#49556=ORIENTED_EDGE('',*,*,#35560,.T.);
#49557=ORIENTED_EDGE('',*,*,#35571,.T.);
#49558=ORIENTED_EDGE('',*,*,#35568,.T.);
#49559=ORIENTED_EDGE('',*,*,#35565,.T.);
#49560=ORIENTED_EDGE('',*,*,#35561,.T.);
#49561=ORIENTED_EDGE('',*,*,#35383,.F.);
#49562=ORIENTED_EDGE('',*,*,#35574,.T.);
#49563=ORIENTED_EDGE('',*,*,#35585,.T.);
#49564=ORIENTED_EDGE('',*,*,#35582,.T.);
#49565=ORIENTED_EDGE('',*,*,#35579,.T.);
#49566=ORIENTED_EDGE('',*,*,#35575,.T.);
#49567=ORIENTED_EDGE('',*,*,#35379,.F.);
#49568=ORIENTED_EDGE('',*,*,#35588,.T.);
#49569=ORIENTED_EDGE('',*,*,#35599,.T.);
#49570=ORIENTED_EDGE('',*,*,#35596,.T.);
#49571=ORIENTED_EDGE('',*,*,#35593,.T.);
#49572=ORIENTED_EDGE('',*,*,#35589,.T.);
#49573=ORIENTED_EDGE('',*,*,#35375,.F.);
#49574=ORIENTED_EDGE('',*,*,#35602,.T.);
#49575=ORIENTED_EDGE('',*,*,#35613,.T.);
#49576=ORIENTED_EDGE('',*,*,#35610,.T.);
#49577=ORIENTED_EDGE('',*,*,#35607,.T.);
#49578=ORIENTED_EDGE('',*,*,#35603,.T.);
#49579=ORIENTED_EDGE('',*,*,#35371,.F.);
#49580=ORIENTED_EDGE('',*,*,#35627,.T.);
#49581=ORIENTED_EDGE('',*,*,#35624,.T.);
#49582=ORIENTED_EDGE('',*,*,#35621,.T.);
#49583=ORIENTED_EDGE('',*,*,#35618,.T.);
#49584=ORIENTED_EDGE('',*,*,#35614,.T.);
#49585=ORIENTED_EDGE('',*,*,#35367,.F.);
#49586=ORIENTED_EDGE('',*,*,#35340,.T.);
#49587=ORIENTED_EDGE('',*,*,#35352,.T.);
#49588=ORIENTED_EDGE('',*,*,#35349,.T.);
#49589=ORIENTED_EDGE('',*,*,#35346,.T.);
#49590=ORIENTED_EDGE('',*,*,#35342,.T.);
#49591=ORIENTED_EDGE('',*,*,#35630,.T.);
#49592=ORIENTED_EDGE('',*,*,#35631,.F.);
#49593=ORIENTED_EDGE('',*,*,#35354,.T.);
#49594=ORIENTED_EDGE('',*,*,#35632,.F.);
#49595=ORIENTED_EDGE('',*,*,#35633,.T.);
#49596=ORIENTED_EDGE('',*,*,#35631,.T.);
#49597=ORIENTED_EDGE('',*,*,#35633,.F.);
#49598=ORIENTED_EDGE('',*,*,#35328,.T.);
#49599=ORIENTED_EDGE('',*,*,#35330,.T.);
#49600=ORIENTED_EDGE('',*,*,#35329,.T.);
#49601=ORIENTED_EDGE('',*,*,#35634,.F.);
#49602=ORIENTED_EDGE('',*,*,#35635,.T.);
#49603=ORIENTED_EDGE('',*,*,#35632,.T.);
#49604=ORIENTED_EDGE('',*,*,#35635,.F.);
#49605=ORIENTED_EDGE('',*,*,#35634,.T.);
#49606=ORIENTED_EDGE('',*,*,#35628,.F.);
#59078=ADVANCED_FACE('',(#5978),#3043,.T.);
#59079=ADVANCED_FACE('',(#5979),#636,.F.);
#59080=ADVANCED_FACE('',(#5980),#3044,.T.);
#59081=ADVANCED_FACE('',(#5981),#3045,.T.);
#59082=ADVANCED_FACE('',(#5982),#3046,.T.);
#59083=ADVANCED_FACE('',(#5983),#110,.T.);
#59084=ADVANCED_FACE('',(#5984),#637,.T.);
#59085=ADVANCED_FACE('',(#5985),#111,.T.);
#59086=ADVANCED_FACE('',(#5986),#3047,.T.);
#59087=ADVANCED_FACE('',(#5987),#638,.T.);
#59088=ADVANCED_FACE('',(#5988),#3048,.T.);
#59089=ADVANCED_FACE('',(#5989),#3049,.T.);
#59090=ADVANCED_FACE('',(#5990),#112,.T.);
#59091=ADVANCED_FACE('',(#5991),#639,.T.);
#59092=ADVANCED_FACE('',(#5992),#113,.T.);
#59093=ADVANCED_FACE('',(#5993),#3050,.T.);
#59094=ADVANCED_FACE('',(#5994),#3051,.T.);
#59095=ADVANCED_FACE('',(#5995),#3052,.T.);
#59096=ADVANCED_FACE('',(#5996),#114,.T.);
#59097=ADVANCED_FACE('',(#5997),#640,.T.);
#59098=ADVANCED_FACE('',(#5998),#115,.T.);
#59099=ADVANCED_FACE('',(#5999),#3053,.T.);
#59100=ADVANCED_FACE('',(#6000),#3054,.T.);
#59101=ADVANCED_FACE('',(#6001),#3055,.T.);
#59102=ADVANCED_FACE('',(#6002),#116,.T.);
#59103=ADVANCED_FACE('',(#6003),#641,.T.);
#59104=ADVANCED_FACE('',(#6004),#117,.T.);
#59105=ADVANCED_FACE('',(#6005),#3056,.T.);
#59106=ADVANCED_FACE('',(#6006),#3057,.T.);
#59107=ADVANCED_FACE('',(#6007),#3058,.T.);
#59108=ADVANCED_FACE('',(#6008),#118,.T.);
#59109=ADVANCED_FACE('',(#6009),#642,.T.);
#59110=ADVANCED_FACE('',(#6010),#119,.T.);
#59111=ADVANCED_FACE('',(#6011),#3059,.T.);
#59112=ADVANCED_FACE('',(#6012),#3060,.T.);
#59113=ADVANCED_FACE('',(#6013),#3061,.T.);
#59114=ADVANCED_FACE('',(#6014),#120,.T.);
#59115=ADVANCED_FACE('',(#6015),#643,.T.);
#59116=ADVANCED_FACE('',(#6016),#121,.T.);
#59117=ADVANCED_FACE('',(#6017),#3062,.T.);
#59118=ADVANCED_FACE('',(#6018),#3063,.T.);
#59119=ADVANCED_FACE('',(#6019),#3064,.T.);
#59120=ADVANCED_FACE('',(#6020),#122,.T.);
#59121=ADVANCED_FACE('',(#6021),#644,.T.);
#59122=ADVANCED_FACE('',(#6022),#123,.T.);
#59123=ADVANCED_FACE('',(#6023),#3065,.T.);
#59124=ADVANCED_FACE('',(#6024),#3066,.T.);
#59125=ADVANCED_FACE('',(#6025),#3067,.T.);
#59126=ADVANCED_FACE('',(#6026),#124,.T.);
#59127=ADVANCED_FACE('',(#6027),#645,.T.);
#59128=ADVANCED_FACE('',(#6028),#125,.T.);
#59129=ADVANCED_FACE('',(#6029),#3068,.T.);
#59130=ADVANCED_FACE('',(#6030),#3069,.T.);
#59131=ADVANCED_FACE('',(#6031),#3070,.T.);
#59132=ADVANCED_FACE('',(#6032),#126,.T.);
#59133=ADVANCED_FACE('',(#6033),#646,.T.);
#59134=ADVANCED_FACE('',(#6034),#127,.T.);
#59135=ADVANCED_FACE('',(#6035),#3071,.T.);
#59136=ADVANCED_FACE('',(#6036),#3072,.T.);
#59137=ADVANCED_FACE('',(#6037),#3073,.T.);
#59138=ADVANCED_FACE('',(#6038),#128,.T.);
#59139=ADVANCED_FACE('',(#6039),#647,.T.);
#59140=ADVANCED_FACE('',(#6040),#129,.T.);
#59141=ADVANCED_FACE('',(#6041),#3074,.T.);
#59142=ADVANCED_FACE('',(#6042),#3075,.T.);
#59143=ADVANCED_FACE('',(#6043),#3076,.T.);
#59144=ADVANCED_FACE('',(#6044),#130,.T.);
#59145=ADVANCED_FACE('',(#6045),#648,.T.);
#59146=ADVANCED_FACE('',(#6046),#131,.T.);
#59147=ADVANCED_FACE('',(#6047),#3077,.T.);
#59148=ADVANCED_FACE('',(#6048),#3078,.T.);
#59149=ADVANCED_FACE('',(#6049),#3079,.T.);
#59150=ADVANCED_FACE('',(#6050),#132,.T.);
#59151=ADVANCED_FACE('',(#6051),#649,.T.);
#59152=ADVANCED_FACE('',(#6052),#133,.T.);
#59153=ADVANCED_FACE('',(#6053),#3080,.T.);
#59154=ADVANCED_FACE('',(#6054),#3081,.T.);
#59155=ADVANCED_FACE('',(#6055),#3082,.T.);
#59156=ADVANCED_FACE('',(#6056),#134,.T.);
#59157=ADVANCED_FACE('',(#6057),#650,.T.);
#59158=ADVANCED_FACE('',(#6058),#135,.T.);
#59159=ADVANCED_FACE('',(#6059),#3083,.T.);
#59160=ADVANCED_FACE('',(#6060),#3084,.T.);
#59161=ADVANCED_FACE('',(#6061),#3085,.T.);
#59162=ADVANCED_FACE('',(#6062),#136,.T.);
#59163=ADVANCED_FACE('',(#6063),#651,.T.);
#59164=ADVANCED_FACE('',(#6064),#137,.T.);
#59165=ADVANCED_FACE('',(#6065),#3086,.T.);
#59166=ADVANCED_FACE('',(#6066),#3087,.T.);
#59167=ADVANCED_FACE('',(#6067),#3088,.T.);
#59168=ADVANCED_FACE('',(#6068),#138,.T.);
#59169=ADVANCED_FACE('',(#6069),#652,.T.);
#59170=ADVANCED_FACE('',(#6070),#139,.T.);
#59171=ADVANCED_FACE('',(#6071),#3089,.T.);
#59172=ADVANCED_FACE('',(#6072),#3090,.T.);
#59173=ADVANCED_FACE('',(#6073),#140,.T.);
#59174=ADVANCED_FACE('',(#6074),#653,.T.);
#59175=ADVANCED_FACE('',(#6075),#141,.T.);
#59176=ADVANCED_FACE('',(#6076),#3091,.T.);
#59177=ADVANCED_FACE('',(#6077),#3092,.T.);
#59178=ADVANCED_FACE('',(#6078,#1827),#654,.F.);
#59179=ADVANCED_FACE('',(#6079,#1828),#3093,.T.);
#59180=ADVANCED_FACE('',(#6080,#1829),#3094,.T.);
#59181=ADVANCED_FACE('',(#6081,#1830),#655,.T.);
#59182=ADVANCED_FACE('',(#6082),#913,.T.);
#59183=ADVANCED_FACE('',(#6083,#1831),#3095,.T.);
#60396=CLOSED_SHELL('',(#59078,#59079,#59080,#59081,#59082,#59083,#59084,
#59085,#59086,#59087,#59088,#59089,#59090,#59091,#59092,#59093,#59094,#59095,
#59096,#59097,#59098,#59099,#59100,#59101,#59102,#59103,#59104,#59105,#59106,
#59107,#59108,#59109,#59110,#59111,#59112,#59113,#59114,#59115,#59116,#59117,
#59118,#59119,#59120,#59121,#59122,#59123,#59124,#59125,#59126,#59127,#59128,
#59129,#59130,#59131,#59132,#59133,#59134,#59135,#59136,#59137,#59138,#59139,
#59140,#59141,#59142,#59143,#59144,#59145,#59146,#59147,#59148,#59149,#59150,
#59151,#59152,#59153,#59154,#59155,#59156,#59157,#59158,#59159,#59160,#59161,
#59162,#59163,#59164,#59165,#59166,#59167,#59168,#59169,#59170,#59171,#59172,
#59173,#59174,#59175,#59176,#59177,#59178,#59179,#59180,#59181,#59182,#59183));
#61989=AXIS2_PLACEMENT_3D('',#92656,#69989,#69990);
#61990=AXIS2_PLACEMENT_3D('',#92657,#69991,#69992);
#61991=AXIS2_PLACEMENT_3D('',#92661,#69994,#69995);
#61992=AXIS2_PLACEMENT_3D('',#92662,#69996,#69997);
#61993=AXIS2_PLACEMENT_3D('',#92708,#69999,#70000);
#61994=AXIS2_PLACEMENT_3D('',#92730,#70001,#70002);
#61995=AXIS2_PLACEMENT_3D('',#92731,#70003,#70004);
#61996=AXIS2_PLACEMENT_3D('',#92733,#70006,#70007);
#61997=AXIS2_PLACEMENT_3D('',#92742,#70012,#70013);
#61998=AXIS2_PLACEMENT_3D('',#92894,#70019,#70020);
#61999=AXIS2_PLACEMENT_3D('',#92896,#70021,#70022);
#62000=AXIS2_PLACEMENT_3D('',#92898,#70023,#70024);
#62001=AXIS2_PLACEMENT_3D('',#93040,#70026,#70027);
#62002=AXIS2_PLACEMENT_3D('',#93041,#70028,#70029);
#62003=AXIS2_PLACEMENT_3D('',#93042,#70030,#70031);
#62004=AXIS2_PLACEMENT_3D('',#93044,#70032,#70033);
#62005=AXIS2_PLACEMENT_3D('',#93048,#70035,#70036);
#62006=AXIS2_PLACEMENT_3D('',#93052,#70038,#70039);
#62007=AXIS2_PLACEMENT_3D('',#93056,#70041,#70042);
#62008=AXIS2_PLACEMENT_3D('',#93060,#70044,#70045);
#62009=AXIS2_PLACEMENT_3D('',#93064,#70047,#70048);
#62010=AXIS2_PLACEMENT_3D('',#93067,#70050,#70051);
#62011=AXIS2_PLACEMENT_3D('',#93069,#70052,#70053);
#62012=AXIS2_PLACEMENT_3D('',#93073,#70055,#70056);
#62013=AXIS2_PLACEMENT_3D('',#93077,#70058,#70059);
#62014=AXIS2_PLACEMENT_3D('',#93081,#70061,#70062);
#62015=AXIS2_PLACEMENT_3D('',#93085,#70064,#70065);
#62016=AXIS2_PLACEMENT_3D('',#93089,#70067,#70068);
#62017=AXIS2_PLACEMENT_3D('',#93093,#70070,#70071);
#62018=AXIS2_PLACEMENT_3D('',#93097,#70073,#70074);
#62019=AXIS2_PLACEMENT_3D('',#93101,#70076,#70077);
#62020=AXIS2_PLACEMENT_3D('',#93105,#70079,#70080);
#62021=AXIS2_PLACEMENT_3D('',#93109,#70082,#70083);
#62022=AXIS2_PLACEMENT_3D('',#93113,#70085,#70086);
#62023=AXIS2_PLACEMENT_3D('',#93117,#70088,#70089);
#62024=AXIS2_PLACEMENT_3D('',#93121,#70091,#70092);
#62025=AXIS2_PLACEMENT_3D('',#93125,#70094,#70095);
#62026=AXIS2_PLACEMENT_3D('',#93129,#70097,#70098);
#62027=AXIS2_PLACEMENT_3D('',#93133,#70100,#70101);
#62028=AXIS2_PLACEMENT_3D('',#93137,#70103,#70104);
#62029=AXIS2_PLACEMENT_3D('',#93141,#70106,#70107);
#62030=AXIS2_PLACEMENT_3D('',#93145,#70109,#70110);
#62031=AXIS2_PLACEMENT_3D('',#93149,#70112,#70113);
#62032=AXIS2_PLACEMENT_3D('',#93153,#70115,#70116);
#62033=AXIS2_PLACEMENT_3D('',#93157,#70118,#70119);
#62034=AXIS2_PLACEMENT_3D('',#93161,#70121,#70122);
#62035=AXIS2_PLACEMENT_3D('',#93165,#70124,#70125);
#62036=AXIS2_PLACEMENT_3D('',#93168,#70127,#70128);
#62037=AXIS2_PLACEMENT_3D('',#93169,#70129,#70130);
#62038=AXIS2_PLACEMENT_3D('',#93175,#70134,#70135);
#62039=AXIS2_PLACEMENT_3D('',#93324,#70140,#70141);
#62040=AXIS2_PLACEMENT_3D('',#93326,#70142,#70143);
#62041=AXIS2_PLACEMENT_3D('',#93328,#70144,#70145);
#62042=AXIS2_PLACEMENT_3D('',#93470,#70147,#70148);
#62043=AXIS2_PLACEMENT_3D('',#93471,#70149,#70150);
#62044=AXIS2_PLACEMENT_3D('',#93477,#70154,#70155);
#62045=AXIS2_PLACEMENT_3D('',#93626,#70160,#70161);
#62046=AXIS2_PLACEMENT_3D('',#93628,#70162,#70163);
#62047=AXIS2_PLACEMENT_3D('',#93630,#70164,#70165);
#62048=AXIS2_PLACEMENT_3D('',#93772,#70167,#70168);
#62049=AXIS2_PLACEMENT_3D('',#93773,#70169,#70170);
#62050=AXIS2_PLACEMENT_3D('',#93779,#70174,#70175);
#62051=AXIS2_PLACEMENT_3D('',#93928,#70180,#70181);
#62052=AXIS2_PLACEMENT_3D('',#93930,#70182,#70183);
#62053=AXIS2_PLACEMENT_3D('',#93932,#70184,#70185);
#62054=AXIS2_PLACEMENT_3D('',#94074,#70187,#70188);
#62055=AXIS2_PLACEMENT_3D('',#94075,#70189,#70190);
#62056=AXIS2_PLACEMENT_3D('',#94081,#70194,#70195);
#62057=AXIS2_PLACEMENT_3D('',#94230,#70200,#70201);
#62058=AXIS2_PLACEMENT_3D('',#94232,#70202,#70203);
#62059=AXIS2_PLACEMENT_3D('',#94234,#70204,#70205);
#62060=AXIS2_PLACEMENT_3D('',#94376,#70207,#70208);
#62061=AXIS2_PLACEMENT_3D('',#94377,#70209,#70210);
#62062=AXIS2_PLACEMENT_3D('',#94383,#70214,#70215);
#62063=AXIS2_PLACEMENT_3D('',#94532,#70220,#70221);
#62064=AXIS2_PLACEMENT_3D('',#94534,#70222,#70223);
#62065=AXIS2_PLACEMENT_3D('',#94536,#70224,#70225);
#62066=AXIS2_PLACEMENT_3D('',#94678,#70227,#70228);
#62067=AXIS2_PLACEMENT_3D('',#94679,#70229,#70230);
#62068=AXIS2_PLACEMENT_3D('',#94685,#70234,#70235);
#62069=AXIS2_PLACEMENT_3D('',#94834,#70240,#70241);
#62070=AXIS2_PLACEMENT_3D('',#94836,#70242,#70243);
#62071=AXIS2_PLACEMENT_3D('',#94838,#70244,#70245);
#62072=AXIS2_PLACEMENT_3D('',#94980,#70247,#70248);
#62073=AXIS2_PLACEMENT_3D('',#94981,#70249,#70250);
#62074=AXIS2_PLACEMENT_3D('',#94987,#70254,#70255);
#62075=AXIS2_PLACEMENT_3D('',#95136,#70260,#70261);
#62076=AXIS2_PLACEMENT_3D('',#95138,#70262,#70263);
#62077=AXIS2_PLACEMENT_3D('',#95140,#70264,#70265);
#62078=AXIS2_PLACEMENT_3D('',#95282,#70267,#70268);
#62079=AXIS2_PLACEMENT_3D('',#95283,#70269,#70270);
#62080=AXIS2_PLACEMENT_3D('',#95289,#70274,#70275);
#62081=AXIS2_PLACEMENT_3D('',#95438,#70280,#70281);
#62082=AXIS2_PLACEMENT_3D('',#95440,#70282,#70283);
#62083=AXIS2_PLACEMENT_3D('',#95442,#70284,#70285);
#62084=AXIS2_PLACEMENT_3D('',#95584,#70287,#70288);
#62085=AXIS2_PLACEMENT_3D('',#95585,#70289,#70290);
#62086=AXIS2_PLACEMENT_3D('',#95591,#70294,#70295);
#62087=AXIS2_PLACEMENT_3D('',#95740,#70300,#70301);
#62088=AXIS2_PLACEMENT_3D('',#95742,#70302,#70303);
#62089=AXIS2_PLACEMENT_3D('',#95744,#70304,#70305);
#62090=AXIS2_PLACEMENT_3D('',#95886,#70307,#70308);
#62091=AXIS2_PLACEMENT_3D('',#95887,#70309,#70310);
#62092=AXIS2_PLACEMENT_3D('',#95893,#70314,#70315);
#62093=AXIS2_PLACEMENT_3D('',#96042,#70320,#70321);
#62094=AXIS2_PLACEMENT_3D('',#96044,#70322,#70323);
#62095=AXIS2_PLACEMENT_3D('',#96046,#70324,#70325);
#62096=AXIS2_PLACEMENT_3D('',#96188,#70327,#70328);
#62097=AXIS2_PLACEMENT_3D('',#96189,#70329,#70330);
#62098=AXIS2_PLACEMENT_3D('',#96195,#70334,#70335);
#62099=AXIS2_PLACEMENT_3D('',#96344,#70340,#70341);
#62100=AXIS2_PLACEMENT_3D('',#96346,#70342,#70343);
#62101=AXIS2_PLACEMENT_3D('',#96348,#70344,#70345);
#62102=AXIS2_PLACEMENT_3D('',#96490,#70347,#70348);
#62103=AXIS2_PLACEMENT_3D('',#96491,#70349,#70350);
#62104=AXIS2_PLACEMENT_3D('',#96497,#70354,#70355);
#62105=AXIS2_PLACEMENT_3D('',#96646,#70360,#70361);
#62106=AXIS2_PLACEMENT_3D('',#96648,#70362,#70363);
#62107=AXIS2_PLACEMENT_3D('',#96650,#70364,#70365);
#62108=AXIS2_PLACEMENT_3D('',#96792,#70367,#70368);
#62109=AXIS2_PLACEMENT_3D('',#96793,#70369,#70370);
#62110=AXIS2_PLACEMENT_3D('',#96799,#70374,#70375);
#62111=AXIS2_PLACEMENT_3D('',#96948,#70380,#70381);
#62112=AXIS2_PLACEMENT_3D('',#96950,#70382,#70383);
#62113=AXIS2_PLACEMENT_3D('',#96952,#70384,#70385);
#62114=AXIS2_PLACEMENT_3D('',#97094,#70387,#70388);
#62115=AXIS2_PLACEMENT_3D('',#97095,#70389,#70390);
#62116=AXIS2_PLACEMENT_3D('',#97101,#70394,#70395);
#62117=AXIS2_PLACEMENT_3D('',#97250,#70400,#70401);
#62118=AXIS2_PLACEMENT_3D('',#97252,#70402,#70403);
#62119=AXIS2_PLACEMENT_3D('',#97254,#70404,#70405);
#62120=AXIS2_PLACEMENT_3D('',#97396,#70407,#70408);
#62121=AXIS2_PLACEMENT_3D('',#97397,#70409,#70410);
#62122=AXIS2_PLACEMENT_3D('',#97546,#70415,#70416);
#62123=AXIS2_PLACEMENT_3D('',#97548,#70417,#70418);
#62124=AXIS2_PLACEMENT_3D('',#97550,#70419,#70420);
#62125=AXIS2_PLACEMENT_3D('',#97695,#70423,#70424);
#62126=AXIS2_PLACEMENT_3D('',#97698,#70427,#70428);
#62127=AXIS2_PLACEMENT_3D('',#97699,#70429,#70430);
#62128=AXIS2_PLACEMENT_3D('',#97701,#70431,#70432);
#62129=AXIS2_PLACEMENT_3D('',#97704,#70434,#70435);
#62130=AXIS2_PLACEMENT_3D('',#97705,#70436,#70437);
#62131=AXIS2_PLACEMENT_3D('',#97706,#70438,#70439);
#62132=AXIS2_PLACEMENT_3D('',#97708,#70440,#70441);
#62133=AXIS2_PLACEMENT_3D('',#97709,#70442,#70443);
#62134=AXIS2_PLACEMENT_3D('',#97711,#70444,#70445);
#62135=AXIS2_PLACEMENT_3D('',#97713,#70447,#70448);
#62136=AXIS2_PLACEMENT_3D('',#97715,#70449,#70450);
#62137=AXIS2_PLACEMENT_3D('',#97717,#70452,#70453);
#69989=DIRECTION('axis',(0.,0.,1.));
#69990=DIRECTION('refdir',(1.,0.,0.));
#69991=DIRECTION('center_axis',(0.,1.,0.));
#69992=DIRECTION('ref_axis',(1.,0.,0.));
#69993=DIRECTION('',(0.,0.,-1.));
#69994=DIRECTION('center_axis',(0.,-1.,0.));
#69995=DIRECTION('ref_axis',(1.,0.,0.));
#69996=DIRECTION('center_axis',(0.,-1.,0.));
#69997=DIRECTION('ref_axis',(1.,0.,0.));
#69998=DIRECTION('',(0.,-1.,0.));
#69999=DIRECTION('center_axis',(0.,-1.,0.));
#70000=DIRECTION('ref_axis',(1.,0.,0.));
#70001=DIRECTION('center_axis',(0.,-1.,0.));
#70002=DIRECTION('ref_axis',(1.,0.,0.));
#70003=DIRECTION('center_axis',(0.,1.,0.));
#70004=DIRECTION('ref_axis',(1.,0.,0.));
#70005=DIRECTION('',(0.,0.,1.));
#70006=DIRECTION('center_axis',(0.959768443582426,-0.280792689903722,0.));
#70007=DIRECTION('ref_axis',(-0.280792689903722,-0.959768443582426,0.));
#70008=DIRECTION('',(0.,0.,-1.));
#70009=DIRECTION('',(0.280792689903722,0.959768443582426,0.));
#70010=DIRECTION('',(0.,0.,-1.));
#70011=DIRECTION('',(-0.280792689903722,-0.959768443582426,0.));
#70012=DIRECTION('center_axis',(-0.877209189964524,0.48010835968746,0.));
#70013=DIRECTION('ref_axis',(0.48010835968746,0.877209189964524,0.));
#70014=DIRECTION('',(0.,0.,1.));
#70015=DIRECTION('',(0.48010835968746,0.877209189964524,0.));
#70016=DIRECTION('',(0.,0.,-1.));
#70017=DIRECTION('',(-0.48010835968746,-0.877209189964524,0.));
#70018=DIRECTION('',(0.,0.,-1.));
#70019=DIRECTION('center_axis',(0.,0.,-1.));
#70020=DIRECTION('ref_axis',(-0.412031471605199,-0.911169614510303,0.));
#70021=DIRECTION('center_axis',(0.,0.,1.));
#70022=DIRECTION('ref_axis',(-0.412031471605199,-0.911169614510303,0.));
#70023=DIRECTION('center_axis',(0.,0.,-1.));
#70024=DIRECTION('ref_axis',(-0.412031471605199,-0.911169614510303,0.));
#70025=DIRECTION('',(0.,0.,-1.));
#70026=DIRECTION('center_axis',(0.,0.,1.));
#70027=DIRECTION('ref_axis',(0.923879532511286,-0.38268343236509,0.));
#70028=DIRECTION('center_axis',(0.,0.,1.));
#70029=DIRECTION('ref_axis',(1.,0.,0.));
#70030=DIRECTION('center_axis',(0.,0.,1.));
#70031=DIRECTION('ref_axis',(1.,0.,0.));
#70032=DIRECTION('center_axis',(0.,0.,1.));
#70033=DIRECTION('ref_axis',(1.,0.,0.));
#70034=DIRECTION('',(0.,0.,-1.));
#70035=DIRECTION('center_axis',(0.,0.,1.));
#70036=DIRECTION('ref_axis',(1.,0.,0.));
#70037=DIRECTION('',(0.,0.,-1.));
#70038=DIRECTION('center_axis',(0.,0.,1.));
#70039=DIRECTION('ref_axis',(1.,0.,0.));
#70040=DIRECTION('',(0.,0.,1.));
#70041=DIRECTION('center_axis',(0.,0.,1.));
#70042=DIRECTION('ref_axis',(1.,0.,0.));
#70043=DIRECTION('',(0.,0.,-1.));
#70044=DIRECTION('center_axis',(0.,0.,1.));
#70045=DIRECTION('ref_axis',(1.,0.,0.));
#70046=DIRECTION('',(0.,0.,1.));
#70047=DIRECTION('center_axis',(0.,0.,1.));
#70048=DIRECTION('ref_axis',(1.,0.,0.));
#70049=DIRECTION('',(0.,0.,-1.));
#70050=DIRECTION('center_axis',(0.,0.,1.));
#70051=DIRECTION('ref_axis',(1.,0.,0.));
#70052=DIRECTION('center_axis',(0.,0.,1.));
#70053=DIRECTION('ref_axis',(1.,0.,0.));
#70054=DIRECTION('',(0.,0.,1.));
#70055=DIRECTION('center_axis',(0.,0.,1.));
#70056=DIRECTION('ref_axis',(1.,0.,0.));
#70057=DIRECTION('',(0.,0.,-1.));
#70058=DIRECTION('center_axis',(0.,0.,1.));
#70059=DIRECTION('ref_axis',(1.,0.,0.));
#70060=DIRECTION('',(0.,0.,1.));
#70061=DIRECTION('center_axis',(0.,0.,1.));
#70062=DIRECTION('ref_axis',(1.,0.,0.));
#70063=DIRECTION('',(0.,0.,-1.));
#70064=DIRECTION('center_axis',(0.,0.,1.));
#70065=DIRECTION('ref_axis',(1.,0.,0.));
#70066=DIRECTION('',(0.,0.,1.));
#70067=DIRECTION('center_axis',(0.,0.,1.));
#70068=DIRECTION('ref_axis',(1.,0.,0.));
#70069=DIRECTION('',(0.,0.,-1.));
#70070=DIRECTION('center_axis',(0.,0.,1.));
#70071=DIRECTION('ref_axis',(1.,0.,0.));
#70072=DIRECTION('',(0.,0.,1.));
#70073=DIRECTION('center_axis',(0.,0.,1.));
#70074=DIRECTION('ref_axis',(1.,0.,0.));
#70075=DIRECTION('',(0.,0.,-1.));
#70076=DIRECTION('center_axis',(0.,0.,1.));
#70077=DIRECTION('ref_axis',(1.,0.,0.));
#70078=DIRECTION('',(0.,0.,1.));
#70079=DIRECTION('center_axis',(0.,0.,1.));
#70080=DIRECTION('ref_axis',(1.,0.,0.));
#70081=DIRECTION('',(0.,0.,-1.));
#70082=DIRECTION('center_axis',(0.,0.,1.));
#70083=DIRECTION('ref_axis',(1.,0.,0.));
#70084=DIRECTION('',(0.,0.,1.));
#70085=DIRECTION('center_axis',(0.,0.,1.));
#70086=DIRECTION('ref_axis',(1.,0.,0.));
#70087=DIRECTION('',(0.,0.,-1.));
#70088=DIRECTION('center_axis',(0.,0.,1.));
#70089=DIRECTION('ref_axis',(1.,0.,0.));
#70090=DIRECTION('',(0.,0.,1.));
#70091=DIRECTION('center_axis',(0.,0.,1.));
#70092=DIRECTION('ref_axis',(1.,0.,0.));
#70093=DIRECTION('',(0.,0.,-1.));
#70094=DIRECTION('center_axis',(0.,0.,1.));
#70095=DIRECTION('ref_axis',(1.,0.,0.));
#70096=DIRECTION('',(0.,0.,1.));
#70097=DIRECTION('center_axis',(0.,0.,1.));
#70098=DIRECTION('ref_axis',(1.,0.,0.));
#70099=DIRECTION('',(0.,0.,-1.));
#70100=DIRECTION('center_axis',(0.,0.,1.));
#70101=DIRECTION('ref_axis',(1.,0.,0.));
#70102=DIRECTION('',(0.,0.,1.));
#70103=DIRECTION('center_axis',(0.,0.,1.));
#70104=DIRECTION('ref_axis',(1.,0.,0.));
#70105=DIRECTION('',(0.,0.,-1.));
#70106=DIRECTION('center_axis',(0.,0.,1.));
#70107=DIRECTION('ref_axis',(1.,0.,0.));
#70108=DIRECTION('',(0.,0.,1.));
#70109=DIRECTION('center_axis',(0.,0.,1.));
#70110=DIRECTION('ref_axis',(1.,0.,0.));
#70111=DIRECTION('',(0.,0.,-1.));
#70112=DIRECTION('center_axis',(0.,0.,1.));
#70113=DIRECTION('ref_axis',(1.,0.,0.));
#70114=DIRECTION('',(0.,0.,1.));
#70115=DIRECTION('center_axis',(0.,0.,1.));
#70116=DIRECTION('ref_axis',(1.,0.,0.));
#70117=DIRECTION('',(0.,0.,-1.));
#70118=DIRECTION('center_axis',(0.,0.,1.));
#70119=DIRECTION('ref_axis',(1.,0.,0.));
#70120=DIRECTION('',(0.,0.,1.));
#70121=DIRECTION('center_axis',(0.,0.,1.));
#70122=DIRECTION('ref_axis',(1.,0.,0.));
#70123=DIRECTION('',(0.,0.,-1.));
#70124=DIRECTION('center_axis',(0.,0.,1.));
#70125=DIRECTION('ref_axis',(1.,0.,0.));
#70126=DIRECTION('',(0.,0.,1.));
#70127=DIRECTION('center_axis',(0.,0.,1.));
#70128=DIRECTION('ref_axis',(1.,0.,0.));
#70129=DIRECTION('center_axis',(0.779255710620635,-0.626706101346659,0.));
#70130=DIRECTION('ref_axis',(-0.626706101346659,-0.779255710620635,0.));
#70131=DIRECTION('',(0.626706101346659,0.779255710620635,0.));
#70132=DIRECTION('',(0.,0.,-1.));
#70133=DIRECTION('',(-0.626706101346659,-0.779255710620635,0.));
#70134=DIRECTION('center_axis',(-0.626706101346659,0.779255710620635,0.));
#70135=DIRECTION('ref_axis',(0.779255710620635,0.626706101346659,0.));
#70136=DIRECTION('',(0.779255710620635,0.626706101346659,0.));
#70137=DIRECTION('',(0.,0.,-1.));
#70138=DIRECTION('',(-0.779255710620635,-0.626706101346659,0.));
#70139=DIRECTION('',(0.,0.,-1.));
#70140=DIRECTION('center_axis',(0.,0.,-1.));
#70141=DIRECTION('ref_axis',(-0.729356958914127,-0.684133339695952,0.));
#70142=DIRECTION('center_axis',(0.,0.,1.));
#70143=DIRECTION('ref_axis',(-0.729356958914127,-0.684133339695952,0.));
#70144=DIRECTION('center_axis',(0.,0.,-1.));
#70145=DIRECTION('ref_axis',(-0.729356958914127,-0.684133339695952,0.));
#70146=DIRECTION('',(0.,0.,-1.));
#70147=DIRECTION('center_axis',(0.,0.,1.));
#70148=DIRECTION('ref_axis',(0.707106781186547,-0.707106781186548,0.));
#70149=DIRECTION('center_axis',(0.48010835968746,-0.877209189964524,0.));
#70150=DIRECTION('ref_axis',(-0.877209189964524,-0.48010835968746,0.));
#70151=DIRECTION('',(0.877209189964524,0.48010835968746,0.));
#70152=DIRECTION('',(0.,0.,-1.));
#70153=DIRECTION('',(-0.877209189964524,-0.48010835968746,0.));
#70154=DIRECTION('center_axis',(-0.280792689903721,0.959768443582426,0.));
#70155=DIRECTION('ref_axis',(0.959768443582426,0.280792689903721,0.));
#70156=DIRECTION('',(0.959768443582426,0.280792689903721,0.));
#70157=DIRECTION('',(0.,0.,-1.));
#70158=DIRECTION('',(-0.959768443582426,-0.280792689903721,0.));
#70159=DIRECTION('',(0.,0.,-1.));
#70160=DIRECTION('center_axis',(0.,0.,-1.));
#70161=DIRECTION('ref_axis',(-0.935644460865676,-0.35294396559706,0.));
#70162=DIRECTION('center_axis',(0.,0.,1.));
#70163=DIRECTION('ref_axis',(-0.935644460865676,-0.35294396559706,0.));
#70164=DIRECTION('center_axis',(0.,0.,-1.));
#70165=DIRECTION('ref_axis',(-0.935644460865676,-0.35294396559706,0.));
#70166=DIRECTION('',(0.,0.,-1.));
#70167=DIRECTION('center_axis',(0.,0.,1.));
#70168=DIRECTION('ref_axis',(0.38268343236509,-0.923879532511287,0.));
#70169=DIRECTION('center_axis',(0.107868863184986,-0.994165131331399,0.));
#70170=DIRECTION('ref_axis',(-0.994165131331399,-0.107868863184986,0.));
#70171=DIRECTION('',(0.994165131331399,0.107868863184986,0.));
#70172=DIRECTION('',(0.,0.,-1.));
#70173=DIRECTION('',(-0.994165131331399,-0.107868863184986,0.));
#70174=DIRECTION('center_axis',(0.107868863184987,0.994165131331399,0.));
#70175=DIRECTION('ref_axis',(0.994165131331399,-0.107868863184987,0.));
#70176=DIRECTION('',(0.994165131331399,-0.107868863184987,0.));
#70177=DIRECTION('',(0.,0.,-1.));
#70178=DIRECTION('',(-0.994165131331399,0.107868863184987,0.));
#70179=DIRECTION('',(0.,0.,-1.));
#70180=DIRECTION('center_axis',(0.,0.,-1.));
#70181=DIRECTION('ref_axis',(-0.999488575288585,0.0319779278189696,0.));
#70182=DIRECTION('center_axis',(0.,0.,1.));
#70183=DIRECTION('ref_axis',(-0.999488575288585,0.0319779278189696,0.));
#70184=DIRECTION('center_axis',(0.,0.,-1.));
#70185=DIRECTION('ref_axis',(-0.999488575288585,0.0319779278189696,0.));
#70186=DIRECTION('',(0.,0.,-1.));
#70187=DIRECTION('center_axis',(0.,0.,1.));
#70188=DIRECTION('ref_axis',(-1.83697019872103E-16,-1.,0.));
#70189=DIRECTION('center_axis',(-0.280792689903722,-0.959768443582426,0.));
#70190=DIRECTION('ref_axis',(-0.959768443582426,0.280792689903722,0.));
#70191=DIRECTION('',(0.959768443582426,-0.280792689903722,0.));
#70192=DIRECTION('',(0.,0.,-1.));
#70193=DIRECTION('',(-0.959768443582426,0.280792689903722,0.));
#70194=DIRECTION('center_axis',(0.48010835968746,0.877209189964524,0.));
#70195=DIRECTION('ref_axis',(0.877209189964524,-0.48010835968746,0.));
#70196=DIRECTION('',(0.877209189964524,-0.48010835968746,0.));
#70197=DIRECTION('',(0.,0.,-1.));
#70198=DIRECTION('',(-0.877209189964524,0.48010835968746,0.));
#70199=DIRECTION('',(0.,0.,-1.));
#70200=DIRECTION('center_axis',(0.,0.,-1.));
#70201=DIRECTION('ref_axis',(-0.911169614510303,0.412031471605199,0.));
#70202=DIRECTION('center_axis',(0.,0.,1.));
#70203=DIRECTION('ref_axis',(-0.911169614510303,0.412031471605199,0.));
#70204=DIRECTION('center_axis',(0.,0.,-1.));
#70205=DIRECTION('ref_axis',(-0.911169614510303,0.412031471605199,0.));
#70206=DIRECTION('',(0.,0.,-1.));
#70207=DIRECTION('center_axis',(0.,0.,1.));
#70208=DIRECTION('ref_axis',(-0.38268343236509,-0.923879532511286,0.));
#70209=DIRECTION('center_axis',(-0.626706101346659,-0.779255710620635,0.));
#70210=DIRECTION('ref_axis',(-0.779255710620635,0.626706101346659,0.));
#70211=DIRECTION('',(0.779255710620635,-0.626706101346659,0.));
#70212=DIRECTION('',(0.,0.,-1.));
#70213=DIRECTION('',(-0.779255710620635,0.626706101346659,0.));
#70214=DIRECTION('center_axis',(0.779255710620635,0.626706101346659,0.));
#70215=DIRECTION('ref_axis',(0.626706101346659,-0.779255710620635,0.));
#70216=DIRECTION('',(0.626706101346659,-0.779255710620635,0.));
#70217=DIRECTION('',(0.,0.,-1.));
#70218=DIRECTION('',(-0.626706101346659,0.779255710620635,0.));
#70219=DIRECTION('',(0.,0.,-1.));
#70220=DIRECTION('center_axis',(0.,0.,-1.));
#70221=DIRECTION('ref_axis',(-0.684133339695952,0.729356958914127,0.));
#70222=DIRECTION('center_axis',(0.,0.,1.));
#70223=DIRECTION('ref_axis',(-0.684133339695952,0.729356958914127,0.));
#70224=DIRECTION('center_axis',(0.,0.,-1.));
#70225=DIRECTION('ref_axis',(-0.684133339695952,0.729356958914127,0.));
#70226=DIRECTION('',(0.,0.,-1.));
#70227=DIRECTION('center_axis',(0.,0.,1.));
#70228=DIRECTION('ref_axis',(-0.707106781186548,-0.707106781186547,0.));
#70229=DIRECTION('center_axis',(-0.877209189964525,-0.480108359687459,0.));
#70230=DIRECTION('ref_axis',(-0.480108359687459,0.877209189964524,0.));
#70231=DIRECTION('',(0.480108359687459,-0.877209189964524,0.));
#70232=DIRECTION('',(0.,0.,-1.));
#70233=DIRECTION('',(-0.480108359687459,0.877209189964524,0.));
#70234=DIRECTION('center_axis',(0.959768443582426,0.280792689903721,0.));
#70235=DIRECTION('ref_axis',(0.280792689903721,-0.959768443582426,0.));
#70236=DIRECTION('',(0.280792689903721,-0.959768443582426,0.));
#70237=DIRECTION('',(0.,0.,-1.));
#70238=DIRECTION('',(-0.280792689903721,0.959768443582426,0.));
#70239=DIRECTION('',(0.,0.,-1.));
#70240=DIRECTION('center_axis',(0.,0.,-1.));
#70241=DIRECTION('ref_axis',(-0.35294396559706,0.935644460865676,0.));
#70242=DIRECTION('center_axis',(0.,0.,1.));
#70243=DIRECTION('ref_axis',(-0.35294396559706,0.935644460865676,0.));
#70244=DIRECTION('center_axis',(0.,0.,-1.));
#70245=DIRECTION('ref_axis',(-0.35294396559706,0.935644460865676,0.));
#70246=DIRECTION('',(0.,0.,-1.));
#70247=DIRECTION('center_axis',(0.,0.,1.));
#70248=DIRECTION('ref_axis',(-0.923879532511287,-0.38268343236509,0.));
#70249=DIRECTION('center_axis',(-0.994165131331399,-0.107868863184986,0.));
#70250=DIRECTION('ref_axis',(-0.107868863184986,0.994165131331399,0.));
#70251=DIRECTION('',(0.107868863184986,-0.994165131331399,0.));
#70252=DIRECTION('',(0.,0.,-1.));
#70253=DIRECTION('',(-0.107868863184986,0.994165131331399,0.));
#70254=DIRECTION('center_axis',(0.994165131331399,-0.107868863184987,0.));
#70255=DIRECTION('ref_axis',(-0.107868863184987,-0.994165131331399,0.));
#70256=DIRECTION('',(-0.107868863184987,-0.994165131331399,0.));
#70257=DIRECTION('',(0.,0.,-1.));
#70258=DIRECTION('',(0.107868863184987,0.994165131331399,0.));
#70259=DIRECTION('',(0.,0.,-1.));
#70260=DIRECTION('center_axis',(0.,0.,-1.));
#70261=DIRECTION('ref_axis',(0.0319779278189696,0.999488575288585,0.));
#70262=DIRECTION('center_axis',(0.,0.,1.));
#70263=DIRECTION('ref_axis',(0.0319779278189696,0.999488575288585,0.));
#70264=DIRECTION('center_axis',(0.,0.,-1.));
#70265=DIRECTION('ref_axis',(0.0319779278189696,0.999488575288585,0.));
#70266=DIRECTION('',(0.,0.,-1.));
#70267=DIRECTION('center_axis',(0.,0.,1.));
#70268=DIRECTION('ref_axis',(-1.,1.22464679914735E-16,0.));
#70269=DIRECTION('center_axis',(-0.959768443582426,0.280792689903721,0.));
#70270=DIRECTION('ref_axis',(0.280792689903721,0.959768443582426,0.));
#70271=DIRECTION('',(-0.280792689903721,-0.959768443582426,0.));
#70272=DIRECTION('',(0.,0.,-1.));
#70273=DIRECTION('',(0.280792689903721,0.959768443582426,0.));
#70274=DIRECTION('center_axis',(0.877209189964524,-0.48010835968746,0.));
#70275=DIRECTION('ref_axis',(-0.48010835968746,-0.877209189964524,0.));
#70276=DIRECTION('',(-0.48010835968746,-0.877209189964524,0.));
#70277=DIRECTION('',(0.,0.,-1.));
#70278=DIRECTION('',(0.48010835968746,0.877209189964524,0.));
#70279=DIRECTION('',(0.,0.,-1.));
#70280=DIRECTION('center_axis',(0.,0.,-1.));
#70281=DIRECTION('ref_axis',(0.412031471605198,0.911169614510303,0.));
#70282=DIRECTION('center_axis',(0.,0.,1.));
#70283=DIRECTION('ref_axis',(0.412031471605198,0.911169614510303,0.));
#70284=DIRECTION('center_axis',(0.,0.,-1.));
#70285=DIRECTION('ref_axis',(0.412031471605198,0.911169614510303,0.));
#70286=DIRECTION('',(0.,0.,-1.));
#70287=DIRECTION('center_axis',(0.,0.,1.));
#70288=DIRECTION('ref_axis',(-0.923879532511287,0.38268343236509,0.));
#70289=DIRECTION('center_axis',(-0.779255710620635,0.626706101346659,0.));
#70290=DIRECTION('ref_axis',(0.626706101346659,0.779255710620635,0.));
#70291=DIRECTION('',(-0.626706101346659,-0.779255710620635,0.));
#70292=DIRECTION('',(0.,0.,-1.));
#70293=DIRECTION('',(0.626706101346659,0.779255710620635,0.));
#70294=DIRECTION('center_axis',(0.626706101346659,-0.779255710620635,0.));
#70295=DIRECTION('ref_axis',(-0.779255710620635,-0.626706101346659,0.));
#70296=DIRECTION('',(-0.779255710620635,-0.626706101346659,0.));
#70297=DIRECTION('',(0.,0.,-1.));
#70298=DIRECTION('',(0.779255710620635,0.626706101346659,0.));
#70299=DIRECTION('',(0.,0.,-1.));
#70300=DIRECTION('center_axis',(0.,0.,-1.));
#70301=DIRECTION('ref_axis',(0.729356958914127,0.684133339695952,0.));
#70302=DIRECTION('center_axis',(0.,0.,1.));
#70303=DIRECTION('ref_axis',(0.729356958914127,0.684133339695952,0.));
#70304=DIRECTION('center_axis',(0.,0.,-1.));
#70305=DIRECTION('ref_axis',(0.729356958914127,0.684133339695952,0.));
#70306=DIRECTION('',(0.,0.,-1.));
#70307=DIRECTION('center_axis',(0.,0.,1.));
#70308=DIRECTION('ref_axis',(-0.707106781186547,0.707106781186548,0.));
#70309=DIRECTION('center_axis',(-0.480108359687459,0.877209189964524,0.));
#70310=DIRECTION('ref_axis',(0.877209189964524,0.480108359687459,0.));
#70311=DIRECTION('',(-0.877209189964524,-0.480108359687459,0.));
#70312=DIRECTION('',(0.,0.,-1.));
#70313=DIRECTION('',(0.877209189964524,0.480108359687459,0.));
#70314=DIRECTION('center_axis',(0.280792689903721,-0.959768443582426,0.));
#70315=DIRECTION('ref_axis',(-0.959768443582426,-0.280792689903721,0.));
#70316=DIRECTION('',(-0.959768443582426,-0.280792689903721,0.));
#70317=DIRECTION('',(0.,0.,-1.));
#70318=DIRECTION('',(0.959768443582426,0.280792689903721,0.));
#70319=DIRECTION('',(0.,0.,-1.));
#70320=DIRECTION('center_axis',(0.,0.,-1.));
#70321=DIRECTION('ref_axis',(0.935644460865676,0.35294396559706,0.));
#70322=DIRECTION('center_axis',(0.,0.,1.));
#70323=DIRECTION('ref_axis',(0.935644460865676,0.35294396559706,0.));
#70324=DIRECTION('center_axis',(0.,0.,-1.));
#70325=DIRECTION('ref_axis',(0.935644460865676,0.35294396559706,0.));
#70326=DIRECTION('',(0.,0.,-1.));
#70327=DIRECTION('center_axis',(0.,0.,1.));
#70328=DIRECTION('ref_axis',(-0.38268343236509,0.923879532511287,0.));
#70329=DIRECTION('center_axis',(-0.107868863184986,0.994165131331399,0.));
#70330=DIRECTION('ref_axis',(0.994165131331399,0.107868863184986,0.));
#70331=DIRECTION('',(-0.994165131331399,-0.107868863184986,0.));
#70332=DIRECTION('',(0.,0.,-1.));
#70333=DIRECTION('',(0.994165131331399,0.107868863184986,0.));
#70334=DIRECTION('center_axis',(-0.107868863184987,-0.994165131331399,0.));
#70335=DIRECTION('ref_axis',(-0.994165131331399,0.107868863184987,0.));
#70336=DIRECTION('',(-0.994165131331399,0.107868863184987,0.));
#70337=DIRECTION('',(0.,0.,-1.));
#70338=DIRECTION('',(0.994165131331399,-0.107868863184987,0.));
#70339=DIRECTION('',(0.,0.,-1.));
#70340=DIRECTION('center_axis',(0.,0.,-1.));
#70341=DIRECTION('ref_axis',(0.999488575288585,-0.0319779278189695,0.));
#70342=DIRECTION('center_axis',(0.,0.,1.));
#70343=DIRECTION('ref_axis',(0.999488575288585,-0.0319779278189695,0.));
#70344=DIRECTION('center_axis',(0.,0.,-1.));
#70345=DIRECTION('ref_axis',(0.999488575288585,-0.0319779278189695,0.));
#70346=DIRECTION('',(0.,0.,-1.));
#70347=DIRECTION('center_axis',(0.,0.,1.));
#70348=DIRECTION('ref_axis',(6.12323399573677E-17,1.,0.));
#70349=DIRECTION('center_axis',(0.280792689903721,0.959768443582426,0.));
#70350=DIRECTION('ref_axis',(0.959768443582426,-0.280792689903721,0.));
#70351=DIRECTION('',(-0.959768443582426,0.280792689903721,0.));
#70352=DIRECTION('',(0.,0.,-1.));
#70353=DIRECTION('',(0.959768443582426,-0.280792689903721,0.));
#70354=DIRECTION('center_axis',(-0.48010835968746,-0.877209189964524,0.));
#70355=DIRECTION('ref_axis',(-0.877209189964524,0.480108359687459,0.));
#70356=DIRECTION('',(-0.877209189964524,0.480108359687459,0.));
#70357=DIRECTION('',(0.,0.,-1.));
#70358=DIRECTION('',(0.877209189964524,-0.480108359687459,0.));
#70359=DIRECTION('',(0.,0.,-1.));
#70360=DIRECTION('center_axis',(0.,0.,-1.));
#70361=DIRECTION('ref_axis',(0.911169614510303,-0.412031471605198,0.));
#70362=DIRECTION('center_axis',(0.,0.,1.));
#70363=DIRECTION('ref_axis',(0.911169614510303,-0.412031471605198,0.));
#70364=DIRECTION('center_axis',(0.,0.,-1.));
#70365=DIRECTION('ref_axis',(0.911169614510303,-0.412031471605198,0.));
#70366=DIRECTION('',(0.,0.,-1.));
#70367=DIRECTION('center_axis',(0.,0.,1.));
#70368=DIRECTION('ref_axis',(0.38268343236509,0.923879532511287,0.));
#70369=DIRECTION('center_axis',(0.626706101346659,0.779255710620635,0.));
#70370=DIRECTION('ref_axis',(0.779255710620635,-0.626706101346659,0.));
#70371=DIRECTION('',(-0.779255710620635,0.626706101346659,0.));
#70372=DIRECTION('',(0.,0.,-1.));
#70373=DIRECTION('',(0.779255710620635,-0.626706101346659,0.));
#70374=DIRECTION('center_axis',(-0.779255710620635,-0.626706101346659,0.));
#70375=DIRECTION('ref_axis',(-0.626706101346659,0.779255710620635,0.));
#70376=DIRECTION('',(-0.626706101346659,0.779255710620635,0.));
#70377=DIRECTION('',(0.,0.,-1.));
#70378=DIRECTION('',(0.626706101346659,-0.779255710620635,0.));
#70379=DIRECTION('',(0.,0.,-1.));
#70380=DIRECTION('center_axis',(0.,0.,-1.));
#70381=DIRECTION('ref_axis',(0.684133339695952,-0.729356958914127,0.));
#70382=DIRECTION('center_axis',(0.,0.,1.));
#70383=DIRECTION('ref_axis',(0.684133339695952,-0.729356958914127,0.));
#70384=DIRECTION('center_axis',(0.,0.,-1.));
#70385=DIRECTION('ref_axis',(0.684133339695952,-0.729356958914127,0.));
#70386=DIRECTION('',(0.,0.,-1.));
#70387=DIRECTION('center_axis',(0.,0.,1.));
#70388=DIRECTION('ref_axis',(0.707106781186548,0.707106781186548,0.));
#70389=DIRECTION('center_axis',(0.877209189964524,0.480108359687459,0.));
#70390=DIRECTION('ref_axis',(0.480108359687459,-0.877209189964524,0.));
#70391=DIRECTION('',(-0.480108359687459,0.877209189964524,0.));
#70392=DIRECTION('',(0.,0.,-1.));
#70393=DIRECTION('',(0.480108359687459,-0.877209189964524,0.));
#70394=DIRECTION('center_axis',(-0.959768443582426,-0.280792689903721,0.));
#70395=DIRECTION('ref_axis',(-0.280792689903721,0.959768443582426,0.));
#70396=DIRECTION('',(-0.280792689903721,0.959768443582426,0.));
#70397=DIRECTION('',(0.,0.,-1.));
#70398=DIRECTION('',(0.280792689903721,-0.959768443582426,0.));
#70399=DIRECTION('',(0.,0.,-1.));
#70400=DIRECTION('center_axis',(0.,0.,-1.));
#70401=DIRECTION('ref_axis',(0.35294396559706,-0.935644460865676,0.));
#70402=DIRECTION('center_axis',(0.,0.,1.));
#70403=DIRECTION('ref_axis',(0.35294396559706,-0.935644460865676,0.));
#70404=DIRECTION('center_axis',(0.,0.,-1.));
#70405=DIRECTION('ref_axis',(0.35294396559706,-0.935644460865676,0.));
#70406=DIRECTION('',(0.,0.,-1.));
#70407=DIRECTION('center_axis',(0.,0.,1.));
#70408=DIRECTION('ref_axis',(0.923879532511287,0.38268343236509,0.));
#70409=DIRECTION('center_axis',(-0.994165131331399,0.107868863184986,0.));
#70410=DIRECTION('ref_axis',(0.107868863184986,0.994165131331399,0.));
#70411=DIRECTION('',(0.107868863184986,0.994165131331399,0.));
#70412=DIRECTION('',(0.,0.,-1.));
#70413=DIRECTION('',(-0.107868863184986,-0.994165131331399,0.));
#70414=DIRECTION('',(0.,0.,-1.));
#70415=DIRECTION('center_axis',(0.,0.,-1.));
#70416=DIRECTION('ref_axis',(-0.0319779278189694,-0.999488575288585,0.));
#70417=DIRECTION('center_axis',(0.,0.,1.));
#70418=DIRECTION('ref_axis',(-0.0319779278189694,-0.999488575288585,0.));
#70419=DIRECTION('center_axis',(0.,0.,-1.));
#70420=DIRECTION('ref_axis',(-0.0319779278189694,-0.999488575288585,0.));
#70421=DIRECTION('',(0.,0.,-1.));
#70422=DIRECTION('',(0.,0.,-1.));
#70423=DIRECTION('center_axis',(0.994165131331399,0.107868863184986,0.));
#70424=DIRECTION('ref_axis',(0.107868863184986,-0.994165131331399,0.));
#70425=DIRECTION('',(-0.107868863184986,0.994165131331399,0.));
#70426=DIRECTION('',(0.107868863184986,-0.994165131331399,0.));
#70427=DIRECTION('center_axis',(0.,0.,1.));
#70428=DIRECTION('ref_axis',(1.,0.,0.));
#70429=DIRECTION('center_axis',(0.,0.,1.));
#70430=DIRECTION('ref_axis',(1.,0.,0.));
#70431=DIRECTION('center_axis',(0.,0.,1.));
#70432=DIRECTION('ref_axis',(1.,0.,0.));
#70433=DIRECTION('',(0.,0.,-1.));
#70434=DIRECTION('center_axis',(0.,0.,1.));
#70435=DIRECTION('ref_axis',(1.,0.,0.));
#70436=DIRECTION('center_axis',(0.,0.,-1.));
#70437=DIRECTION('ref_axis',(-1.,0.,0.));
#70438=DIRECTION('center_axis',(0.,0.,-1.));
#70439=DIRECTION('ref_axis',(-1.,0.,0.));
#70440=DIRECTION('center_axis',(0.,0.,1.));
#70441=DIRECTION('ref_axis',(1.,0.,0.));
#70442=DIRECTION('center_axis',(0.,0.,1.));
#70443=DIRECTION('ref_axis',(1.,0.,0.));
#70444=DIRECTION('center_axis',(0.,0.,1.));
#70445=DIRECTION('ref_axis',(1.,0.,0.));
#70446=DIRECTION('',(0.,0.,-1.));
#70447=DIRECTION('center_axis',(0.,0.,-1.));
#70448=DIRECTION('ref_axis',(1.,0.,0.));
#70449=DIRECTION('center_axis',(0.,0.,1.));
#70450=DIRECTION('ref_axis',(1.,0.,0.));
#70451=DIRECTION('',(-0.707106781186547,-8.65956056235493E-17,-0.707106781186547));
#70452=DIRECTION('center_axis',(0.,0.,1.));
#70453=DIRECTION('ref_axis',(1.,0.,0.));
#92656=CARTESIAN_POINT('',(0.,0.,0.));
#92657=CARTESIAN_POINT('Origin',(110.,20.4,33.3));
#92658=CARTESIAN_POINT('',(110.7,20.4,34.0826237921249));
#92659=CARTESIAN_POINT('',(110.7,20.4,32.5173762078751));
#92660=CARTESIAN_POINT('',(110.7,20.4,30.4));
#92661=CARTESIAN_POINT('Origin',(110.,20.4,33.3));
#92662=CARTESIAN_POINT('Origin',(110.,22.5,33.3));
#92663=CARTESIAN_POINT('',(110.,22.5,34.35));
#92664=CARTESIAN_POINT('',(108.95,22.3757856437444,33.3));
#92665=CARTESIAN_POINT('Ctrl Pts',(110.,22.5,34.35));
#92666=CARTESIAN_POINT('Ctrl Pts',(109.867639766981,22.5,34.35));
#92667=CARTESIAN_POINT('Ctrl Pts',(109.72678604534,22.4935734225297,34.3234481778509));
#92668=CARTESIAN_POINT('Ctrl Pts',(109.46822707977,22.470354072227,34.2161384098672));
#92669=CARTESIAN_POINT('Ctrl Pts',(109.350482714578,22.4538755915385,34.1354069550695));
#92670=CARTESIAN_POINT('Ctrl Pts',(109.164583259651,22.4227775468468,33.9495075001425));
#92671=CARTESIAN_POINT('Ctrl Pts',(109.083859447964,22.4060986376458,33.8317672389861));
#92672=CARTESIAN_POINT('Ctrl Pts',(108.97655524524,22.382417098112,33.5732227222323));
#92673=CARTESIAN_POINT('Ctrl Pts',(108.95,22.3757856437444,33.4323741679718));
#92674=CARTESIAN_POINT('Ctrl Pts',(108.95,22.3757856437444,33.3));
#92675=CARTESIAN_POINT('',(110.,22.5,32.25));
#92676=CARTESIAN_POINT('Ctrl Pts',(110.,22.5,32.25));
#92677=CARTESIAN_POINT('Ctrl Pts',(110.132360233019,22.5,32.25));
#92678=CARTESIAN_POINT('Ctrl Pts',(110.27321395466,22.4935734225297,32.2765518221491));
#92679=CARTESIAN_POINT('Ctrl Pts',(110.53177292023,22.470354072227,32.3838615901328));
#92680=CARTESIAN_POINT('Ctrl Pts',(110.649517285422,22.4538755915385,32.4645930449305));
#92681=CARTESIAN_POINT('Ctrl Pts',(110.835416740349,22.4227775468468,32.6504924998574));
#92682=CARTESIAN_POINT('Ctrl Pts',(110.916140552036,22.4060986376458,32.7682327610139));
#92683=CARTESIAN_POINT('Ctrl Pts',(111.02344475476,22.382417098112,33.0267772777677));
#92684=CARTESIAN_POINT('Ctrl Pts',(111.05,22.3757856437444,33.1676258320282));
#92685=CARTESIAN_POINT('Ctrl Pts',(111.05,22.3757856437444,33.3));
#92686=CARTESIAN_POINT('Ctrl Pts',(111.05,22.3757856437444,33.4323741679718));
#92687=CARTESIAN_POINT('Ctrl Pts',(111.02344475476,22.382417098112,33.5732227222323));
#92688=CARTESIAN_POINT('Ctrl Pts',(110.916140552036,22.4060986376458,33.8317672389861));
#92689=CARTESIAN_POINT('Ctrl Pts',(110.835416740349,22.4227775468468,33.9495075001425));
#92690=CARTESIAN_POINT('Ctrl Pts',(110.649517285422,22.4538755915385,34.1354069550695));
#92691=CARTESIAN_POINT('Ctrl Pts',(110.53177292023,22.470354072227,34.2161384098672));
#92692=CARTESIAN_POINT('Ctrl Pts',(110.27321395466,22.4935734225297,34.3234481778509));
#92693=CARTESIAN_POINT('Ctrl Pts',(110.132360233019,22.5,34.35));
#92694=CARTESIAN_POINT('Ctrl Pts',(110.,22.5,34.35));
#92695=CARTESIAN_POINT('Ctrl Pts',(108.95,22.3757856437444,33.3));
#92696=CARTESIAN_POINT('Ctrl Pts',(108.95,22.3757856437444,33.1676258320282));
#92697=CARTESIAN_POINT('Ctrl Pts',(108.97655524524,22.382417098112,33.0267772777677));
#92698=CARTESIAN_POINT('Ctrl Pts',(109.083859447964,22.4060986376458,32.7682327610139));
#92699=CARTESIAN_POINT('Ctrl Pts',(109.164583259651,22.4227775468468,32.6504924998574));
#92700=CARTESIAN_POINT('Ctrl Pts',(109.350482714578,22.4538755915385,32.4645930449305));
#92701=CARTESIAN_POINT('Ctrl Pts',(109.46822707977,22.470354072227,32.3838615901328));
#92702=CARTESIAN_POINT('Ctrl Pts',(109.72678604534,22.4935734225297,32.2765518221491));
#92703=CARTESIAN_POINT('Ctrl Pts',(109.867639766981,22.5,32.25));
#92704=CARTESIAN_POINT('Ctrl Pts',(110.,22.5,32.25));
#92705=CARTESIAN_POINT('',(108.95,20.4,33.3));
#92706=CARTESIAN_POINT('',(108.95,22.5,33.3));
#92707=CARTESIAN_POINT('',(109.3,20.4,32.5173762078751));
#92708=CARTESIAN_POINT('Origin',(110.,20.4,33.3));
#92709=CARTESIAN_POINT('Ctrl Pts',(110.7,20.4,32.5173762078751));
#92710=CARTESIAN_POINT('Ctrl Pts',(110.615542349369,20.424633481434,32.4418349886629));
#92711=CARTESIAN_POINT('Ctrl Pts',(110.514132074769,20.4491019379392,32.376755439497));
#92712=CARTESIAN_POINT('Ctrl Pts',(110.274969793834,20.4882751681165,32.2770312340585));
#92713=CARTESIAN_POINT('Ctrl Pts',(110.133578485591,20.5,32.25));
#92714=CARTESIAN_POINT('Ctrl Pts',(109.866421514409,20.5,32.25));
#92715=CARTESIAN_POINT('Ctrl Pts',(109.725030206166,20.4882751681165,32.2770312340585));
#92716=CARTESIAN_POINT('Ctrl Pts',(109.485867925231,20.4491019379392,32.376755439497));
#92717=CARTESIAN_POINT('Ctrl Pts',(109.384457650631,20.424633481434,32.4418349886629));
#92718=CARTESIAN_POINT('Ctrl Pts',(109.3,20.4,32.5173762078751));
#92719=CARTESIAN_POINT('',(109.3,20.4,34.0826237921249));
#92720=CARTESIAN_POINT('Ctrl Pts',(109.3,20.4,34.0826237921249));
#92721=CARTESIAN_POINT('Ctrl Pts',(109.384457650631,20.424633481434,34.1581650113371));
#92722=CARTESIAN_POINT('Ctrl Pts',(109.485867925231,20.4491019379392,34.223244560503));
#92723=CARTESIAN_POINT('Ctrl Pts',(109.725030206166,20.4882751681165,34.3229687659415));
#92724=CARTESIAN_POINT('Ctrl Pts',(109.866421514409,20.5,34.35));
#92725=CARTESIAN_POINT('Ctrl Pts',(110.133578485591,20.5,34.35));
#92726=CARTESIAN_POINT('Ctrl Pts',(110.274969793834,20.4882751681165,34.3229687659415));
#92727=CARTESIAN_POINT('Ctrl Pts',(110.514132074769,20.4491019379392,34.223244560503));
#92728=CARTESIAN_POINT('Ctrl Pts',(110.615542349369,20.424633481434,34.1581650113371));
#92729=CARTESIAN_POINT('Ctrl Pts',(110.7,20.4,34.0826237921249));
#92730=CARTESIAN_POINT('Origin',(110.,20.4,33.3));
#92731=CARTESIAN_POINT('Origin',(110.,20.4,33.3));
#92732=CARTESIAN_POINT('',(109.3,20.4,30.4));
#92733=CARTESIAN_POINT('Origin',(109.09444357506,14.9047467694467,31.));
#92734=CARTESIAN_POINT('',(109.052324671575,14.7607815029093,31.));
#92735=CARTESIAN_POINT('',(109.052324671575,14.7607815029093,26.));
#92736=CARTESIAN_POINT('',(109.052324671575,14.7607815029093,28.9));
#92737=CARTESIAN_POINT('',(108.944564725307,14.3924507036097,31.));
#92738=CARTESIAN_POINT('',(108.944564725307,14.3924507036097,31.));
#92739=CARTESIAN_POINT('',(108.944564725307,14.3924507036097,26.));
#92740=CARTESIAN_POINT('',(108.944564725307,14.3924507036097,31.));
#92741=CARTESIAN_POINT('',(108.944564725307,14.3924507036097,26.));
#92742=CARTESIAN_POINT('Origin',(108.195382868896,14.702771989219,31.));
#92743=CARTESIAN_POINT('',(108.379634286055,15.0394189838697,26.));
#92744=CARTESIAN_POINT('',(108.379634286055,15.0394189838697,31.));
#92745=CARTESIAN_POINT('',(108.379634286055,15.0394189838697,28.9));
#92746=CARTESIAN_POINT('',(108.195382868896,14.702771989219,26.));
#92747=CARTESIAN_POINT('',(108.451650540008,15.1710003623644,26.));
#92748=CARTESIAN_POINT('',(108.195382868896,14.702771989219,31.));
#92749=CARTESIAN_POINT('',(108.195382868896,14.702771989219,31.));
#92750=CARTESIAN_POINT('',(108.451650540008,15.1710003623644,31.));
#92751=CARTESIAN_POINT('Ctrl Pts',(108.145858377777,13.8997367347037,31.));
#92752=CARTESIAN_POINT('Ctrl Pts',(108.145858377777,13.8997367347037,26.));
#92753=CARTESIAN_POINT('Ctrl Pts',(108.14473177199,13.9069480980004,31.));
#92754=CARTESIAN_POINT('Ctrl Pts',(108.14473177199,13.9069480980004,26.));
#92755=CARTESIAN_POINT('Ctrl Pts',(108.14253438479,13.9213259759795,31.));
#92756=CARTESIAN_POINT('Ctrl Pts',(108.14253438479,13.9213259759795,26.));
#92757=CARTESIAN_POINT('Ctrl Pts',(108.139405776934,13.9427582473116,31.));
#92758=CARTESIAN_POINT('Ctrl Pts',(108.139405776934,13.9427582473116,26.));
#92759=CARTESIAN_POINT('Ctrl Pts',(108.135569853724,13.9710650288043,31.));
#92760=CARTESIAN_POINT('Ctrl Pts',(108.135569853724,13.9710650288043,26.));
#92761=CARTESIAN_POINT('Ctrl Pts',(108.131337578061,14.005995880259,31.));
#92762=CARTESIAN_POINT('Ctrl Pts',(108.131337578061,14.005995880259,26.));
#92763=CARTESIAN_POINT('Ctrl Pts',(108.127671920245,14.0404690398857,31.));
#92764=CARTESIAN_POINT('Ctrl Pts',(108.127671920245,14.0404690398857,26.));
#92765=CARTESIAN_POINT('Ctrl Pts',(108.124576114257,14.0744781941125,31.));
#92766=CARTESIAN_POINT('Ctrl Pts',(108.124576114257,14.0744781941125,26.));
#92767=CARTESIAN_POINT('Ctrl Pts',(108.122051296587,14.1080161789411,31.));
#92768=CARTESIAN_POINT('Ctrl Pts',(108.122051296587,14.1080161789411,26.));
#92769=CARTESIAN_POINT('Ctrl Pts',(108.120094755478,14.141075848522,31.));
#92770=CARTESIAN_POINT('Ctrl Pts',(108.120094755478,14.141075848522,26.));
#92771=CARTESIAN_POINT('Ctrl Pts',(108.118699969367,14.1736486380529,31.));
#92772=CARTESIAN_POINT('Ctrl Pts',(108.118699969367,14.1736486380529,26.));
#92773=CARTESIAN_POINT('Ctrl Pts',(108.117857140196,14.2057226050197,31.));
#92774=CARTESIAN_POINT('Ctrl Pts',(108.117857140196,14.2057226050197,26.));
#92775=CARTESIAN_POINT('Ctrl Pts',(108.11755334977,14.2372805163279,31.));
#92776=CARTESIAN_POINT('Ctrl Pts',(108.11755334977,14.2372805163279,26.));
#92777=CARTESIAN_POINT('Ctrl Pts',(108.117772886125,14.2682984546298,31.));
#92778=CARTESIAN_POINT('Ctrl Pts',(108.117772886125,14.2682984546298,26.));
#92779=CARTESIAN_POINT('Ctrl Pts',(108.118496961781,14.2987431062216,31.));
#92780=CARTESIAN_POINT('Ctrl Pts',(108.118496961781,14.2987431062216,26.));
#92781=CARTESIAN_POINT('Ctrl Pts',(108.119705321862,14.3285749073991,31.));
#92782=CARTESIAN_POINT('Ctrl Pts',(108.119705321862,14.3285749073991,26.));
#92783=CARTESIAN_POINT('Ctrl Pts',(108.121378863878,14.3577546057035,31.));
#92784=CARTESIAN_POINT('Ctrl Pts',(108.121378863878,14.3577546057035,26.));
#92785=CARTESIAN_POINT('Ctrl Pts',(108.123502124645,14.3862495604353,31.));
#92786=CARTESIAN_POINT('Ctrl Pts',(108.123502124645,14.3862495604353,26.));
#92787=CARTESIAN_POINT('Ctrl Pts',(108.126065158394,14.4140388871472,31.));
#92788=CARTESIAN_POINT('Ctrl Pts',(108.126065158394,14.4140388871472,26.));
#92789=CARTESIAN_POINT('Ctrl Pts',(108.129067047035,14.4411228648582,31.));
#92790=CARTESIAN_POINT('Ctrl Pts',(108.129067047035,14.4411228648582,26.));
#92791=CARTESIAN_POINT('Ctrl Pts',(108.132512853032,14.4675164161688,31.));
#92792=CARTESIAN_POINT('Ctrl Pts',(108.132512853032,14.4675164161688,26.));
#92793=CARTESIAN_POINT('Ctrl Pts',(108.136405082654,14.4932291911838,31.));
#92794=CARTESIAN_POINT('Ctrl Pts',(108.136405082654,14.4932291911838,26.));
#92795=CARTESIAN_POINT('Ctrl Pts',(108.140736063189,14.5182483587362,31.));
#92796=CARTESIAN_POINT('Ctrl Pts',(108.140736063189,14.5182483587362,26.));
#92797=CARTESIAN_POINT('Ctrl Pts',(108.145480953033,14.5425228839262,31.));
#92798=CARTESIAN_POINT('Ctrl Pts',(108.145480953033,14.5425228839262,26.));
#92799=CARTESIAN_POINT('Ctrl Pts',(108.150587396025,14.5659407047248,31.));
#92800=CARTESIAN_POINT('Ctrl Pts',(108.150587396025,14.5659407047248,26.));
#92801=CARTESIAN_POINT('Ctrl Pts',(108.155978401035,14.5883354024226,31.));
#92802=CARTESIAN_POINT('Ctrl Pts',(108.155978401035,14.5883354024226,26.));
#92803=CARTESIAN_POINT('Ctrl Pts',(108.161565843363,14.6095165692449,31.));
#92804=CARTESIAN_POINT('Ctrl Pts',(108.161565843363,14.6095165692449,26.));
#92805=CARTESIAN_POINT('Ctrl Pts',(108.167261205399,14.6292944653163,31.));
#92806=CARTESIAN_POINT('Ctrl Pts',(108.167261205399,14.6292944653163,26.));
#92807=CARTESIAN_POINT('Ctrl Pts',(108.172986416044,14.6475048278073,31.));
#92808=CARTESIAN_POINT('Ctrl Pts',(108.172986416044,14.6475048278073,26.));
#92809=CARTESIAN_POINT('Ctrl Pts',(108.178687097234,14.6640400995864,31.));
#92810=CARTESIAN_POINT('Ctrl Pts',(108.178687097234,14.6640400995864,26.));
#92811=CARTESIAN_POINT('Ctrl Pts',(108.184331851892,14.6788459938496,31.));
#92812=CARTESIAN_POINT('Ctrl Pts',(108.184331851892,14.6788459938496,26.));
#92813=CARTESIAN_POINT('Ctrl Pts',(108.188790420063,14.6892908937643,31.));
#92814=CARTESIAN_POINT('Ctrl Pts',(108.188790420063,14.6892908937643,26.));
#92815=CARTESIAN_POINT('Ctrl Pts',(108.192099987045,14.6963371269515,31.));
#92816=CARTESIAN_POINT('Ctrl Pts',(108.192099987045,14.6963371269515,26.));
#92817=CARTESIAN_POINT('Ctrl Pts',(108.194291116197,14.7006852604777,31.));
#92818=CARTESIAN_POINT('Ctrl Pts',(108.194291116197,14.7006852604777,26.));
#92819=CARTESIAN_POINT('Ctrl Pts',(108.195382868896,14.702771989219,31.));
#92820=CARTESIAN_POINT('Ctrl Pts',(108.195382868896,14.702771989219,26.));
#92821=CARTESIAN_POINT('',(108.145858377777,13.8997367347037,31.));
#92822=CARTESIAN_POINT('Ctrl Pts',(108.195382868896,14.702771989219,31.));
#92823=CARTESIAN_POINT('Ctrl Pts',(108.194291116197,14.7006852604777,31.));
#92824=CARTESIAN_POINT('Ctrl Pts',(108.192099987045,14.6963371269515,31.));
#92825=CARTESIAN_POINT('Ctrl Pts',(108.188790420063,14.6892908937643,31.));
#92826=CARTESIAN_POINT('Ctrl Pts',(108.184331851892,14.6788459938496,31.));
#92827=CARTESIAN_POINT('Ctrl Pts',(108.178687097234,14.6640400995864,31.));
#92828=CARTESIAN_POINT('Ctrl Pts',(108.172986416044,14.6475048278073,31.));
#92829=CARTESIAN_POINT('Ctrl Pts',(108.167261205399,14.6292944653163,31.));
#92830=CARTESIAN_POINT('Ctrl Pts',(108.161565843363,14.6095165692449,31.));
#92831=CARTESIAN_POINT('Ctrl Pts',(108.155978401035,14.5883354024226,31.));
#92832=CARTESIAN_POINT('Ctrl Pts',(108.150587396025,14.5659407047248,31.));
#92833=CARTESIAN_POINT('Ctrl Pts',(108.145480953033,14.5425228839262,31.));
#92834=CARTESIAN_POINT('Ctrl Pts',(108.140736063189,14.5182483587362,31.));
#92835=CARTESIAN_POINT('Ctrl Pts',(108.136405082654,14.4932291911838,31.));
#92836=CARTESIAN_POINT('Ctrl Pts',(108.132512853032,14.4675164161688,31.));
#92837=CARTESIAN_POINT('Ctrl Pts',(108.129067047035,14.4411228648582,31.));
#92838=CARTESIAN_POINT('Ctrl Pts',(108.126065158394,14.4140388871472,31.));
#92839=CARTESIAN_POINT('Ctrl Pts',(108.123502124645,14.3862495604353,31.));
#92840=CARTESIAN_POINT('Ctrl Pts',(108.121378863878,14.3577546057035,31.));
#92841=CARTESIAN_POINT('Ctrl Pts',(108.119705321862,14.3285749073991,31.));
#92842=CARTESIAN_POINT('Ctrl Pts',(108.118496961781,14.2987431062216,31.));
#92843=CARTESIAN_POINT('Ctrl Pts',(108.117772886125,14.2682984546298,31.));
#92844=CARTESIAN_POINT('Ctrl Pts',(108.11755334977,14.2372805163279,31.));
#92845=CARTESIAN_POINT('Ctrl Pts',(108.117857140196,14.2057226050197,31.));
#92846=CARTESIAN_POINT('Ctrl Pts',(108.118699969367,14.1736486380529,31.));
#92847=CARTESIAN_POINT('Ctrl Pts',(108.120094755478,14.141075848522,31.));
#92848=CARTESIAN_POINT('Ctrl Pts',(108.122051296587,14.1080161789411,31.));
#92849=CARTESIAN_POINT('Ctrl Pts',(108.124576114257,14.0744781941125,31.));
#92850=CARTESIAN_POINT('Ctrl Pts',(108.127671920245,14.0404690398857,31.));
#92851=CARTESIAN_POINT('Ctrl Pts',(108.131337578061,14.005995880259,31.));
#92852=CARTESIAN_POINT('Ctrl Pts',(108.135569853724,13.9710650288043,31.));
#92853=CARTESIAN_POINT('Ctrl Pts',(108.139405776934,13.9427582473116,31.));
#92854=CARTESIAN_POINT('Ctrl Pts',(108.14253438479,13.9213259759795,31.));
#92855=CARTESIAN_POINT('Ctrl Pts',(108.14473177199,13.9069480980004,31.));
#92856=CARTESIAN_POINT('Ctrl Pts',(108.145858377777,13.8997367347037,31.));
#92857=CARTESIAN_POINT('',(108.145858377777,13.8997367347037,26.));
#92858=CARTESIAN_POINT('Ctrl Pts',(108.145858377777,13.8997367347037,26.));
#92859=CARTESIAN_POINT('Ctrl Pts',(108.14473177199,13.9069480980004,26.));
#92860=CARTESIAN_POINT('Ctrl Pts',(108.14253438479,13.9213259759795,26.));
#92861=CARTESIAN_POINT('Ctrl Pts',(108.139405776934,13.9427582473116,26.));
#92862=CARTESIAN_POINT('Ctrl Pts',(108.135569853724,13.9710650288043,26.));
#92863=CARTESIAN_POINT('Ctrl Pts',(108.131337578061,14.005995880259,26.));
#92864=CARTESIAN_POINT('Ctrl Pts',(108.127671920245,14.0404690398857,26.));
#92865=CARTESIAN_POINT('Ctrl Pts',(108.124576114257,14.0744781941125,26.));
#92866=CARTESIAN_POINT('Ctrl Pts',(108.122051296587,14.1080161789411,26.));
#92867=CARTESIAN_POINT('Ctrl Pts',(108.120094755478,14.141075848522,26.));
#92868=CARTESIAN_POINT('Ctrl Pts',(108.118699969367,14.1736486380529,26.));
#92869=CARTESIAN_POINT('Ctrl Pts',(108.117857140196,14.2057226050197,26.));
#92870=CARTESIAN_POINT('Ctrl Pts',(108.11755334977,14.2372805163279,26.));
#92871=CARTESIAN_POINT('Ctrl Pts',(108.117772886125,14.2682984546298,26.));
#92872=CARTESIAN_POINT('Ctrl Pts',(108.118496961781,14.2987431062216,26.));
#92873=CARTESIAN_POINT('Ctrl Pts',(108.119705321862,14.3285749073991,26.));
#92874=CARTESIAN_POINT('Ctrl Pts',(108.121378863878,14.3577546057035,26.));
#92875=CARTESIAN_POINT('Ctrl Pts',(108.123502124645,14.3862495604353,26.));
#92876=CARTESIAN_POINT('Ctrl Pts',(108.126065158394,14.4140388871472,26.));
#92877=CARTESIAN_POINT('Ctrl Pts',(108.129067047035,14.4411228648582,26.));
#92878=CARTESIAN_POINT('Ctrl Pts',(108.132512853032,14.4675164161688,26.));
#92879=CARTESIAN_POINT('Ctrl Pts',(108.136405082654,14.4932291911838,26.));
#92880=CARTESIAN_POINT('Ctrl Pts',(108.140736063189,14.5182483587362,26.));
#92881=CARTESIAN_POINT('Ctrl Pts',(108.145480953033,14.5425228839262,26.));
#92882=CARTESIAN_POINT('Ctrl Pts',(108.150587396025,14.5659407047248,26.));
#92883=CARTESIAN_POINT('Ctrl Pts',(108.155978401035,14.5883354024226,26.));
#92884=CARTESIAN_POINT('Ctrl Pts',(108.161565843363,14.6095165692449,26.));
#92885=CARTESIAN_POINT('Ctrl Pts',(108.167261205399,14.6292944653163,26.));
#92886=CARTESIAN_POINT('Ctrl Pts',(108.172986416044,14.6475048278073,26.));
#92887=CARTESIAN_POINT('Ctrl Pts',(108.178687097234,14.6640400995864,26.));
#92888=CARTESIAN_POINT('Ctrl Pts',(108.184331851892,14.6788459938496,26.));
#92889=CARTESIAN_POINT('Ctrl Pts',(108.188790420063,14.6892908937643,26.));
#92890=CARTESIAN_POINT('Ctrl Pts',(108.192099987045,14.6963371269515,26.));
#92891=CARTESIAN_POINT('Ctrl Pts',(108.194291116197,14.7006852604777,26.));
#92892=CARTESIAN_POINT('Ctrl Pts',(108.195382868896,14.702771989219,26.));
#92893=CARTESIAN_POINT('',(108.145858377777,13.8997367347037,31.));
#92894=CARTESIAN_POINT('Origin',(110.000000000001,18.0000000000028,31.));
#92895=CARTESIAN_POINT('',(108.411752154813,13.7895999261044,31.));
#92896=CARTESIAN_POINT('Origin',(110.000000000001,18.0000000000028,31.));
#92897=CARTESIAN_POINT('',(108.411752154813,13.7895999261044,26.));
#92898=CARTESIAN_POINT('Origin',(110.000000000001,18.0000000000028,26.));
#92899=CARTESIAN_POINT('',(108.411752154813,13.7895999261044,31.));
#92900=CARTESIAN_POINT('Ctrl Pts',(108.944564725307,14.3924507036097,31.));
#92901=CARTESIAN_POINT('Ctrl Pts',(108.944564725307,14.3924507036097,26.));
#92902=CARTESIAN_POINT('Ctrl Pts',(108.943861171006,14.3902031778268,31.));
#92903=CARTESIAN_POINT('Ctrl Pts',(108.943861171006,14.3902031778268,26.));
#92904=CARTESIAN_POINT('Ctrl Pts',(108.942335938597,14.3855792208381,31.));
#92905=CARTESIAN_POINT('Ctrl Pts',(108.942335938597,14.3855792208381,26.));
#92906=CARTESIAN_POINT('Ctrl Pts',(108.939693716593,14.3782565643098,31.));
#92907=CARTESIAN_POINT('Ctrl Pts',(108.939693716593,14.3782565643098,26.));
#92908=CARTESIAN_POINT('Ctrl Pts',(108.935460740827,14.3677182209614,31.));
#92909=CARTESIAN_POINT('Ctrl Pts',(108.935460740827,14.3677182209614,26.));
#92910=CARTESIAN_POINT('Ctrl Pts',(108.928982836883,14.3532574284319,31.));
#92911=CARTESIAN_POINT('Ctrl Pts',(108.928982836883,14.3532574284319,26.));
#92912=CARTESIAN_POINT('Ctrl Pts',(108.921321624393,14.3375342353073,31.));
#92913=CARTESIAN_POINT('Ctrl Pts',(108.921321624393,14.3375342353073,26.));
#92914=CARTESIAN_POINT('Ctrl Pts',(108.912493288843,14.3206092292388,31.));
#92915=CARTESIAN_POINT('Ctrl Pts',(108.912493288843,14.3206092292388,26.));
#92916=CARTESIAN_POINT('Ctrl Pts',(108.902535433517,14.3025969156976,31.));
#92917=CARTESIAN_POINT('Ctrl Pts',(108.902535433517,14.3025969156976,26.));
#92918=CARTESIAN_POINT('Ctrl Pts',(108.891509005179,14.2836686506462,31.));
#92919=CARTESIAN_POINT('Ctrl Pts',(108.891509005179,14.2836686506462,26.));
#92920=CARTESIAN_POINT('Ctrl Pts',(108.879485578779,14.2640211918396,31.));
#92921=CARTESIAN_POINT('Ctrl Pts',(108.879485578779,14.2640211918396,26.));
#92922=CARTESIAN_POINT('Ctrl Pts',(108.86653747937,14.2438514914799,31.));
#92923=CARTESIAN_POINT('Ctrl Pts',(108.86653747937,14.2438514914799,26.));
#92924=CARTESIAN_POINT('Ctrl Pts',(108.852727941796,14.2233316663176,31.));
#92925=CARTESIAN_POINT('Ctrl Pts',(108.852727941796,14.2233316663176,26.));
#92926=CARTESIAN_POINT('Ctrl Pts',(108.838099184477,14.2025779775712,31.));
#92927=CARTESIAN_POINT('Ctrl Pts',(108.838099184477,14.2025779775712,26.));
#92928=CARTESIAN_POINT('Ctrl Pts',(108.822669728866,14.1816440780331,31.));
#92929=CARTESIAN_POINT('Ctrl Pts',(108.822669728866,14.1816440780331,26.));
#92930=CARTESIAN_POINT('Ctrl Pts',(108.80644322254,14.1605444661352,31.));
#92931=CARTESIAN_POINT('Ctrl Pts',(108.80644322254,14.1605444661352,26.));
#92932=CARTESIAN_POINT('Ctrl Pts',(108.789414614043,14.1392705460246,31.));
#92933=CARTESIAN_POINT('Ctrl Pts',(108.789414614043,14.1392705460246,26.));
#92934=CARTESIAN_POINT('Ctrl Pts',(108.771576931205,14.117808186126,31.));
#92935=CARTESIAN_POINT('Ctrl Pts',(108.771576931205,14.117808186126,26.));
#92936=CARTESIAN_POINT('Ctrl Pts',(108.752929327551,14.0961578383272,31.));
#92937=CARTESIAN_POINT('Ctrl Pts',(108.752929327551,14.0961578383272,26.));
#92938=CARTESIAN_POINT('Ctrl Pts',(108.733479537902,14.0743413028801,31.));
#92939=CARTESIAN_POINT('Ctrl Pts',(108.733479537902,14.0743413028801,26.));
#92940=CARTESIAN_POINT('Ctrl Pts',(108.713239708603,14.052392594365,31.));
#92941=CARTESIAN_POINT('Ctrl Pts',(108.713239708603,14.052392594365,26.));
#92942=CARTESIAN_POINT('Ctrl Pts',(108.692224087836,14.0303529759594,31.));
#92943=CARTESIAN_POINT('Ctrl Pts',(108.692224087836,14.0303529759594,26.));
#92944=CARTESIAN_POINT('Ctrl Pts',(108.670446329005,14.008264745788,31.));
#92945=CARTESIAN_POINT('Ctrl Pts',(108.670446329005,14.008264745788,26.));
#92946=CARTESIAN_POINT('Ctrl Pts',(108.647916703691,13.9861647449546,31.));
#92947=CARTESIAN_POINT('Ctrl Pts',(108.647916703691,13.9861647449546,26.));
#92948=CARTESIAN_POINT('Ctrl Pts',(108.624641013961,13.9640809956211,31.));
#92949=CARTESIAN_POINT('Ctrl Pts',(108.624641013961,13.9640809956211,26.));
#92950=CARTESIAN_POINT('Ctrl Pts',(108.60062231089,13.9420348179765,31.));
#92951=CARTESIAN_POINT('Ctrl Pts',(108.60062231089,13.9420348179765,26.));
#92952=CARTESIAN_POINT('Ctrl Pts',(108.575862110827,13.9200415849314,31.));
#92953=CARTESIAN_POINT('Ctrl Pts',(108.575862110827,13.9200415849314,26.));
#92954=CARTESIAN_POINT('Ctrl Pts',(108.550361858556,13.8981119641586,31.));
#92955=CARTESIAN_POINT('Ctrl Pts',(108.550361858556,13.8981119641586,26.));
#92956=CARTESIAN_POINT('Ctrl Pts',(108.524124689469,13.8762529260328,31.));
#92957=CARTESIAN_POINT('Ctrl Pts',(108.524124689469,13.8762529260328,26.));
#92958=CARTESIAN_POINT('Ctrl Pts',(108.497156472931,13.8544687326315,31.));
#92959=CARTESIAN_POINT('Ctrl Pts',(108.497156472931,13.8544687326315,26.));
#92960=CARTESIAN_POINT('Ctrl Pts',(108.469463960127,13.8327615615353,31.));
#92961=CARTESIAN_POINT('Ctrl Pts',(108.469463960127,13.8327615615353,26.));
#92962=CARTESIAN_POINT('Ctrl Pts',(108.446735635703,13.8154580516872,31.));
#92963=CARTESIAN_POINT('Ctrl Pts',(108.446735635703,13.8154580516872,26.));
#92964=CARTESIAN_POINT('Ctrl Pts',(108.429368471565,13.8025154070864,31.));
#92965=CARTESIAN_POINT('Ctrl Pts',(108.429368471565,13.8025154070864,26.));
#92966=CARTESIAN_POINT('Ctrl Pts',(108.417647989244,13.7939024994221,31.));
#92967=CARTESIAN_POINT('Ctrl Pts',(108.417647989244,13.7939024994221,26.));
#92968=CARTESIAN_POINT('Ctrl Pts',(108.411752154813,13.7895999261044,31.));
#92969=CARTESIAN_POINT('Ctrl Pts',(108.411752154813,13.7895999261044,26.));
#92970=CARTESIAN_POINT('Ctrl Pts',(108.944564725307,14.3924507036097,31.));
#92971=CARTESIAN_POINT('Ctrl Pts',(108.943861171006,14.3902031778268,31.));
#92972=CARTESIAN_POINT('Ctrl Pts',(108.942335938597,14.3855792208381,31.));
#92973=CARTESIAN_POINT('Ctrl Pts',(108.939693716593,14.3782565643098,31.));
#92974=CARTESIAN_POINT('Ctrl Pts',(108.935460740827,14.3677182209614,31.));
#92975=CARTESIAN_POINT('Ctrl Pts',(108.928982836883,14.3532574284319,31.));
#92976=CARTESIAN_POINT('Ctrl Pts',(108.921321624393,14.3375342353073,31.));
#92977=CARTESIAN_POINT('Ctrl Pts',(108.912493288843,14.3206092292388,31.));
#92978=CARTESIAN_POINT('Ctrl Pts',(108.902535433517,14.3025969156976,31.));
#92979=CARTESIAN_POINT('Ctrl Pts',(108.891509005179,14.2836686506462,31.));
#92980=CARTESIAN_POINT('Ctrl Pts',(108.879485578779,14.2640211918396,31.));
#92981=CARTESIAN_POINT('Ctrl Pts',(108.86653747937,14.2438514914799,31.));
#92982=CARTESIAN_POINT('Ctrl Pts',(108.852727941796,14.2233316663176,31.));
#92983=CARTESIAN_POINT('Ctrl Pts',(108.838099184477,14.2025779775712,31.));
#92984=CARTESIAN_POINT('Ctrl Pts',(108.822669728866,14.1816440780331,31.));
#92985=CARTESIAN_POINT('Ctrl Pts',(108.80644322254,14.1605444661352,31.));
#92986=CARTESIAN_POINT('Ctrl Pts',(108.789414614043,14.1392705460246,31.));
#92987=CARTESIAN_POINT('Ctrl Pts',(108.771576931205,14.117808186126,31.));
#92988=CARTESIAN_POINT('Ctrl Pts',(108.752929327551,14.0961578383272,31.));
#92989=CARTESIAN_POINT('Ctrl Pts',(108.733479537902,14.0743413028801,31.));
#92990=CARTESIAN_POINT('Ctrl Pts',(108.713239708603,14.052392594365,31.));
#92991=CARTESIAN_POINT('Ctrl Pts',(108.692224087836,14.0303529759594,31.));
#92992=CARTESIAN_POINT('Ctrl Pts',(108.670446329005,14.008264745788,31.));
#92993=CARTESIAN_POINT('Ctrl Pts',(108.647916703691,13.9861647449546,31.));
#92994=CARTESIAN_POINT('Ctrl Pts',(108.624641013961,13.9640809956211,31.));
#92995=CARTESIAN_POINT('Ctrl Pts',(108.60062231089,13.9420348179765,31.));
#92996=CARTESIAN_POINT('Ctrl Pts',(108.575862110827,13.9200415849314,31.));
#92997=CARTESIAN_POINT('Ctrl Pts',(108.550361858556,13.8981119641586,31.));
#92998=CARTESIAN_POINT('Ctrl Pts',(108.524124689469,13.8762529260328,31.));
#92999=CARTESIAN_POINT('Ctrl Pts',(108.497156472931,13.8544687326315,31.));
#93000=CARTESIAN_POINT('Ctrl Pts',(108.469463960127,13.8327615615353,31.));
#93001=CARTESIAN_POINT('Ctrl Pts',(108.446735635703,13.8154580516872,31.));
#93002=CARTESIAN_POINT('Ctrl Pts',(108.429368471565,13.8025154070864,31.));
#93003=CARTESIAN_POINT('Ctrl Pts',(108.417647989244,13.7939024994221,31.));
#93004=CARTESIAN_POINT('Ctrl Pts',(108.411752154813,13.7895999261044,31.));
#93005=CARTESIAN_POINT('Ctrl Pts',(108.944564725307,14.3924507036097,26.));
#93006=CARTESIAN_POINT('Ctrl Pts',(108.943861171006,14.3902031778268,26.));
#93007=CARTESIAN_POINT('Ctrl Pts',(108.942335938597,14.3855792208381,26.));
#93008=CARTESIAN_POINT('Ctrl Pts',(108.939693716593,14.3782565643098,26.));
#93009=CARTESIAN_POINT('Ctrl Pts',(108.935460740827,14.3677182209614,26.));
#93010=CARTESIAN_POINT('Ctrl Pts',(108.928982836883,14.3532574284319,26.));
#93011=CARTESIAN_POINT('Ctrl Pts',(108.921321624393,14.3375342353073,26.));
#93012=CARTESIAN_POINT('Ctrl Pts',(108.912493288843,14.3206092292388,26.));
#93013=CARTESIAN_POINT('Ctrl Pts',(108.902535433517,14.3025969156976,26.));
#93014=CARTESIAN_POINT('Ctrl Pts',(108.891509005179,14.2836686506462,26.));
#93015=CARTESIAN_POINT('Ctrl Pts',(108.879485578779,14.2640211918396,26.));
#93016=CARTESIAN_POINT('Ctrl Pts',(108.86653747937,14.2438514914799,26.));
#93017=CARTESIAN_POINT('Ctrl Pts',(108.852727941796,14.2233316663176,26.));
#93018=CARTESIAN_POINT('Ctrl Pts',(108.838099184477,14.2025779775712,26.));
#93019=CARTESIAN_POINT('Ctrl Pts',(108.822669728866,14.1816440780331,26.));
#93020=CARTESIAN_POINT('Ctrl Pts',(108.80644322254,14.1605444661352,26.));
#93021=CARTESIAN_POINT('Ctrl Pts',(108.789414614043,14.1392705460246,26.));
#93022=CARTESIAN_POINT('Ctrl Pts',(108.771576931205,14.117808186126,26.));
#93023=CARTESIAN_POINT('Ctrl Pts',(108.752929327551,14.0961578383272,26.));
#93024=CARTESIAN_POINT('Ctrl Pts',(108.733479537902,14.0743413028801,26.));
#93025=CARTESIAN_POINT('Ctrl Pts',(108.713239708603,14.052392594365,26.));
#93026=CARTESIAN_POINT('Ctrl Pts',(108.692224087836,14.0303529759594,26.));
#93027=CARTESIAN_POINT('Ctrl Pts',(108.670446329005,14.008264745788,26.));
#93028=CARTESIAN_POINT('Ctrl Pts',(108.647916703691,13.9861647449546,26.));
#93029=CARTESIAN_POINT('Ctrl Pts',(108.624641013961,13.9640809956211,26.));
#93030=CARTESIAN_POINT('Ctrl Pts',(108.60062231089,13.9420348179765,26.));
#93031=CARTESIAN_POINT('Ctrl Pts',(108.575862110827,13.9200415849314,26.));
#93032=CARTESIAN_POINT('Ctrl Pts',(108.550361858556,13.8981119641586,26.));
#93033=CARTESIAN_POINT('Ctrl Pts',(108.524124689469,13.8762529260328,26.));
#93034=CARTESIAN_POINT('Ctrl Pts',(108.497156472931,13.8544687326315,26.));
#93035=CARTESIAN_POINT('Ctrl Pts',(108.469463960127,13.8327615615353,26.));
#93036=CARTESIAN_POINT('Ctrl Pts',(108.446735635703,13.8154580516872,26.));
#93037=CARTESIAN_POINT('Ctrl Pts',(108.429368471565,13.8025154070864,26.));
#93038=CARTESIAN_POINT('Ctrl Pts',(108.417647989244,13.7939024994221,26.));
#93039=CARTESIAN_POINT('Ctrl Pts',(108.411752154813,13.7895999261044,26.));
#93040=CARTESIAN_POINT('Origin',(108.52548580596,14.4402078347963,31.));
#93041=CARTESIAN_POINT('Origin',(110.,18.,31.));
#93042=CARTESIAN_POINT('Origin',(110.,18.,28.9));
#93043=CARTESIAN_POINT('',(106.625,18.,31.8));
#93044=CARTESIAN_POINT('Origin',(110.,18.,31.8));
#93045=CARTESIAN_POINT('',(106.625,18.,31.));
#93046=CARTESIAN_POINT('',(106.625,18.,28.9));
#93047=CARTESIAN_POINT('',(106.644692681757,17.6359425867508,31.));
#93048=CARTESIAN_POINT('Origin',(110.,18.,31.));
#93049=CARTESIAN_POINT('',(106.644692681757,17.6359425867508,26.));
#93050=CARTESIAN_POINT('',(106.644692681757,17.6359425867508,28.9));
#93051=CARTESIAN_POINT('',(106.760781502909,17.0523246715749,26.));
#93052=CARTESIAN_POINT('Origin',(110.,18.,26.));
#93053=CARTESIAN_POINT('',(106.760781502909,17.0523246715749,31.));
#93054=CARTESIAN_POINT('',(106.760781502909,17.0523246715749,28.9));
#93055=CARTESIAN_POINT('',(107.03941898387,16.3796342860549,31.));
#93056=CARTESIAN_POINT('Origin',(110.,18.,31.));
#93057=CARTESIAN_POINT('',(107.03941898387,16.3796342860549,26.));
#93058=CARTESIAN_POINT('',(107.03941898387,16.3796342860549,28.9));
#93059=CARTESIAN_POINT('',(107.370011976655,15.884866907955,26.));
#93060=CARTESIAN_POINT('Origin',(110.,18.,26.));
#93061=CARTESIAN_POINT('',(107.370011976655,15.884866907955,31.));
#93062=CARTESIAN_POINT('',(107.370011976655,15.884866907955,28.9));
#93063=CARTESIAN_POINT('',(107.884866907955,15.3700119766554,31.));
#93064=CARTESIAN_POINT('Origin',(110.,18.,31.));
#93065=CARTESIAN_POINT('',(107.884866907955,15.3700119766554,26.));
#93066=CARTESIAN_POINT('',(107.884866907955,15.3700119766554,28.9));
#93067=CARTESIAN_POINT('Origin',(110.,18.,26.));
#93068=CARTESIAN_POINT('',(109.635942586751,14.6446926817565,26.));
#93069=CARTESIAN_POINT('Origin',(110.,18.,26.));
#93070=CARTESIAN_POINT('',(109.635942586751,14.6446926817565,31.));
#93071=CARTESIAN_POINT('',(109.635942586751,14.6446926817565,28.9));
#93072=CARTESIAN_POINT('',(110.364057413249,14.6446926817565,31.));
#93073=CARTESIAN_POINT('Origin',(110.,18.,31.));
#93074=CARTESIAN_POINT('',(110.364057413249,14.6446926817565,26.));
#93075=CARTESIAN_POINT('',(110.364057413249,14.6446926817565,28.9));
#93076=CARTESIAN_POINT('',(110.947675328425,14.7607815029093,26.));
#93077=CARTESIAN_POINT('Origin',(110.,18.,26.));
#93078=CARTESIAN_POINT('',(110.947675328425,14.7607815029093,31.));
#93079=CARTESIAN_POINT('',(110.947675328425,14.7607815029093,28.9));
#93080=CARTESIAN_POINT('',(111.620365713945,15.0394189838697,31.));
#93081=CARTESIAN_POINT('Origin',(110.,18.,31.));
#93082=CARTESIAN_POINT('',(111.620365713945,15.0394189838697,26.));
#93083=CARTESIAN_POINT('',(111.620365713945,15.0394189838697,28.9));
#93084=CARTESIAN_POINT('',(112.115133092045,15.3700119766554,26.));
#93085=CARTESIAN_POINT('Origin',(110.,18.,26.));
#93086=CARTESIAN_POINT('',(112.115133092045,15.3700119766554,31.));
#93087=CARTESIAN_POINT('',(112.115133092045,15.3700119766554,28.9));
#93088=CARTESIAN_POINT('',(112.629988023345,15.884866907955,31.));
#93089=CARTESIAN_POINT('Origin',(110.,18.,31.));
#93090=CARTESIAN_POINT('',(112.629988023345,15.884866907955,26.));
#93091=CARTESIAN_POINT('',(112.629988023345,15.884866907955,28.9));
#93092=CARTESIAN_POINT('',(112.96058101613,16.3796342860549,26.));
#93093=CARTESIAN_POINT('Origin',(110.,18.,26.));
#93094=CARTESIAN_POINT('',(112.96058101613,16.3796342860549,31.));
#93095=CARTESIAN_POINT('',(112.96058101613,16.3796342860549,28.9));
#93096=CARTESIAN_POINT('',(113.239218497091,17.0523246715749,31.));
#93097=CARTESIAN_POINT('Origin',(110.,18.,31.));
#93098=CARTESIAN_POINT('',(113.239218497091,17.0523246715749,26.));
#93099=CARTESIAN_POINT('',(113.239218497091,17.0523246715749,28.9));
#93100=CARTESIAN_POINT('',(113.355307318243,17.6359425867508,26.));
#93101=CARTESIAN_POINT('Origin',(110.,18.,26.));
#93102=CARTESIAN_POINT('',(113.355307318243,17.6359425867508,31.));
#93103=CARTESIAN_POINT('',(113.355307318243,17.6359425867508,28.9));
#93104=CARTESIAN_POINT('',(113.355307318243,18.3640574132493,31.));
#93105=CARTESIAN_POINT('Origin',(110.,18.,31.));
#93106=CARTESIAN_POINT('',(113.355307318243,18.3640574132493,26.));
#93107=CARTESIAN_POINT('',(113.355307318243,18.3640574132493,28.9));
#93108=CARTESIAN_POINT('',(113.239218497091,18.9476753284251,26.));
#93109=CARTESIAN_POINT('Origin',(110.,18.,26.));
#93110=CARTESIAN_POINT('',(113.239218497091,18.9476753284251,31.));
#93111=CARTESIAN_POINT('',(113.239218497091,18.9476753284251,28.9));
#93112=CARTESIAN_POINT('',(112.96058101613,19.6203657139451,31.));
#93113=CARTESIAN_POINT('Origin',(110.,18.,31.));
#93114=CARTESIAN_POINT('',(112.96058101613,19.6203657139451,26.));
#93115=CARTESIAN_POINT('',(112.96058101613,19.6203657139451,28.9));
#93116=CARTESIAN_POINT('',(112.629988023345,20.115133092045,26.));
#93117=CARTESIAN_POINT('Origin',(110.,18.,26.));
#93118=CARTESIAN_POINT('',(112.629988023345,20.115133092045,31.));
#93119=CARTESIAN_POINT('',(112.629988023345,20.115133092045,28.9));
#93120=CARTESIAN_POINT('',(112.115133092045,20.6299880233446,31.));
#93121=CARTESIAN_POINT('Origin',(110.,18.,31.));
#93122=CARTESIAN_POINT('',(112.115133092045,20.6299880233446,26.));
#93123=CARTESIAN_POINT('',(112.115133092045,20.6299880233446,28.9));
#93124=CARTESIAN_POINT('',(111.620365713945,20.9605810161303,26.));
#93125=CARTESIAN_POINT('Origin',(110.,18.,26.));
#93126=CARTESIAN_POINT('',(111.620365713945,20.9605810161303,31.));
#93127=CARTESIAN_POINT('',(111.620365713945,20.9605810161303,28.9));
#93128=CARTESIAN_POINT('',(110.947675328425,21.2392184970907,31.));
#93129=CARTESIAN_POINT('Origin',(110.,18.,31.));
#93130=CARTESIAN_POINT('',(110.947675328425,21.2392184970907,26.));
#93131=CARTESIAN_POINT('',(110.947675328425,21.2392184970907,28.9));
#93132=CARTESIAN_POINT('',(110.364057413249,21.3553073182435,26.));
#93133=CARTESIAN_POINT('Origin',(110.,18.,26.));
#93134=CARTESIAN_POINT('',(110.364057413249,21.3553073182435,31.));
#93135=CARTESIAN_POINT('',(110.364057413249,21.3553073182435,28.9));
#93136=CARTESIAN_POINT('',(109.635942586751,21.3553073182435,31.));
#93137=CARTESIAN_POINT('Origin',(110.,18.,31.));
#93138=CARTESIAN_POINT('',(109.635942586751,21.3553073182435,26.));
#93139=CARTESIAN_POINT('',(109.635942586751,21.3553073182435,28.9));
#93140=CARTESIAN_POINT('',(109.052324671575,21.2392184970907,26.));
#93141=CARTESIAN_POINT('Origin',(110.,18.,26.));
#93142=CARTESIAN_POINT('',(109.052324671575,21.2392184970907,31.));
#93143=CARTESIAN_POINT('',(109.052324671575,21.2392184970907,28.9));
#93144=CARTESIAN_POINT('',(108.379634286055,20.9605810161303,31.));
#93145=CARTESIAN_POINT('Origin',(110.,18.,31.));
#93146=CARTESIAN_POINT('',(108.379634286055,20.9605810161303,26.));
#93147=CARTESIAN_POINT('',(108.379634286055,20.9605810161303,28.9));
#93148=CARTESIAN_POINT('',(107.884866907955,20.6299880233446,26.));
#93149=CARTESIAN_POINT('Origin',(110.,18.,26.));
#93150=CARTESIAN_POINT('',(107.884866907955,20.6299880233446,31.));
#93151=CARTESIAN_POINT('',(107.884866907955,20.6299880233446,28.9));
#93152=CARTESIAN_POINT('',(107.370011976655,20.115133092045,31.));
#93153=CARTESIAN_POINT('Origin',(110.,18.,31.));
#93154=CARTESIAN_POINT('',(107.370011976655,20.115133092045,26.));
#93155=CARTESIAN_POINT('',(107.370011976655,20.115133092045,28.9));
#93156=CARTESIAN_POINT('',(107.03941898387,19.6203657139451,26.));
#93157=CARTESIAN_POINT('Origin',(110.,18.,26.));
#93158=CARTESIAN_POINT('',(107.03941898387,19.6203657139451,31.));
#93159=CARTESIAN_POINT('',(107.03941898387,19.6203657139451,28.9));
#93160=CARTESIAN_POINT('',(106.760781502909,18.9476753284252,31.));
#93161=CARTESIAN_POINT('Origin',(110.,18.,31.));
#93162=CARTESIAN_POINT('',(106.760781502909,18.9476753284252,26.));
#93163=CARTESIAN_POINT('',(106.760781502909,18.9476753284252,28.9));
#93164=CARTESIAN_POINT('',(106.644692681757,18.3640574132493,26.));
#93165=CARTESIAN_POINT('Origin',(110.,18.,26.));
#93166=CARTESIAN_POINT('',(106.644692681757,18.3640574132493,31.));
#93167=CARTESIAN_POINT('',(106.644692681757,18.3640574132493,28.9));
#93168=CARTESIAN_POINT('Origin',(110.,18.,31.));
#93169=CARTESIAN_POINT('Origin',(107.978872823157,15.4869003332485,31.));
#93170=CARTESIAN_POINT('',(107.644355604652,15.0709566360981,31.));
#93171=CARTESIAN_POINT('',(107.644355604652,15.0709566360981,31.));
#93172=CARTESIAN_POINT('',(107.644355604652,15.0709566360981,26.));
#93173=CARTESIAN_POINT('',(107.644355604652,15.0709566360981,31.));
#93174=CARTESIAN_POINT('',(107.644355604652,15.0709566360981,26.));
#93175=CARTESIAN_POINT('Origin',(107.070956636098,15.6443556046521,31.));
#93176=CARTESIAN_POINT('',(107.070956636098,15.6443556046521,26.));
#93177=CARTESIAN_POINT('',(107.486900333248,15.978872823157,26.));
#93178=CARTESIAN_POINT('',(107.070956636098,15.6443556046521,31.));
#93179=CARTESIAN_POINT('',(107.070956636098,15.6443556046521,31.));
#93180=CARTESIAN_POINT('',(107.486900333248,15.978872823157,31.));
#93181=CARTESIAN_POINT('Ctrl Pts',(106.717893684886,14.9213999713683,31.));
#93182=CARTESIAN_POINT('Ctrl Pts',(106.717893684886,14.9213999713683,26.));
#93183=CARTESIAN_POINT('Ctrl Pts',(106.719612506117,14.9284935356891,31.));
#93184=CARTESIAN_POINT('Ctrl Pts',(106.719612506117,14.9284935356891,26.));
#93185=CARTESIAN_POINT('Ctrl Pts',(106.723084560754,14.9426178665506,31.));
#93186=CARTESIAN_POINT('Ctrl Pts',(106.723084560754,14.9426178665506,26.));
#93187=CARTESIAN_POINT('Ctrl Pts',(106.728395879147,14.9636159697624,31.));
#93188=CARTESIAN_POINT('Ctrl Pts',(106.728395879147,14.9636159697624,26.));
#93189=CARTESIAN_POINT('Ctrl Pts',(106.735684484505,14.9912359700753,31.));
#93190=CARTESIAN_POINT('Ctrl Pts',(106.735684484505,14.9912359700753,26.));
#93191=CARTESIAN_POINT('Ctrl Pts',(106.745141829775,15.0251274905646,31.));
#93192=CARTESIAN_POINT('Ctrl Pts',(106.745141829775,15.0251274905646,26.));
#93193=CARTESIAN_POINT('Ctrl Pts',(106.754947510596,15.0583793236798,31.));
#93194=CARTESIAN_POINT('Ctrl Pts',(106.754947510596,15.0583793236798,26.));
#93195=CARTESIAN_POINT('Ctrl Pts',(106.765102098678,15.0909843988495,31.));
#93196=CARTESIAN_POINT('Ctrl Pts',(106.765102098678,15.0909843988495,26.));
#93197=CARTESIAN_POINT('Ctrl Pts',(106.775603902459,15.1229356624862,31.));
#93198=CARTESIAN_POINT('Ctrl Pts',(106.775603902459,15.1229356624862,26.));
#93199=CARTESIAN_POINT('Ctrl Pts',(106.786447682002,15.1542275504307,31.));
#93200=CARTESIAN_POINT('Ctrl Pts',(106.786447682002,15.1542275504307,26.));
#93201=CARTESIAN_POINT('Ctrl Pts',(106.79762413456,15.1848546455316,31.));
#93202=CARTESIAN_POINT('Ctrl Pts',(106.79762413456,15.1848546455316,26.));
#93203=CARTESIAN_POINT('Ctrl Pts',(106.809119637709,15.2148096638986,31.));
#93204=CARTESIAN_POINT('Ctrl Pts',(106.809119637709,15.2148096638986,26.));
#93205=CARTESIAN_POINT('Ctrl Pts',(106.82091566177,15.244081627808,31.));
#93206=CARTESIAN_POINT('Ctrl Pts',(106.82091566177,15.244081627808,26.));
#93207=CARTESIAN_POINT('Ctrl Pts',(106.832988538009,15.2726544532201,31.));
#93208=CARTESIAN_POINT('Ctrl Pts',(106.832988538009,15.2726544532201,26.));
#93209=CARTESIAN_POINT('Ctrl Pts',(106.845308160455,15.3005045519429,31.));
#93210=CARTESIAN_POINT('Ctrl Pts',(106.845308160455,15.3005045519429,26.));
#93211=CARTESIAN_POINT('Ctrl Pts',(106.85784067567,15.3276031230855,31.));
#93212=CARTESIAN_POINT('Ctrl Pts',(106.85784067567,15.3276031230855,26.));
#93213=CARTESIAN_POINT('Ctrl Pts',(106.870553413989,15.3539212123107,31.));
#93214=CARTESIAN_POINT('Ctrl Pts',(106.870553413989,15.3539212123107,26.));
#93215=CARTESIAN_POINT('Ctrl Pts',(106.883419598235,15.379434581049,31.));
#93216=CARTESIAN_POINT('Ctrl Pts',(106.883419598235,15.379434581049,26.));
#93217=CARTESIAN_POINT('Ctrl Pts',(106.896422047586,15.4041277406684,31.));
#93218=CARTESIAN_POINT('Ctrl Pts',(106.896422047586,15.4041277406684,26.));
#93219=CARTESIAN_POINT('Ctrl Pts',(106.909560020613,15.4280013002857,31.));
#93220=CARTESIAN_POINT('Ctrl Pts',(106.909560020613,15.4280013002857,26.));
#93221=CARTESIAN_POINT('Ctrl Pts',(106.922843905055,15.4510671092656,31.));
#93222=CARTESIAN_POINT('Ctrl Pts',(106.922843905055,15.4510671092656,26.));
#93223=CARTESIAN_POINT('Ctrl Pts',(106.936279709336,15.4733331240349,31.));
#93224=CARTESIAN_POINT('Ctrl Pts',(106.936279709336,15.4733331240349,26.));
#93225=CARTESIAN_POINT('Ctrl Pts',(106.949855434522,15.4947904263603,31.));
#93226=CARTESIAN_POINT('Ctrl Pts',(106.949855434522,15.4947904263603,26.));
#93227=CARTESIAN_POINT('Ctrl Pts',(106.963528599752,15.5154013726131,31.));
#93228=CARTESIAN_POINT('Ctrl Pts',(106.963528599752,15.5154013726131,26.));
#93229=CARTESIAN_POINT('Ctrl Pts',(106.977207949958,15.5350824668136,31.));
#93230=CARTESIAN_POINT('Ctrl Pts',(106.977207949958,15.5350824668136,26.));
#93231=CARTESIAN_POINT('Ctrl Pts',(106.990758668928,15.5537094213523,31.));
#93232=CARTESIAN_POINT('Ctrl Pts',(106.990758668928,15.5537094213523,26.));
#93233=CARTESIAN_POINT('Ctrl Pts',(107.004026474155,15.5711400462457,31.));
#93234=CARTESIAN_POINT('Ctrl Pts',(107.004026474155,15.5711400462457,26.));
#93235=CARTESIAN_POINT('Ctrl Pts',(107.016856975724,15.5872329189297,31.));
#93236=CARTESIAN_POINT('Ctrl Pts',(107.016856975724,15.5872329189297,26.));
#93237=CARTESIAN_POINT('Ctrl Pts',(107.029115184681,15.6018661568543,31.));
#93238=CARTESIAN_POINT('Ctrl Pts',(107.029115184681,15.6018661568543,26.));
#93239=CARTESIAN_POINT('Ctrl Pts',(107.040709701913,15.6149611997708,31.));
#93240=CARTESIAN_POINT('Ctrl Pts',(107.040709701913,15.6149611997708,26.));
#93241=CARTESIAN_POINT('Ctrl Pts',(107.051590745644,15.6264799083536,31.));
#93242=CARTESIAN_POINT('Ctrl Pts',(107.051590745644,15.6264799083536,26.));
#93243=CARTESIAN_POINT('Ctrl Pts',(107.059707015671,15.6344235174329,31.));
#93244=CARTESIAN_POINT('Ctrl Pts',(107.059707015671,15.6344235174329,26.));
#93245=CARTESIAN_POINT('Ctrl Pts',(107.065461133568,15.6396668716037,31.));
#93246=CARTESIAN_POINT('Ctrl Pts',(107.065461133568,15.6396668716037,26.));
#93247=CARTESIAN_POINT('Ctrl Pts',(107.069149431608,15.6428455143482,31.));
#93248=CARTESIAN_POINT('Ctrl Pts',(107.069149431608,15.6428455143482,26.));
#93249=CARTESIAN_POINT('Ctrl Pts',(107.070956636098,15.6443556046521,31.));
#93250=CARTESIAN_POINT('Ctrl Pts',(107.070956636098,15.6443556046521,26.));
#93251=CARTESIAN_POINT('',(106.717893684886,14.9213999713683,31.));
#93252=CARTESIAN_POINT('Ctrl Pts',(107.070956636098,15.6443556046521,31.));
#93253=CARTESIAN_POINT('Ctrl Pts',(107.069149431608,15.6428455143482,31.));
#93254=CARTESIAN_POINT('Ctrl Pts',(107.065461133568,15.6396668716037,31.));
#93255=CARTESIAN_POINT('Ctrl Pts',(107.059707015671,15.6344235174329,31.));
#93256=CARTESIAN_POINT('Ctrl Pts',(107.051590745644,15.6264799083536,31.));
#93257=CARTESIAN_POINT('Ctrl Pts',(107.040709701913,15.6149611997708,31.));
#93258=CARTESIAN_POINT('Ctrl Pts',(107.029115184681,15.6018661568543,31.));
#93259=CARTESIAN_POINT('Ctrl Pts',(107.016856975724,15.5872329189297,31.));
#93260=CARTESIAN_POINT('Ctrl Pts',(107.004026474155,15.5711400462457,31.));
#93261=CARTESIAN_POINT('Ctrl Pts',(106.990758668928,15.5537094213523,31.));
#93262=CARTESIAN_POINT('Ctrl Pts',(106.977207949958,15.5350824668136,31.));
#93263=CARTESIAN_POINT('Ctrl Pts',(106.963528599752,15.5154013726131,31.));
#93264=CARTESIAN_POINT('Ctrl Pts',(106.949855434522,15.4947904263603,31.));
#93265=CARTESIAN_POINT('Ctrl Pts',(106.936279709336,15.4733331240349,31.));
#93266=CARTESIAN_POINT('Ctrl Pts',(106.922843905055,15.4510671092656,31.));
#93267=CARTESIAN_POINT('Ctrl Pts',(106.909560020613,15.4280013002857,31.));
#93268=CARTESIAN_POINT('Ctrl Pts',(106.896422047586,15.4041277406684,31.));
#93269=CARTESIAN_POINT('Ctrl Pts',(106.883419598235,15.379434581049,31.));
#93270=CARTESIAN_POINT('Ctrl Pts',(106.870553413989,15.3539212123107,31.));
#93271=CARTESIAN_POINT('Ctrl Pts',(106.85784067567,15.3276031230855,31.));
#93272=CARTESIAN_POINT('Ctrl Pts',(106.845308160455,15.3005045519429,31.));
#93273=CARTESIAN_POINT('Ctrl Pts',(106.832988538009,15.2726544532201,31.));
#93274=CARTESIAN_POINT('Ctrl Pts',(106.82091566177,15.244081627808,31.));
#93275=CARTESIAN_POINT('Ctrl Pts',(106.809119637709,15.2148096638986,31.));
#93276=CARTESIAN_POINT('Ctrl Pts',(106.79762413456,15.1848546455316,31.));
#93277=CARTESIAN_POINT('Ctrl Pts',(106.786447682002,15.1542275504307,31.));
#93278=CARTESIAN_POINT('Ctrl Pts',(106.775603902459,15.1229356624862,31.));
#93279=CARTESIAN_POINT('Ctrl Pts',(106.765102098678,15.0909843988495,31.));
#93280=CARTESIAN_POINT('Ctrl Pts',(106.754947510596,15.0583793236798,31.));
#93281=CARTESIAN_POINT('Ctrl Pts',(106.745141829775,15.0251274905646,31.));
#93282=CARTESIAN_POINT('Ctrl Pts',(106.735684484505,14.9912359700753,31.));
#93283=CARTESIAN_POINT('Ctrl Pts',(106.728395879147,14.9636159697624,31.));
#93284=CARTESIAN_POINT('Ctrl Pts',(106.723084560754,14.9426178665506,31.));
#93285=CARTESIAN_POINT('Ctrl Pts',(106.719612506117,14.9284935356891,31.));
#93286=CARTESIAN_POINT('Ctrl Pts',(106.717893684886,14.9213999713683,31.));
#93287=CARTESIAN_POINT('',(106.717893684886,14.9213999713683,26.));
#93288=CARTESIAN_POINT('Ctrl Pts',(106.717893684886,14.9213999713683,26.));
#93289=CARTESIAN_POINT('Ctrl Pts',(106.719612506117,14.9284935356891,26.));
#93290=CARTESIAN_POINT('Ctrl Pts',(106.723084560754,14.9426178665506,26.));
#93291=CARTESIAN_POINT('Ctrl Pts',(106.728395879147,14.9636159697624,26.));
#93292=CARTESIAN_POINT('Ctrl Pts',(106.735684484505,14.9912359700753,26.));
#93293=CARTESIAN_POINT('Ctrl Pts',(106.745141829775,15.0251274905646,26.));
#93294=CARTESIAN_POINT('Ctrl Pts',(106.754947510596,15.0583793236798,26.));
#93295=CARTESIAN_POINT('Ctrl Pts',(106.765102098678,15.0909843988495,26.));
#93296=CARTESIAN_POINT('Ctrl Pts',(106.775603902459,15.1229356624862,26.));
#93297=CARTESIAN_POINT('Ctrl Pts',(106.786447682002,15.1542275504307,26.));
#93298=CARTESIAN_POINT('Ctrl Pts',(106.79762413456,15.1848546455316,26.));
#93299=CARTESIAN_POINT('Ctrl Pts',(106.809119637709,15.2148096638986,26.));
#93300=CARTESIAN_POINT('Ctrl Pts',(106.82091566177,15.244081627808,26.));
#93301=CARTESIAN_POINT('Ctrl Pts',(106.832988538009,15.2726544532201,26.));
#93302=CARTESIAN_POINT('Ctrl Pts',(106.845308160455,15.3005045519429,26.));
#93303=CARTESIAN_POINT('Ctrl Pts',(106.85784067567,15.3276031230855,26.));
#93304=CARTESIAN_POINT('Ctrl Pts',(106.870553413989,15.3539212123107,26.));
#93305=CARTESIAN_POINT('Ctrl Pts',(106.883419598235,15.379434581049,26.));
#93306=CARTESIAN_POINT('Ctrl Pts',(106.896422047586,15.4041277406684,26.));
#93307=CARTESIAN_POINT('Ctrl Pts',(106.909560020613,15.4280013002857,26.));
#93308=CARTESIAN_POINT('Ctrl Pts',(106.922843905055,15.4510671092656,26.));
#93309=CARTESIAN_POINT('Ctrl Pts',(106.936279709336,15.4733331240349,26.));
#93310=CARTESIAN_POINT('Ctrl Pts',(106.949855434522,15.4947904263603,26.));
#93311=CARTESIAN_POINT('Ctrl Pts',(106.963528599752,15.5154013726131,26.));
#93312=CARTESIAN_POINT('Ctrl Pts',(106.977207949958,15.5350824668136,26.));
#93313=CARTESIAN_POINT('Ctrl Pts',(106.990758668928,15.5537094213523,26.));
#93314=CARTESIAN_POINT('Ctrl Pts',(107.004026474155,15.5711400462457,26.));
#93315=CARTESIAN_POINT('Ctrl Pts',(107.016856975724,15.5872329189297,26.));
#93316=CARTESIAN_POINT('Ctrl Pts',(107.029115184681,15.6018661568543,26.));
#93317=CARTESIAN_POINT('Ctrl Pts',(107.040709701913,15.6149611997708,26.));
#93318=CARTESIAN_POINT('Ctrl Pts',(107.051590745644,15.6264799083536,26.));
#93319=CARTESIAN_POINT('Ctrl Pts',(107.059707015671,15.6344235174329,26.));
#93320=CARTESIAN_POINT('Ctrl Pts',(107.065461133568,15.6396668716037,26.));
#93321=CARTESIAN_POINT('Ctrl Pts',(107.069149431608,15.6428455143482,26.));
#93322=CARTESIAN_POINT('Ctrl Pts',(107.070956636098,15.6443556046521,26.));
#93323=CARTESIAN_POINT('',(106.717893684886,14.9213999713683,31.));
#93324=CARTESIAN_POINT('Origin',(110.000000000002,18.0000000000022,31.));
#93325=CARTESIAN_POINT('',(106.921399971368,14.7178936848864,31.));
#93326=CARTESIAN_POINT('Origin',(110.000000000002,18.0000000000022,31.));
#93327=CARTESIAN_POINT('',(106.921399971368,14.7178936848864,26.));
#93328=CARTESIAN_POINT('Origin',(110.000000000002,18.0000000000022,26.));
#93329=CARTESIAN_POINT('',(106.921399971368,14.7178936848864,31.));
#93330=CARTESIAN_POINT('Ctrl Pts',(107.644355604652,15.0709566360981,31.));
#93331=CARTESIAN_POINT('Ctrl Pts',(107.644355604652,15.0709566360981,26.));
#93332=CARTESIAN_POINT('Ctrl Pts',(107.642845514352,15.0691494316033,31.));
#93333=CARTESIAN_POINT('Ctrl Pts',(107.642845514352,15.0691494316033,26.));
#93334=CARTESIAN_POINT('Ctrl Pts',(107.639666871615,15.0654611335559,31.));
#93335=CARTESIAN_POINT('Ctrl Pts',(107.639666871615,15.0654611335559,26.));
#93336=CARTESIAN_POINT('Ctrl Pts',(107.634423517451,15.0597070156512,31.));
#93337=CARTESIAN_POINT('Ctrl Pts',(107.634423517451,15.0597070156512,26.));
#93338=CARTESIAN_POINT('Ctrl Pts',(107.626479908375,15.0515907456204,31.));
#93339=CARTESIAN_POINT('Ctrl Pts',(107.626479908375,15.0515907456204,26.));
#93340=CARTESIAN_POINT('Ctrl Pts',(107.614961199788,15.0407097018941,31.));
#93341=CARTESIAN_POINT('Ctrl Pts',(107.614961199788,15.0407097018941,26.));
#93342=CARTESIAN_POINT('Ctrl Pts',(107.601866156862,15.0291151846723,31.));
#93343=CARTESIAN_POINT('Ctrl Pts',(107.601866156862,15.0291151846723,26.));
#93344=CARTESIAN_POINT('Ctrl Pts',(107.587232918926,15.0168569757285,31.));
#93345=CARTESIAN_POINT('Ctrl Pts',(107.587232918926,15.0168569757285,26.));
#93346=CARTESIAN_POINT('Ctrl Pts',(107.571140046232,15.0040264741695,31.));
#93347=CARTESIAN_POINT('Ctrl Pts',(107.571140046232,15.0040264741695,26.));
#93348=CARTESIAN_POINT('Ctrl Pts',(107.553709421335,14.9907586689459,31.));
#93349=CARTESIAN_POINT('Ctrl Pts',(107.553709421335,14.9907586689459,26.));
#93350=CARTESIAN_POINT('Ctrl Pts',(107.5350824668,14.9772079499723,31.));
#93351=CARTESIAN_POINT('Ctrl Pts',(107.5350824668,14.9772079499723,26.));
#93352=CARTESIAN_POINT('Ctrl Pts',(107.515401372608,14.9635285997574,31.));
#93353=CARTESIAN_POINT('Ctrl Pts',(107.515401372608,14.9635285997574,26.));
#93354=CARTESIAN_POINT('Ctrl Pts',(107.494790426365,14.9498554345175,31.));
#93355=CARTESIAN_POINT('Ctrl Pts',(107.494790426365,14.9498554345175,26.));
#93356=CARTESIAN_POINT('Ctrl Pts',(107.473333124048,14.9362797093226,31.));
#93357=CARTESIAN_POINT('Ctrl Pts',(107.473333124048,14.9362797093226,26.));
#93358=CARTESIAN_POINT('Ctrl Pts',(107.451067109284,14.9228439050363,31.));
#93359=CARTESIAN_POINT('Ctrl Pts',(107.451067109284,14.9228439050363,26.));
#93360=CARTESIAN_POINT('Ctrl Pts',(107.428001300302,14.9095600205959,31.));
#93361=CARTESIAN_POINT('Ctrl Pts',(107.428001300302,14.9095600205959,26.));
#93362=CARTESIAN_POINT('Ctrl Pts',(107.404127740676,14.8964220475778,31.));
#93363=CARTESIAN_POINT('Ctrl Pts',(107.404127740676,14.8964220475778,26.));
#93364=CARTESIAN_POINT('Ctrl Pts',(107.379434581043,14.8834195982418,31.));
#93365=CARTESIAN_POINT('Ctrl Pts',(107.379434581043,14.8834195982418,26.));
#93366=CARTESIAN_POINT('Ctrl Pts',(107.353921212289,14.8705534140105,31.));
#93367=CARTESIAN_POINT('Ctrl Pts',(107.353921212289,14.8705534140105,26.));
#93368=CARTESIAN_POINT('Ctrl Pts',(107.327603123054,14.8578406757021,31.));
#93369=CARTESIAN_POINT('Ctrl Pts',(107.327603123054,14.8578406757021,26.));
#93370=CARTESIAN_POINT('Ctrl Pts',(107.300504551911,14.8453081604869,31.));
#93371=CARTESIAN_POINT('Ctrl Pts',(107.300504551911,14.8453081604869,26.));
#93372=CARTESIAN_POINT('Ctrl Pts',(107.272654453203,14.8329885380258,31.));
#93373=CARTESIAN_POINT('Ctrl Pts',(107.272654453203,14.8329885380258,26.));
#93374=CARTESIAN_POINT('Ctrl Pts',(107.244081627818,14.8209156617599,31.));
#93375=CARTESIAN_POINT('Ctrl Pts',(107.244081627818,14.8209156617599,26.));
#93376=CARTESIAN_POINT('Ctrl Pts',(107.214809663941,14.8091196376662,31.));
#93377=CARTESIAN_POINT('Ctrl Pts',(107.214809663941,14.8091196376662,26.));
#93378=CARTESIAN_POINT('Ctrl Pts',(107.1848546456,14.7976241344926,31.));
#93379=CARTESIAN_POINT('Ctrl Pts',(107.1848546456,14.7976241344926,26.));
#93380=CARTESIAN_POINT('Ctrl Pts',(107.154227550504,14.7864476819287,31.));
#93381=CARTESIAN_POINT('Ctrl Pts',(107.154227550504,14.7864476819287,26.));
#93382=CARTESIAN_POINT('Ctrl Pts',(107.122935662534,14.7756039024108,31.));
#93383=CARTESIAN_POINT('Ctrl Pts',(107.122935662534,14.7756039024108,26.));
#93384=CARTESIAN_POINT('Ctrl Pts',(107.090984398839,14.7651020986883,31.));
#93385=CARTESIAN_POINT('Ctrl Pts',(107.090984398839,14.7651020986883,26.));
#93386=CARTESIAN_POINT('Ctrl Pts',(107.05837932359,14.7549475106854,31.));
#93387=CARTESIAN_POINT('Ctrl Pts',(107.05837932359,14.7549475106854,26.));
#93388=CARTESIAN_POINT('Ctrl Pts',(107.0251274904,14.7451418299393,31.));
#93389=CARTESIAN_POINT('Ctrl Pts',(107.0251274904,14.7451418299393,26.));
#93390=CARTESIAN_POINT('Ctrl Pts',(106.991235969875,14.7356844847053,31.));
#93391=CARTESIAN_POINT('Ctrl Pts',(106.991235969875,14.7356844847053,26.));
#93392=CARTESIAN_POINT('Ctrl Pts',(106.963615969591,14.7283958793185,31.));
#93393=CARTESIAN_POINT('Ctrl Pts',(106.963615969591,14.7283958793185,26.));
#93394=CARTESIAN_POINT('Ctrl Pts',(106.942617866446,14.7230845608581,31.));
#93395=CARTESIAN_POINT('Ctrl Pts',(106.942617866446,14.7230845608581,26.));
#93396=CARTESIAN_POINT('Ctrl Pts',(106.928493535651,14.7196125061553,31.));
#93397=CARTESIAN_POINT('Ctrl Pts',(106.928493535651,14.7196125061553,26.));
#93398=CARTESIAN_POINT('Ctrl Pts',(106.921399971368,14.7178936848864,31.));
#93399=CARTESIAN_POINT('Ctrl Pts',(106.921399971368,14.7178936848864,26.));
#93400=CARTESIAN_POINT('Ctrl Pts',(107.644355604652,15.0709566360981,31.));
#93401=CARTESIAN_POINT('Ctrl Pts',(107.642845514352,15.0691494316033,31.));
#93402=CARTESIAN_POINT('Ctrl Pts',(107.639666871615,15.0654611335559,31.));
#93403=CARTESIAN_POINT('Ctrl Pts',(107.634423517451,15.0597070156512,31.));
#93404=CARTESIAN_POINT('Ctrl Pts',(107.626479908375,15.0515907456204,31.));
#93405=CARTESIAN_POINT('Ctrl Pts',(107.614961199788,15.0407097018941,31.));
#93406=CARTESIAN_POINT('Ctrl Pts',(107.601866156862,15.0291151846723,31.));
#93407=CARTESIAN_POINT('Ctrl Pts',(107.587232918926,15.0168569757285,31.));
#93408=CARTESIAN_POINT('Ctrl Pts',(107.571140046232,15.0040264741695,31.));
#93409=CARTESIAN_POINT('Ctrl Pts',(107.553709421335,14.9907586689459,31.));
#93410=CARTESIAN_POINT('Ctrl Pts',(107.5350824668,14.9772079499723,31.));
#93411=CARTESIAN_POINT('Ctrl Pts',(107.515401372608,14.9635285997574,31.));
#93412=CARTESIAN_POINT('Ctrl Pts',(107.494790426365,14.9498554345175,31.));
#93413=CARTESIAN_POINT('Ctrl Pts',(107.473333124048,14.9362797093226,31.));
#93414=CARTESIAN_POINT('Ctrl Pts',(107.451067109284,14.9228439050363,31.));
#93415=CARTESIAN_POINT('Ctrl Pts',(107.428001300302,14.9095600205959,31.));
#93416=CARTESIAN_POINT('Ctrl Pts',(107.404127740676,14.8964220475778,31.));
#93417=CARTESIAN_POINT('Ctrl Pts',(107.379434581043,14.8834195982418,31.));
#93418=CARTESIAN_POINT('Ctrl Pts',(107.353921212289,14.8705534140105,31.));
#93419=CARTESIAN_POINT('Ctrl Pts',(107.327603123054,14.8578406757021,31.));
#93420=CARTESIAN_POINT('Ctrl Pts',(107.300504551911,14.8453081604869,31.));
#93421=CARTESIAN_POINT('Ctrl Pts',(107.272654453203,14.8329885380258,31.));
#93422=CARTESIAN_POINT('Ctrl Pts',(107.244081627818,14.8209156617599,31.));
#93423=CARTESIAN_POINT('Ctrl Pts',(107.214809663941,14.8091196376662,31.));
#93424=CARTESIAN_POINT('Ctrl Pts',(107.1848546456,14.7976241344926,31.));
#93425=CARTESIAN_POINT('Ctrl Pts',(107.154227550504,14.7864476819287,31.));
#93426=CARTESIAN_POINT('Ctrl Pts',(107.122935662534,14.7756039024108,31.));
#93427=CARTESIAN_POINT('Ctrl Pts',(107.090984398839,14.7651020986883,31.));
#93428=CARTESIAN_POINT('Ctrl Pts',(107.05837932359,14.7549475106854,31.));
#93429=CARTESIAN_POINT('Ctrl Pts',(107.0251274904,14.7451418299393,31.));
#93430=CARTESIAN_POINT('Ctrl Pts',(106.991235969875,14.7356844847053,31.));
#93431=CARTESIAN_POINT('Ctrl Pts',(106.963615969591,14.7283958793185,31.));
#93432=CARTESIAN_POINT('Ctrl Pts',(106.942617866446,14.7230845608581,31.));
#93433=CARTESIAN_POINT('Ctrl Pts',(106.928493535651,14.7196125061553,31.));
#93434=CARTESIAN_POINT('Ctrl Pts',(106.921399971368,14.7178936848864,31.));
#93435=CARTESIAN_POINT('Ctrl Pts',(107.644355604652,15.0709566360981,26.));
#93436=CARTESIAN_POINT('Ctrl Pts',(107.642845514352,15.0691494316033,26.));
#93437=CARTESIAN_POINT('Ctrl Pts',(107.639666871615,15.0654611335559,26.));
#93438=CARTESIAN_POINT('Ctrl Pts',(107.634423517451,15.0597070156512,26.));
#93439=CARTESIAN_POINT('Ctrl Pts',(107.626479908375,15.0515907456204,26.));
#93440=CARTESIAN_POINT('Ctrl Pts',(107.614961199788,15.0407097018941,26.));
#93441=CARTESIAN_POINT('Ctrl Pts',(107.601866156862,15.0291151846723,26.));
#93442=CARTESIAN_POINT('Ctrl Pts',(107.587232918926,15.0168569757285,26.));
#93443=CARTESIAN_POINT('Ctrl Pts',(107.571140046232,15.0040264741695,26.));
#93444=CARTESIAN_POINT('Ctrl Pts',(107.553709421335,14.9907586689459,26.));
#93445=CARTESIAN_POINT('Ctrl Pts',(107.5350824668,14.9772079499723,26.));
#93446=CARTESIAN_POINT('Ctrl Pts',(107.515401372608,14.9635285997574,26.));
#93447=CARTESIAN_POINT('Ctrl Pts',(107.494790426365,14.9498554345175,26.));
#93448=CARTESIAN_POINT('Ctrl Pts',(107.473333124048,14.9362797093226,26.));
#93449=CARTESIAN_POINT('Ctrl Pts',(107.451067109284,14.9228439050363,26.));
#93450=CARTESIAN_POINT('Ctrl Pts',(107.428001300302,14.9095600205959,26.));
#93451=CARTESIAN_POINT('Ctrl Pts',(107.404127740676,14.8964220475778,26.));
#93452=CARTESIAN_POINT('Ctrl Pts',(107.379434581043,14.8834195982418,26.));
#93453=CARTESIAN_POINT('Ctrl Pts',(107.353921212289,14.8705534140105,26.));
#93454=CARTESIAN_POINT('Ctrl Pts',(107.327603123054,14.8578406757021,26.));
#93455=CARTESIAN_POINT('Ctrl Pts',(107.300504551911,14.8453081604869,26.));
#93456=CARTESIAN_POINT('Ctrl Pts',(107.272654453203,14.8329885380258,26.));
#93457=CARTESIAN_POINT('Ctrl Pts',(107.244081627818,14.8209156617599,26.));
#93458=CARTESIAN_POINT('Ctrl Pts',(107.214809663941,14.8091196376662,26.));
#93459=CARTESIAN_POINT('Ctrl Pts',(107.1848546456,14.7976241344926,26.));
#93460=CARTESIAN_POINT('Ctrl Pts',(107.154227550504,14.7864476819287,26.));
#93461=CARTESIAN_POINT('Ctrl Pts',(107.122935662534,14.7756039024108,26.));
#93462=CARTESIAN_POINT('Ctrl Pts',(107.090984398839,14.7651020986883,26.));
#93463=CARTESIAN_POINT('Ctrl Pts',(107.05837932359,14.7549475106854,26.));
#93464=CARTESIAN_POINT('Ctrl Pts',(107.0251274904,14.7451418299393,26.));
#93465=CARTESIAN_POINT('Ctrl Pts',(106.991235969875,14.7356844847053,26.));
#93466=CARTESIAN_POINT('Ctrl Pts',(106.963615969591,14.7283958793185,26.));
#93467=CARTESIAN_POINT('Ctrl Pts',(106.942617866446,14.7230845608581,26.));
#93468=CARTESIAN_POINT('Ctrl Pts',(106.928493535651,14.7196125061553,26.));
#93469=CARTESIAN_POINT('Ctrl Pts',(106.921399971368,14.7178936848864,26.));
#93470=CARTESIAN_POINT('Origin',(107.275453031443,15.2754530314203,31.));
#93471=CARTESIAN_POINT('Origin',(107.171000362364,16.451650540008,31.));
#93472=CARTESIAN_POINT('',(106.702771989219,16.1953828688963,31.));
#93473=CARTESIAN_POINT('',(106.702771989219,16.1953828688963,31.));
#93474=CARTESIAN_POINT('',(106.702771989219,16.1953828688963,26.));
#93475=CARTESIAN_POINT('',(106.702771989219,16.1953828688963,31.));
#93476=CARTESIAN_POINT('',(106.702771989219,16.1953828688963,26.));
#93477=CARTESIAN_POINT('Origin',(106.39245070361,16.9445647253073,31.));
#93478=CARTESIAN_POINT('',(106.39245070361,16.9445647253073,26.));
#93479=CARTESIAN_POINT('',(106.904746769447,17.0944435750604,26.));
#93480=CARTESIAN_POINT('',(106.39245070361,16.9445647253073,31.));
#93481=CARTESIAN_POINT('',(106.39245070361,16.9445647253073,31.));
#93482=CARTESIAN_POINT('',(106.904746769447,17.0944435750604,31.));
#93483=CARTESIAN_POINT('Ctrl Pts',(105.789599926104,16.4117521548133,31.));
#93484=CARTESIAN_POINT('Ctrl Pts',(105.789599926104,16.4117521548133,26.));
#93485=CARTESIAN_POINT('Ctrl Pts',(105.793902499401,16.4176479892937,31.));
#93486=CARTESIAN_POINT('Ctrl Pts',(105.793902499401,16.4176479892937,26.));
#93487=CARTESIAN_POINT('Ctrl Pts',(105.80251540703,16.4293684717013,31.));
#93488=CARTESIAN_POINT('Ctrl Pts',(105.80251540703,16.4293684717013,26.));
#93489=CARTESIAN_POINT('Ctrl Pts',(105.815458051595,16.4467356359271,31.));
#93490=CARTESIAN_POINT('Ctrl Pts',(105.815458051595,16.4467356359271,26.));
#93491=CARTESIAN_POINT('Ctrl Pts',(105.832761561427,16.4694639603885,31.));
#93492=CARTESIAN_POINT('Ctrl Pts',(105.832761561427,16.4694639603885,26.));
#93493=CARTESIAN_POINT('Ctrl Pts',(105.854468732543,16.4971564731453,31.));
#93494=CARTESIAN_POINT('Ctrl Pts',(105.854468732543,16.4971564731453,26.));
#93495=CARTESIAN_POINT('Ctrl Pts',(105.876252925984,16.5241246895858,31.));
#93496=CARTESIAN_POINT('Ctrl Pts',(105.876252925984,16.5241246895858,26.));
#93497=CARTESIAN_POINT('Ctrl Pts',(105.898111964153,16.5503618585695,31.));
#93498=CARTESIAN_POINT('Ctrl Pts',(105.898111964153,16.5503618585695,26.));
#93499=CARTESIAN_POINT('Ctrl Pts',(105.920041584957,16.5758621107647,31.));
#93500=CARTESIAN_POINT('Ctrl Pts',(105.920041584957,16.5758621107647,26.));
#93501=CARTESIAN_POINT('Ctrl Pts',(105.942034818016,16.6006223107948,31.));
#93502=CARTESIAN_POINT('Ctrl Pts',(105.942034818016,16.6006223107948,26.));
#93503=CARTESIAN_POINT('Ctrl Pts',(105.964080995658,16.6246410138719,31.));
#93504=CARTESIAN_POINT('Ctrl Pts',(105.964080995658,16.6246410138719,26.));
#93505=CARTESIAN_POINT('Ctrl Pts',(105.986164744977,16.6479167036358,31.));
#93506=CARTESIAN_POINT('Ctrl Pts',(105.986164744977,16.6479167036358,26.));
#93507=CARTESIAN_POINT('Ctrl Pts',(106.008264745793,16.6704463289922,31.));
#93508=CARTESIAN_POINT('Ctrl Pts',(106.008264745793,16.6704463289922,26.));
#93509=CARTESIAN_POINT('Ctrl Pts',(106.03035297595,16.6922240878588,31.));
#93510=CARTESIAN_POINT('Ctrl Pts',(106.03035297595,16.6922240878588,26.));
#93511=CARTESIAN_POINT('Ctrl Pts',(106.052392594348,16.7132397086437,31.));
#93512=CARTESIAN_POINT('Ctrl Pts',(106.052392594348,16.7132397086437,26.));
#93513=CARTESIAN_POINT('Ctrl Pts',(106.074341302863,16.733479537944,31.));
#93514=CARTESIAN_POINT('Ctrl Pts',(106.074341302863,16.733479537944,26.));
#93515=CARTESIAN_POINT('Ctrl Pts',(106.096157838315,16.7529293275796,31.));
#93516=CARTESIAN_POINT('Ctrl Pts',(106.096157838315,16.7529293275796,26.));
#93517=CARTESIAN_POINT('Ctrl Pts',(106.117808186123,16.7715769312133,31.));
#93518=CARTESIAN_POINT('Ctrl Pts',(106.117808186123,16.7715769312133,26.));
#93519=CARTESIAN_POINT('Ctrl Pts',(106.139270546029,16.7894146140322,31.));
#93520=CARTESIAN_POINT('Ctrl Pts',(106.139270546029,16.7894146140322,26.));
#93521=CARTESIAN_POINT('Ctrl Pts',(106.160544466144,16.8064432225185,31.));
#93522=CARTESIAN_POINT('Ctrl Pts',(106.160544466144,16.8064432225185,26.));
#93523=CARTESIAN_POINT('Ctrl Pts',(106.181644078043,16.8226697288425,31.));
#93524=CARTESIAN_POINT('Ctrl Pts',(106.181644078043,16.8226697288425,26.));
#93525=CARTESIAN_POINT('Ctrl Pts',(106.202577977579,16.8380991844595,31.));
#93526=CARTESIAN_POINT('Ctrl Pts',(106.202577977579,16.8380991844595,26.));
#93527=CARTESIAN_POINT('Ctrl Pts',(106.22333166632,16.8527279417898,31.));
#93528=CARTESIAN_POINT('Ctrl Pts',(106.22333166632,16.8527279417898,26.));
#93529=CARTESIAN_POINT('Ctrl Pts',(106.243851491477,16.866537479377,31.));
#93530=CARTESIAN_POINT('Ctrl Pts',(106.243851491477,16.866537479377,26.));
#93531=CARTESIAN_POINT('Ctrl Pts',(106.264021191832,16.8794855787969,31.));
#93532=CARTESIAN_POINT('Ctrl Pts',(106.264021191832,16.8794855787969,26.));
#93533=CARTESIAN_POINT('Ctrl Pts',(106.283668650636,16.8915090052018,31.));
#93534=CARTESIAN_POINT('Ctrl Pts',(106.283668650636,16.8915090052018,26.));
#93535=CARTESIAN_POINT('Ctrl Pts',(106.302596915689,16.9025354335354,31.));
#93536=CARTESIAN_POINT('Ctrl Pts',(106.302596915689,16.9025354335354,26.));
#93537=CARTESIAN_POINT('Ctrl Pts',(106.320609229236,16.912493288848,31.));
#93538=CARTESIAN_POINT('Ctrl Pts',(106.320609229236,16.912493288848,26.));
#93539=CARTESIAN_POINT('Ctrl Pts',(106.337534235312,16.9213216243828,31.));
#93540=CARTESIAN_POINT('Ctrl Pts',(106.337534235312,16.9213216243828,26.));
#93541=CARTESIAN_POINT('Ctrl Pts',(106.353257428443,16.9289828368596,31.));
#93542=CARTESIAN_POINT('Ctrl Pts',(106.353257428443,16.9289828368596,26.));
#93543=CARTESIAN_POINT('Ctrl Pts',(106.367718220975,16.9354607407975,31.));
#93544=CARTESIAN_POINT('Ctrl Pts',(106.367718220975,16.9354607407975,26.));
#93545=CARTESIAN_POINT('Ctrl Pts',(106.378256564321,16.9396937165682,31.));
#93546=CARTESIAN_POINT('Ctrl Pts',(106.378256564321,16.9396937165682,26.));
#93547=CARTESIAN_POINT('Ctrl Pts',(106.385579220845,16.9423359385813,31.));
#93548=CARTESIAN_POINT('Ctrl Pts',(106.385579220845,16.9423359385813,26.));
#93549=CARTESIAN_POINT('Ctrl Pts',(106.390203177829,16.9438611710006,31.));
#93550=CARTESIAN_POINT('Ctrl Pts',(106.390203177829,16.9438611710006,26.));
#93551=CARTESIAN_POINT('Ctrl Pts',(106.39245070361,16.9445647253073,31.));
#93552=CARTESIAN_POINT('Ctrl Pts',(106.39245070361,16.9445647253073,26.));
#93553=CARTESIAN_POINT('',(105.789599926104,16.4117521548133,31.));
#93554=CARTESIAN_POINT('Ctrl Pts',(106.39245070361,16.9445647253073,31.));
#93555=CARTESIAN_POINT('Ctrl Pts',(106.390203177829,16.9438611710006,31.));
#93556=CARTESIAN_POINT('Ctrl Pts',(106.385579220845,16.9423359385813,31.));
#93557=CARTESIAN_POINT('Ctrl Pts',(106.378256564321,16.9396937165682,31.));
#93558=CARTESIAN_POINT('Ctrl Pts',(106.367718220975,16.9354607407975,31.));
#93559=CARTESIAN_POINT('Ctrl Pts',(106.353257428443,16.9289828368596,31.));
#93560=CARTESIAN_POINT('Ctrl Pts',(106.337534235312,16.9213216243828,31.));
#93561=CARTESIAN_POINT('Ctrl Pts',(106.320609229236,16.912493288848,31.));
#93562=CARTESIAN_POINT('Ctrl Pts',(106.302596915689,16.9025354335354,31.));
#93563=CARTESIAN_POINT('Ctrl Pts',(106.283668650636,16.8915090052018,31.));
#93564=CARTESIAN_POINT('Ctrl Pts',(106.264021191832,16.8794855787969,31.));
#93565=CARTESIAN_POINT('Ctrl Pts',(106.243851491477,16.866537479377,31.));
#93566=CARTESIAN_POINT('Ctrl Pts',(106.22333166632,16.8527279417898,31.));
#93567=CARTESIAN_POINT('Ctrl Pts',(106.202577977579,16.8380991844595,31.));
#93568=CARTESIAN_POINT('Ctrl Pts',(106.181644078043,16.8226697288425,31.));
#93569=CARTESIAN_POINT('Ctrl Pts',(106.160544466144,16.8064432225185,31.));
#93570=CARTESIAN_POINT('Ctrl Pts',(106.139270546029,16.7894146140322,31.));
#93571=CARTESIAN_POINT('Ctrl Pts',(106.117808186123,16.7715769312133,31.));
#93572=CARTESIAN_POINT('Ctrl Pts',(106.096157838315,16.7529293275796,31.));
#93573=CARTESIAN_POINT('Ctrl Pts',(106.074341302863,16.733479537944,31.));
#93574=CARTESIAN_POINT('Ctrl Pts',(106.052392594348,16.7132397086437,31.));
#93575=CARTESIAN_POINT('Ctrl Pts',(106.03035297595,16.6922240878588,31.));
#93576=CARTESIAN_POINT('Ctrl Pts',(106.008264745793,16.6704463289922,31.));
#93577=CARTESIAN_POINT('Ctrl Pts',(105.986164744977,16.6479167036358,31.));
#93578=CARTESIAN_POINT('Ctrl Pts',(105.964080995658,16.6246410138719,31.));
#93579=CARTESIAN_POINT('Ctrl Pts',(105.942034818016,16.6006223107948,31.));
#93580=CARTESIAN_POINT('Ctrl Pts',(105.920041584957,16.5758621107647,31.));
#93581=CARTESIAN_POINT('Ctrl Pts',(105.898111964153,16.5503618585695,31.));
#93582=CARTESIAN_POINT('Ctrl Pts',(105.876252925984,16.5241246895858,31.));
#93583=CARTESIAN_POINT('Ctrl Pts',(105.854468732543,16.4971564731453,31.));
#93584=CARTESIAN_POINT('Ctrl Pts',(105.832761561427,16.4694639603885,31.));
#93585=CARTESIAN_POINT('Ctrl Pts',(105.815458051595,16.4467356359271,31.));
#93586=CARTESIAN_POINT('Ctrl Pts',(105.80251540703,16.4293684717013,31.));
#93587=CARTESIAN_POINT('Ctrl Pts',(105.793902499401,16.4176479892937,31.));
#93588=CARTESIAN_POINT('Ctrl Pts',(105.789599926104,16.4117521548133,31.));
#93589=CARTESIAN_POINT('',(105.789599926104,16.4117521548133,26.));
#93590=CARTESIAN_POINT('Ctrl Pts',(105.789599926104,16.4117521548133,26.));
#93591=CARTESIAN_POINT('Ctrl Pts',(105.793902499401,16.4176479892937,26.));
#93592=CARTESIAN_POINT('Ctrl Pts',(105.80251540703,16.4293684717013,26.));
#93593=CARTESIAN_POINT('Ctrl Pts',(105.815458051595,16.4467356359271,26.));
#93594=CARTESIAN_POINT('Ctrl Pts',(105.832761561427,16.4694639603885,26.));
#93595=CARTESIAN_POINT('Ctrl Pts',(105.854468732543,16.4971564731453,26.));
#93596=CARTESIAN_POINT('Ctrl Pts',(105.876252925984,16.5241246895858,26.));
#93597=CARTESIAN_POINT('Ctrl Pts',(105.898111964153,16.5503618585695,26.));
#93598=CARTESIAN_POINT('Ctrl Pts',(105.920041584957,16.5758621107647,26.));
#93599=CARTESIAN_POINT('Ctrl Pts',(105.942034818016,16.6006223107948,26.));
#93600=CARTESIAN_POINT('Ctrl Pts',(105.964080995658,16.6246410138719,26.));
#93601=CARTESIAN_POINT('Ctrl Pts',(105.986164744977,16.6479167036358,26.));
#93602=CARTESIAN_POINT('Ctrl Pts',(106.008264745793,16.6704463289922,26.));
#93603=CARTESIAN_POINT('Ctrl Pts',(106.03035297595,16.6922240878588,26.));
#93604=CARTESIAN_POINT('Ctrl Pts',(106.052392594348,16.7132397086437,26.));
#93605=CARTESIAN_POINT('Ctrl Pts',(106.074341302863,16.733479537944,26.));
#93606=CARTESIAN_POINT('Ctrl Pts',(106.096157838315,16.7529293275796,26.));
#93607=CARTESIAN_POINT('Ctrl Pts',(106.117808186123,16.7715769312133,26.));
#93608=CARTESIAN_POINT('Ctrl Pts',(106.139270546029,16.7894146140322,26.));
#93609=CARTESIAN_POINT('Ctrl Pts',(106.160544466144,16.8064432225185,26.));
#93610=CARTESIAN_POINT('Ctrl Pts',(106.181644078043,16.8226697288425,26.));
#93611=CARTESIAN_POINT('Ctrl Pts',(106.202577977579,16.8380991844595,26.));
#93612=CARTESIAN_POINT('Ctrl Pts',(106.22333166632,16.8527279417898,26.));
#93613=CARTESIAN_POINT('Ctrl Pts',(106.243851491477,16.866537479377,26.));
#93614=CARTESIAN_POINT('Ctrl Pts',(106.264021191832,16.8794855787969,26.));
#93615=CARTESIAN_POINT('Ctrl Pts',(106.283668650636,16.8915090052018,26.));
#93616=CARTESIAN_POINT('Ctrl Pts',(106.302596915689,16.9025354335354,26.));
#93617=CARTESIAN_POINT('Ctrl Pts',(106.320609229236,16.912493288848,26.));
#93618=CARTESIAN_POINT('Ctrl Pts',(106.337534235312,16.9213216243828,26.));
#93619=CARTESIAN_POINT('Ctrl Pts',(106.353257428443,16.9289828368596,26.));
#93620=CARTESIAN_POINT('Ctrl Pts',(106.367718220975,16.9354607407975,26.));
#93621=CARTESIAN_POINT('Ctrl Pts',(106.378256564321,16.9396937165682,26.));
#93622=CARTESIAN_POINT('Ctrl Pts',(106.385579220845,16.9423359385813,26.));
#93623=CARTESIAN_POINT('Ctrl Pts',(106.390203177829,16.9438611710006,26.));
#93624=CARTESIAN_POINT('Ctrl Pts',(106.39245070361,16.9445647253073,26.));
#93625=CARTESIAN_POINT('',(105.789599926104,16.4117521548133,31.));
#93626=CARTESIAN_POINT('Origin',(110.000000000003,18.0000000000012,31.));
#93627=CARTESIAN_POINT('',(105.899736734704,16.1458583777765,31.));
#93628=CARTESIAN_POINT('Origin',(110.000000000003,18.0000000000012,31.));
#93629=CARTESIAN_POINT('',(105.899736734704,16.1458583777765,26.));
#93630=CARTESIAN_POINT('Origin',(110.000000000003,18.0000000000012,26.));
#93631=CARTESIAN_POINT('',(105.899736734704,16.1458583777765,31.));
#93632=CARTESIAN_POINT('Ctrl Pts',(106.702771989219,16.1953828688963,31.));
#93633=CARTESIAN_POINT('Ctrl Pts',(106.702771989219,16.1953828688963,26.));
#93634=CARTESIAN_POINT('Ctrl Pts',(106.70068526048,16.1942911161916,31.));
#93635=CARTESIAN_POINT('Ctrl Pts',(106.70068526048,16.1942911161916,26.));
#93636=CARTESIAN_POINT('Ctrl Pts',(106.696337126957,16.1920999870287,31.));
#93637=CARTESIAN_POINT('Ctrl Pts',(106.696337126957,16.1920999870287,26.));
#93638=CARTESIAN_POINT('Ctrl Pts',(106.689290893774,16.1887904200375,31.));
#93639=CARTESIAN_POINT('Ctrl Pts',(106.689290893774,16.1887904200375,26.));
#93640=CARTESIAN_POINT('Ctrl Pts',(106.678845993861,16.1843318518623,31.));
#93641=CARTESIAN_POINT('Ctrl Pts',(106.678845993861,16.1843318518623,26.));
#93642=CARTESIAN_POINT('Ctrl Pts',(106.664040099595,16.1786870972096,31.));
#93643=CARTESIAN_POINT('Ctrl Pts',(106.664040099595,16.1786870972096,26.));
#93644=CARTESIAN_POINT('Ctrl Pts',(106.647504827811,16.1729864160331,31.));
#93645=CARTESIAN_POINT('Ctrl Pts',(106.647504827811,16.1729864160331,26.));
#93646=CARTESIAN_POINT('Ctrl Pts',(106.629294465314,16.1672612054047,31.));
#93647=CARTESIAN_POINT('Ctrl Pts',(106.629294465314,16.1672612054047,26.));
#93648=CARTESIAN_POINT('Ctrl Pts',(106.609516569238,16.1615658433815,31.));
#93649=CARTESIAN_POINT('Ctrl Pts',(106.609516569238,16.1615658433815,26.));
#93650=CARTESIAN_POINT('Ctrl Pts',(106.588335402414,16.1559784010579,31.));
#93651=CARTESIAN_POINT('Ctrl Pts',(106.588335402414,16.1559784010579,26.));
#93652=CARTESIAN_POINT('Ctrl Pts',(106.565940704718,16.1505873960435,31.));
#93653=CARTESIAN_POINT('Ctrl Pts',(106.565940704718,16.1505873960435,26.));
#93654=CARTESIAN_POINT('Ctrl Pts',(106.542522883923,16.1454809530401,31.));
#93655=CARTESIAN_POINT('Ctrl Pts',(106.542522883923,16.1454809530401,26.));
#93656=CARTESIAN_POINT('Ctrl Pts',(106.518248358739,16.1407360631828,31.));
#93657=CARTESIAN_POINT('Ctrl Pts',(106.518248358739,16.1407360631828,26.));
#93658=CARTESIAN_POINT('Ctrl Pts',(106.493229191191,16.136405082636,31.));
#93659=CARTESIAN_POINT('Ctrl Pts',(106.493229191191,16.136405082636,26.));
#93660=CARTESIAN_POINT('Ctrl Pts',(106.467516416179,16.1325128530083,31.));
#93661=CARTESIAN_POINT('Ctrl Pts',(106.467516416179,16.1325128530083,26.));
#93662=CARTESIAN_POINT('Ctrl Pts',(106.441122864867,16.1290670470128,31.));
#93663=CARTESIAN_POINT('Ctrl Pts',(106.441122864867,16.1290670470128,26.));
#93664=CARTESIAN_POINT('Ctrl Pts',(106.414038887152,16.1260651583832,31.));
#93665=CARTESIAN_POINT('Ctrl Pts',(106.414038887152,16.1260651583832,26.));
#93666=CARTESIAN_POINT('Ctrl Pts',(106.386249560432,16.1235021246537,31.));
#93667=CARTESIAN_POINT('Ctrl Pts',(106.386249560432,16.1235021246537,26.));
#93668=CARTESIAN_POINT('Ctrl Pts',(106.357754605692,16.1213788639067,31.));
#93669=CARTESIAN_POINT('Ctrl Pts',(106.357754605692,16.1213788639067,26.));
#93670=CARTESIAN_POINT('Ctrl Pts',(106.328574907382,16.1197053219033,31.));
#93671=CARTESIAN_POINT('Ctrl Pts',(106.328574907382,16.1197053219033,26.));
#93672=CARTESIAN_POINT('Ctrl Pts',(106.298743106205,16.1184969618219,31.));
#93673=CARTESIAN_POINT('Ctrl Pts',(106.298743106205,16.1184969618219,26.));
#93674=CARTESIAN_POINT('Ctrl Pts',(106.26829845462,16.1177728861474,31.));
#93675=CARTESIAN_POINT('Ctrl Pts',(106.26829845462,16.1177728861474,26.));
#93676=CARTESIAN_POINT('Ctrl Pts',(106.237280516333,16.1175533497575,31.));
#93677=CARTESIAN_POINT('Ctrl Pts',(106.237280516333,16.1175533497575,26.));
#93678=CARTESIAN_POINT('Ctrl Pts',(106.205722605043,16.1178571401407,31.));
#93679=CARTESIAN_POINT('Ctrl Pts',(106.205722605043,16.1178571401407,26.));
#93680=CARTESIAN_POINT('Ctrl Pts',(106.17364863809,16.1186999692782,31.));
#93681=CARTESIAN_POINT('Ctrl Pts',(106.17364863809,16.1186999692782,26.));
#93682=CARTESIAN_POINT('Ctrl Pts',(106.141075848562,16.1200947553829,31.));
#93683=CARTESIAN_POINT('Ctrl Pts',(106.141075848562,16.1200947553829,26.));
#93684=CARTESIAN_POINT('Ctrl Pts',(106.108016178967,16.1220512965248,31.));
#93685=CARTESIAN_POINT('Ctrl Pts',(106.108016178967,16.1220512965248,26.));
#93686=CARTESIAN_POINT('Ctrl Pts',(106.074478194107,16.1245761142702,31.));
#93687=CARTESIAN_POINT('Ctrl Pts',(106.074478194107,16.1245761142702,26.));
#93688=CARTESIAN_POINT('Ctrl Pts',(106.040469039837,16.1276719203621,31.));
#93689=CARTESIAN_POINT('Ctrl Pts',(106.040469039837,16.1276719203621,26.));
#93690=CARTESIAN_POINT('Ctrl Pts',(106.00599588017,16.131337578276,31.));
#93691=CARTESIAN_POINT('Ctrl Pts',(106.00599588017,16.131337578276,26.));
#93692=CARTESIAN_POINT('Ctrl Pts',(105.971065028696,16.1355698539851,31.));
#93693=CARTESIAN_POINT('Ctrl Pts',(105.971065028696,16.1355698539851,26.));
#93694=CARTESIAN_POINT('Ctrl Pts',(105.942758247219,16.1394057771583,31.));
#93695=CARTESIAN_POINT('Ctrl Pts',(105.942758247219,16.1394057771583,26.));
#93696=CARTESIAN_POINT('Ctrl Pts',(105.921325975923,16.1425343849267,31.));
#93697=CARTESIAN_POINT('Ctrl Pts',(105.921325975923,16.1425343849267,26.));
#93698=CARTESIAN_POINT('Ctrl Pts',(105.90694809798,16.1447317720396,31.));
#93699=CARTESIAN_POINT('Ctrl Pts',(105.90694809798,16.1447317720396,26.));
#93700=CARTESIAN_POINT('Ctrl Pts',(105.899736734704,16.1458583777765,31.));
#93701=CARTESIAN_POINT('Ctrl Pts',(105.899736734704,16.1458583777765,26.));
#93702=CARTESIAN_POINT('Ctrl Pts',(106.702771989219,16.1953828688963,31.));
#93703=CARTESIAN_POINT('Ctrl Pts',(106.70068526048,16.1942911161916,31.));
#93704=CARTESIAN_POINT('Ctrl Pts',(106.696337126957,16.1920999870287,31.));
#93705=CARTESIAN_POINT('Ctrl Pts',(106.689290893774,16.1887904200375,31.));
#93706=CARTESIAN_POINT('Ctrl Pts',(106.678845993861,16.1843318518623,31.));
#93707=CARTESIAN_POINT('Ctrl Pts',(106.664040099595,16.1786870972096,31.));
#93708=CARTESIAN_POINT('Ctrl Pts',(106.647504827811,16.1729864160331,31.));
#93709=CARTESIAN_POINT('Ctrl Pts',(106.629294465314,16.1672612054047,31.));
#93710=CARTESIAN_POINT('Ctrl Pts',(106.609516569238,16.1615658433815,31.));
#93711=CARTESIAN_POINT('Ctrl Pts',(106.588335402414,16.1559784010579,31.));
#93712=CARTESIAN_POINT('Ctrl Pts',(106.565940704718,16.1505873960435,31.));
#93713=CARTESIAN_POINT('Ctrl Pts',(106.542522883923,16.1454809530401,31.));
#93714=CARTESIAN_POINT('Ctrl Pts',(106.518248358739,16.1407360631828,31.));
#93715=CARTESIAN_POINT('Ctrl Pts',(106.493229191191,16.136405082636,31.));
#93716=CARTESIAN_POINT('Ctrl Pts',(106.467516416179,16.1325128530083,31.));
#93717=CARTESIAN_POINT('Ctrl Pts',(106.441122864867,16.1290670470128,31.));
#93718=CARTESIAN_POINT('Ctrl Pts',(106.414038887152,16.1260651583832,31.));
#93719=CARTESIAN_POINT('Ctrl Pts',(106.386249560432,16.1235021246537,31.));
#93720=CARTESIAN_POINT('Ctrl Pts',(106.357754605692,16.1213788639067,31.));
#93721=CARTESIAN_POINT('Ctrl Pts',(106.328574907382,16.1197053219033,31.));
#93722=CARTESIAN_POINT('Ctrl Pts',(106.298743106205,16.1184969618219,31.));
#93723=CARTESIAN_POINT('Ctrl Pts',(106.26829845462,16.1177728861474,31.));
#93724=CARTESIAN_POINT('Ctrl Pts',(106.237280516333,16.1175533497575,31.));
#93725=CARTESIAN_POINT('Ctrl Pts',(106.205722605043,16.1178571401407,31.));
#93726=CARTESIAN_POINT('Ctrl Pts',(106.17364863809,16.1186999692782,31.));
#93727=CARTESIAN_POINT('Ctrl Pts',(106.141075848562,16.1200947553829,31.));
#93728=CARTESIAN_POINT('Ctrl Pts',(106.108016178967,16.1220512965248,31.));
#93729=CARTESIAN_POINT('Ctrl Pts',(106.074478194107,16.1245761142702,31.));
#93730=CARTESIAN_POINT('Ctrl Pts',(106.040469039837,16.1276719203621,31.));
#93731=CARTESIAN_POINT('Ctrl Pts',(106.00599588017,16.131337578276,31.));
#93732=CARTESIAN_POINT('Ctrl Pts',(105.971065028696,16.1355698539851,31.));
#93733=CARTESIAN_POINT('Ctrl Pts',(105.942758247219,16.1394057771583,31.));
#93734=CARTESIAN_POINT('Ctrl Pts',(105.921325975923,16.1425343849267,31.));
#93735=CARTESIAN_POINT('Ctrl Pts',(105.90694809798,16.1447317720396,31.));
#93736=CARTESIAN_POINT('Ctrl Pts',(105.899736734704,16.1458583777765,31.));
#93737=CARTESIAN_POINT('Ctrl Pts',(106.702771989219,16.1953828688963,26.));
#93738=CARTESIAN_POINT('Ctrl Pts',(106.70068526048,16.1942911161916,26.));
#93739=CARTESIAN_POINT('Ctrl Pts',(106.696337126957,16.1920999870287,26.));
#93740=CARTESIAN_POINT('Ctrl Pts',(106.689290893774,16.1887904200375,26.));
#93741=CARTESIAN_POINT('Ctrl Pts',(106.678845993861,16.1843318518623,26.));
#93742=CARTESIAN_POINT('Ctrl Pts',(106.664040099595,16.1786870972096,26.));
#93743=CARTESIAN_POINT('Ctrl Pts',(106.647504827811,16.1729864160331,26.));
#93744=CARTESIAN_POINT('Ctrl Pts',(106.629294465314,16.1672612054047,26.));
#93745=CARTESIAN_POINT('Ctrl Pts',(106.609516569238,16.1615658433815,26.));
#93746=CARTESIAN_POINT('Ctrl Pts',(106.588335402414,16.1559784010579,26.));
#93747=CARTESIAN_POINT('Ctrl Pts',(106.565940704718,16.1505873960435,26.));
#93748=CARTESIAN_POINT('Ctrl Pts',(106.542522883923,16.1454809530401,26.));
#93749=CARTESIAN_POINT('Ctrl Pts',(106.518248358739,16.1407360631828,26.));
#93750=CARTESIAN_POINT('Ctrl Pts',(106.493229191191,16.136405082636,26.));
#93751=CARTESIAN_POINT('Ctrl Pts',(106.467516416179,16.1325128530083,26.));
#93752=CARTESIAN_POINT('Ctrl Pts',(106.441122864867,16.1290670470128,26.));
#93753=CARTESIAN_POINT('Ctrl Pts',(106.414038887152,16.1260651583832,26.));
#93754=CARTESIAN_POINT('Ctrl Pts',(106.386249560432,16.1235021246537,26.));
#93755=CARTESIAN_POINT('Ctrl Pts',(106.357754605692,16.1213788639067,26.));
#93756=CARTESIAN_POINT('Ctrl Pts',(106.328574907382,16.1197053219033,26.));
#93757=CARTESIAN_POINT('Ctrl Pts',(106.298743106205,16.1184969618219,26.));
#93758=CARTESIAN_POINT('Ctrl Pts',(106.26829845462,16.1177728861474,26.));
#93759=CARTESIAN_POINT('Ctrl Pts',(106.237280516333,16.1175533497575,26.));
#93760=CARTESIAN_POINT('Ctrl Pts',(106.205722605043,16.1178571401407,26.));
#93761=CARTESIAN_POINT('Ctrl Pts',(106.17364863809,16.1186999692782,26.));
#93762=CARTESIAN_POINT('Ctrl Pts',(106.141075848562,16.1200947553829,26.));
#93763=CARTESIAN_POINT('Ctrl Pts',(106.108016178967,16.1220512965248,26.));
#93764=CARTESIAN_POINT('Ctrl Pts',(106.074478194107,16.1245761142702,26.));
#93765=CARTESIAN_POINT('Ctrl Pts',(106.040469039837,16.1276719203621,26.));
#93766=CARTESIAN_POINT('Ctrl Pts',(106.00599588017,16.131337578276,26.));
#93767=CARTESIAN_POINT('Ctrl Pts',(105.971065028696,16.1355698539851,26.));
#93768=CARTESIAN_POINT('Ctrl Pts',(105.942758247219,16.1394057771583,26.));
#93769=CARTESIAN_POINT('Ctrl Pts',(105.921325975923,16.1425343849267,26.));
#93770=CARTESIAN_POINT('Ctrl Pts',(105.90694809798,16.1447317720396,26.));
#93771=CARTESIAN_POINT('Ctrl Pts',(105.899736734704,16.1458583777765,26.));
#93772=CARTESIAN_POINT('Origin',(106.440207834808,16.5254858059309,31.));
#93773=CARTESIAN_POINT('Origin',(106.793817451456,17.6521229162285,31.));
#93774=CARTESIAN_POINT('',(106.263161448981,17.5945457010101,31.));
#93775=CARTESIAN_POINT('',(106.263161448981,17.5945457010101,31.));
#93776=CARTESIAN_POINT('',(106.263161448981,17.5945457010101,26.));
#93777=CARTESIAN_POINT('',(106.263161448981,17.5945457010101,31.));
#93778=CARTESIAN_POINT('',(106.263161448981,17.5945457010101,26.));
#93779=CARTESIAN_POINT('Origin',(106.263161448981,18.4054542989899,31.));
#93780=CARTESIAN_POINT('',(106.263161448981,18.4054542989899,26.));
#93781=CARTESIAN_POINT('',(106.793817451456,18.3478770837715,26.));
#93782=CARTESIAN_POINT('',(106.263161448981,18.4054542989899,31.));
#93783=CARTESIAN_POINT('',(106.263161448981,18.4054542989899,31.));
#93784=CARTESIAN_POINT('',(106.793817451456,18.3478770837715,31.));
#93785=CARTESIAN_POINT('Ctrl Pts',(105.502301411201,18.1439006751855,31.));
#93786=CARTESIAN_POINT('Ctrl Pts',(105.502301411201,18.1439006751855,26.));
#93787=CARTESIAN_POINT('Ctrl Pts',(105.508532708783,18.1477011924717,31.));
#93788=CARTESIAN_POINT('Ctrl Pts',(105.508532708783,18.1477011924717,26.));
#93789=CARTESIAN_POINT('Ctrl Pts',(105.520975232293,18.1552334892252,31.));
#93790=CARTESIAN_POINT('Ctrl Pts',(105.520975232293,18.1552334892252,26.));
#93791=CARTESIAN_POINT('Ctrl Pts',(105.53957880272,18.1663257211454,31.));
#93792=CARTESIAN_POINT('Ctrl Pts',(105.53957880272,18.1663257211454,26.));
#93793=CARTESIAN_POINT('Ctrl Pts',(105.564262914511,18.1807021883888,31.));
#93794=CARTESIAN_POINT('Ctrl Pts',(105.564262914511,18.1807021883888,26.));
#93795=CARTESIAN_POINT('Ctrl Pts',(105.594915191446,18.1979797593792,31.));
#93796=CARTESIAN_POINT('Ctrl Pts',(105.594915191446,18.1979797593792,26.));
#93797=CARTESIAN_POINT('Ctrl Pts',(105.625361451532,18.2145586926593,31.));
#93798=CARTESIAN_POINT('Ctrl Pts',(105.625361451532,18.2145586926593,26.));
#93799=CARTESIAN_POINT('Ctrl Pts',(105.655597099378,18.2304335843199,31.));
#93800=CARTESIAN_POINT('Ctrl Pts',(105.655597099378,18.2304335843199,26.));
#93801=CARTESIAN_POINT('Ctrl Pts',(105.685615951231,18.2456006428371,31.));
#93802=CARTESIAN_POINT('Ctrl Pts',(105.685615951231,18.2456006428371,26.));
#93803=CARTESIAN_POINT('Ctrl Pts',(105.715410367441,18.26005963895,31.));
#93804=CARTESIAN_POINT('Ctrl Pts',(105.715410367441,18.26005963895,26.));
#93805=CARTESIAN_POINT('Ctrl Pts',(105.744969939469,18.27381332019,31.));
#93806=CARTESIAN_POINT('Ctrl Pts',(105.744969939469,18.27381332019,26.));
#93807=CARTESIAN_POINT('Ctrl Pts',(105.774279884316,18.2868661685787,31.));
#93808=CARTESIAN_POINT('Ctrl Pts',(105.774279884316,18.2868661685787,26.));
#93809=CARTESIAN_POINT('Ctrl Pts',(105.8033193371,18.2992235241532,31.));
#93810=CARTESIAN_POINT('Ctrl Pts',(105.8033193371,18.2992235241532,26.));
#93811=CARTESIAN_POINT('Ctrl Pts',(105.832060188363,18.3108907501027,31.));
#93812=CARTESIAN_POINT('Ctrl Pts',(105.832060188363,18.3108907501027,26.));
#93813=CARTESIAN_POINT('Ctrl Pts',(105.860464470601,18.3218724551924,31.));
#93814=CARTESIAN_POINT('Ctrl Pts',(105.860464470601,18.3218724551924,26.));
#93815=CARTESIAN_POINT('Ctrl Pts',(105.88848788051,18.3321722121141,31.));
#93816=CARTESIAN_POINT('Ctrl Pts',(105.88848788051,18.3321722121141,26.));
#93817=CARTESIAN_POINT('Ctrl Pts',(105.916086843341,18.3417926480007,31.));
#93818=CARTESIAN_POINT('Ctrl Pts',(105.916086843341,18.3417926480007,26.));
#93819=CARTESIAN_POINT('Ctrl Pts',(105.943225285516,18.3507355579176,31.));
#93820=CARTESIAN_POINT('Ctrl Pts',(105.943225285516,18.3507355579176,26.));
#93821=CARTESIAN_POINT('Ctrl Pts',(105.969880106239,18.3590021384258,31.));
#93822=CARTESIAN_POINT('Ctrl Pts',(105.969880106239,18.3590021384258,26.));
#93823=CARTESIAN_POINT('Ctrl Pts',(105.996051211954,18.3665933445037,31.));
#93824=CARTESIAN_POINT('Ctrl Pts',(105.996051211954,18.3665933445037,26.));
#93825=CARTESIAN_POINT('Ctrl Pts',(106.021754326667,18.3735102096776,31.));
#93826=CARTESIAN_POINT('Ctrl Pts',(106.021754326667,18.3735102096776,26.));
#93827=CARTESIAN_POINT('Ctrl Pts',(106.046999325018,18.3797541113929,31.));
#93828=CARTESIAN_POINT('Ctrl Pts',(106.046999325018,18.3797541113929,26.));
#93829=CARTESIAN_POINT('Ctrl Pts',(106.071771416337,18.3853272280346,31.));
#93830=CARTESIAN_POINT('Ctrl Pts',(106.071771416337,18.3853272280346,26.));
#93831=CARTESIAN_POINT('Ctrl Pts',(106.096013944053,18.3902329800424,31.));
#93832=CARTESIAN_POINT('Ctrl Pts',(106.096013944053,18.3902329800424,26.));
#93833=CARTESIAN_POINT('Ctrl Pts',(106.119603340517,18.3944768539199,31.));
#93834=CARTESIAN_POINT('Ctrl Pts',(106.119603340517,18.3944768539199,26.));
#93835=CARTESIAN_POINT('Ctrl Pts',(106.142356391658,18.3980662945134,31.));
#93836=CARTESIAN_POINT('Ctrl Pts',(106.142356391658,18.3980662945134,26.));
#93837=CARTESIAN_POINT('Ctrl Pts',(106.164063459768,18.4010098525282,31.));
#93838=CARTESIAN_POINT('Ctrl Pts',(106.164063459768,18.4010098525282,26.));
#93839=CARTESIAN_POINT('Ctrl Pts',(106.184515373837,18.4033166972663,31.));
#93840=CARTESIAN_POINT('Ctrl Pts',(106.184515373837,18.4033166972663,26.));
#93841=CARTESIAN_POINT('Ctrl Pts',(106.203530498282,18.4049960963551,31.));
#93842=CARTESIAN_POINT('Ctrl Pts',(106.203530498282,18.4049960963551,26.));
#93843=CARTESIAN_POINT('Ctrl Pts',(106.220988653688,18.4060571282417,31.));
#93844=CARTESIAN_POINT('Ctrl Pts',(106.220988653688,18.4060571282417,26.));
#93845=CARTESIAN_POINT('Ctrl Pts',(106.236827670446,18.4065080253827,31.));
#93846=CARTESIAN_POINT('Ctrl Pts',(106.236827670446,18.4065080253827,26.));
#93847=CARTESIAN_POINT('Ctrl Pts',(106.248183719867,18.4063859356555,31.));
#93848=CARTESIAN_POINT('Ctrl Pts',(106.248183719867,18.4063859356555,26.));
#93849=CARTESIAN_POINT('Ctrl Pts',(106.255960106942,18.4060247711612,31.));
#93850=CARTESIAN_POINT('Ctrl Pts',(106.255960106942,18.4060247711612,26.));
#93851=CARTESIAN_POINT('Ctrl Pts',(106.260815767337,18.4056643904459,31.));
#93852=CARTESIAN_POINT('Ctrl Pts',(106.260815767337,18.4056643904459,26.));
#93853=CARTESIAN_POINT('Ctrl Pts',(106.263161448981,18.4054542989899,31.));
#93854=CARTESIAN_POINT('Ctrl Pts',(106.263161448981,18.4054542989899,26.));
#93855=CARTESIAN_POINT('',(105.502301411201,18.1439006751855,31.));
#93856=CARTESIAN_POINT('Ctrl Pts',(106.263161448981,18.4054542989899,31.));
#93857=CARTESIAN_POINT('Ctrl Pts',(106.260815767337,18.4056643904459,31.));
#93858=CARTESIAN_POINT('Ctrl Pts',(106.255960106942,18.4060247711612,31.));
#93859=CARTESIAN_POINT('Ctrl Pts',(106.248183719867,18.4063859356555,31.));
#93860=CARTESIAN_POINT('Ctrl Pts',(106.236827670446,18.4065080253827,31.));
#93861=CARTESIAN_POINT('Ctrl Pts',(106.220988653688,18.4060571282417,31.));
#93862=CARTESIAN_POINT('Ctrl Pts',(106.203530498282,18.4049960963551,31.));
#93863=CARTESIAN_POINT('Ctrl Pts',(106.184515373837,18.4033166972663,31.));
#93864=CARTESIAN_POINT('Ctrl Pts',(106.164063459768,18.4010098525282,31.));
#93865=CARTESIAN_POINT('Ctrl Pts',(106.142356391658,18.3980662945134,31.));
#93866=CARTESIAN_POINT('Ctrl Pts',(106.119603340517,18.3944768539199,31.));
#93867=CARTESIAN_POINT('Ctrl Pts',(106.096013944053,18.3902329800424,31.));
#93868=CARTESIAN_POINT('Ctrl Pts',(106.071771416337,18.3853272280346,31.));
#93869=CARTESIAN_POINT('Ctrl Pts',(106.046999325018,18.3797541113929,31.));
#93870=CARTESIAN_POINT('Ctrl Pts',(106.021754326667,18.3735102096776,31.));
#93871=CARTESIAN_POINT('Ctrl Pts',(105.996051211954,18.3665933445037,31.));
#93872=CARTESIAN_POINT('Ctrl Pts',(105.969880106239,18.3590021384258,31.));
#93873=CARTESIAN_POINT('Ctrl Pts',(105.943225285516,18.3507355579176,31.));
#93874=CARTESIAN_POINT('Ctrl Pts',(105.916086843341,18.3417926480007,31.));
#93875=CARTESIAN_POINT('Ctrl Pts',(105.88848788051,18.3321722121141,31.));
#93876=CARTESIAN_POINT('Ctrl Pts',(105.860464470601,18.3218724551924,31.));
#93877=CARTESIAN_POINT('Ctrl Pts',(105.832060188363,18.3108907501027,31.));
#93878=CARTESIAN_POINT('Ctrl Pts',(105.8033193371,18.2992235241532,31.));
#93879=CARTESIAN_POINT('Ctrl Pts',(105.774279884316,18.2868661685787,31.));
#93880=CARTESIAN_POINT('Ctrl Pts',(105.744969939469,18.27381332019,31.));
#93881=CARTESIAN_POINT('Ctrl Pts',(105.715410367441,18.26005963895,31.));
#93882=CARTESIAN_POINT('Ctrl Pts',(105.685615951231,18.2456006428371,31.));
#93883=CARTESIAN_POINT('Ctrl Pts',(105.655597099378,18.2304335843199,31.));
#93884=CARTESIAN_POINT('Ctrl Pts',(105.625361451532,18.2145586926593,31.));
#93885=CARTESIAN_POINT('Ctrl Pts',(105.594915191446,18.1979797593792,31.));
#93886=CARTESIAN_POINT('Ctrl Pts',(105.564262914511,18.1807021883888,31.));
#93887=CARTESIAN_POINT('Ctrl Pts',(105.53957880272,18.1663257211454,31.));
#93888=CARTESIAN_POINT('Ctrl Pts',(105.520975232293,18.1552334892252,31.));
#93889=CARTESIAN_POINT('Ctrl Pts',(105.508532708783,18.1477011924717,31.));
#93890=CARTESIAN_POINT('Ctrl Pts',(105.502301411201,18.1439006751855,31.));
#93891=CARTESIAN_POINT('',(105.502301411201,18.1439006751855,26.));
#93892=CARTESIAN_POINT('Ctrl Pts',(105.502301411201,18.1439006751855,26.));
#93893=CARTESIAN_POINT('Ctrl Pts',(105.508532708783,18.1477011924717,26.));
#93894=CARTESIAN_POINT('Ctrl Pts',(105.520975232293,18.1552334892252,26.));
#93895=CARTESIAN_POINT('Ctrl Pts',(105.53957880272,18.1663257211454,26.));
#93896=CARTESIAN_POINT('Ctrl Pts',(105.564262914511,18.1807021883888,26.));
#93897=CARTESIAN_POINT('Ctrl Pts',(105.594915191446,18.1979797593792,26.));
#93898=CARTESIAN_POINT('Ctrl Pts',(105.625361451532,18.2145586926593,26.));
#93899=CARTESIAN_POINT('Ctrl Pts',(105.655597099378,18.2304335843199,26.));
#93900=CARTESIAN_POINT('Ctrl Pts',(105.685615951231,18.2456006428371,26.));
#93901=CARTESIAN_POINT('Ctrl Pts',(105.715410367441,18.26005963895,26.));
#93902=CARTESIAN_POINT('Ctrl Pts',(105.744969939469,18.27381332019,26.));
#93903=CARTESIAN_POINT('Ctrl Pts',(105.774279884316,18.2868661685787,26.));
#93904=CARTESIAN_POINT('Ctrl Pts',(105.8033193371,18.2992235241532,26.));
#93905=CARTESIAN_POINT('Ctrl Pts',(105.832060188363,18.3108907501027,26.));
#93906=CARTESIAN_POINT('Ctrl Pts',(105.860464470601,18.3218724551924,26.));
#93907=CARTESIAN_POINT('Ctrl Pts',(105.88848788051,18.3321722121141,26.));
#93908=CARTESIAN_POINT('Ctrl Pts',(105.916086843341,18.3417926480007,26.));
#93909=CARTESIAN_POINT('Ctrl Pts',(105.943225285516,18.3507355579176,26.));
#93910=CARTESIAN_POINT('Ctrl Pts',(105.969880106239,18.3590021384258,26.));
#93911=CARTESIAN_POINT('Ctrl Pts',(105.996051211954,18.3665933445037,26.));
#93912=CARTESIAN_POINT('Ctrl Pts',(106.021754326667,18.3735102096776,26.));
#93913=CARTESIAN_POINT('Ctrl Pts',(106.046999325018,18.3797541113929,26.));
#93914=CARTESIAN_POINT('Ctrl Pts',(106.071771416337,18.3853272280346,26.));
#93915=CARTESIAN_POINT('Ctrl Pts',(106.096013944053,18.3902329800424,26.));
#93916=CARTESIAN_POINT('Ctrl Pts',(106.119603340517,18.3944768539199,26.));
#93917=CARTESIAN_POINT('Ctrl Pts',(106.142356391658,18.3980662945134,26.));
#93918=CARTESIAN_POINT('Ctrl Pts',(106.164063459768,18.4010098525282,26.));
#93919=CARTESIAN_POINT('Ctrl Pts',(106.184515373837,18.4033166972663,26.));
#93920=CARTESIAN_POINT('Ctrl Pts',(106.203530498282,18.4049960963551,26.));
#93921=CARTESIAN_POINT('Ctrl Pts',(106.220988653688,18.4060571282417,26.));
#93922=CARTESIAN_POINT('Ctrl Pts',(106.236827670446,18.4065080253827,26.));
#93923=CARTESIAN_POINT('Ctrl Pts',(106.248183719867,18.4063859356555,26.));
#93924=CARTESIAN_POINT('Ctrl Pts',(106.255960106942,18.4060247711612,26.));
#93925=CARTESIAN_POINT('Ctrl Pts',(106.260815767337,18.4056643904459,26.));
#93926=CARTESIAN_POINT('Ctrl Pts',(106.263161448981,18.4054542989899,26.));
#93927=CARTESIAN_POINT('',(105.502301411201,18.1439006751855,31.));
#93928=CARTESIAN_POINT('Origin',(110.000000000003,18.,31.));
#93929=CARTESIAN_POINT('',(105.502301411201,17.8560993248145,31.));
#93930=CARTESIAN_POINT('Origin',(110.000000000003,18.,31.));
#93931=CARTESIAN_POINT('',(105.502301411201,17.8560993248145,26.));
#93932=CARTESIAN_POINT('Origin',(110.000000000003,18.,26.));
#93933=CARTESIAN_POINT('',(105.502301411201,17.8560993248145,31.));
#93934=CARTESIAN_POINT('Ctrl Pts',(106.263161448981,17.5945457010101,31.));
#93935=CARTESIAN_POINT('Ctrl Pts',(106.263161448981,17.5945457010101,26.));
#93936=CARTESIAN_POINT('Ctrl Pts',(106.260815767337,17.5943356095479,31.));
#93937=CARTESIAN_POINT('Ctrl Pts',(106.260815767337,17.5943356095479,26.));
#93938=CARTESIAN_POINT('Ctrl Pts',(106.255960106942,17.593975228822,31.));
#93939=CARTESIAN_POINT('Ctrl Pts',(106.255960106942,17.593975228822,26.));
#93940=CARTESIAN_POINT('Ctrl Pts',(106.248183719866,17.5936140643173,31.));
#93941=CARTESIAN_POINT('Ctrl Pts',(106.248183719866,17.5936140643173,26.));
#93942=CARTESIAN_POINT('Ctrl Pts',(106.236827670445,17.5934919745854,31.));
#93943=CARTESIAN_POINT('Ctrl Pts',(106.236827670445,17.5934919745854,26.));
#93944=CARTESIAN_POINT('Ctrl Pts',(106.220988653687,17.5939428717324,31.));
#93945=CARTESIAN_POINT('Ctrl Pts',(106.220988653687,17.5939428717324,26.));
#93946=CARTESIAN_POINT('Ctrl Pts',(106.203530498282,17.5950039036334,31.));
#93947=CARTESIAN_POINT('Ctrl Pts',(106.203530498282,17.5950039036334,26.));
#93948=CARTESIAN_POINT('Ctrl Pts',(106.184515373837,17.5966833027395,31.));
#93949=CARTESIAN_POINT('Ctrl Pts',(106.184515373837,17.5966833027395,26.));
#93950=CARTESIAN_POINT('Ctrl Pts',(106.164063459768,17.5989901474915,31.));
#93951=CARTESIAN_POINT('Ctrl Pts',(106.164063459768,17.5989901474915,26.));
#93952=CARTESIAN_POINT('Ctrl Pts',(106.142356391658,17.6019337055115,31.));
#93953=CARTESIAN_POINT('Ctrl Pts',(106.142356391658,17.6019337055115,26.));
#93954=CARTESIAN_POINT('Ctrl Pts',(106.119603340517,17.6055231461002,31.));
#93955=CARTESIAN_POINT('Ctrl Pts',(106.119603340517,17.6055231461002,26.));
#93956=CARTESIAN_POINT('Ctrl Pts',(106.096013944054,17.6097670199654,31.));
#93957=CARTESIAN_POINT('Ctrl Pts',(106.096013944054,17.6097670199654,26.));
#93958=CARTESIAN_POINT('Ctrl Pts',(106.071771416337,17.6146727719589,31.));
#93959=CARTESIAN_POINT('Ctrl Pts',(106.071771416337,17.6146727719589,26.));
#93960=CARTESIAN_POINT('Ctrl Pts',(106.046999325018,17.6202458885881,31.));
#93961=CARTESIAN_POINT('Ctrl Pts',(106.046999325018,17.6202458885881,26.));
#93962=CARTESIAN_POINT('Ctrl Pts',(106.021754326667,17.6264897902966,31.));
#93963=CARTESIAN_POINT('Ctrl Pts',(106.021754326667,17.6264897902966,26.));
#93964=CARTESIAN_POINT('Ctrl Pts',(105.996051211954,17.6334066554725,31.));
#93965=CARTESIAN_POINT('Ctrl Pts',(105.996051211954,17.6334066554725,26.));
#93966=CARTESIAN_POINT('Ctrl Pts',(105.969880106239,17.640997861563,31.));
#93967=CARTESIAN_POINT('Ctrl Pts',(105.969880106239,17.640997861563,26.));
#93968=CARTESIAN_POINT('Ctrl Pts',(105.943225285516,17.6492644420914,31.));
#93969=CARTESIAN_POINT('Ctrl Pts',(105.943225285516,17.6492644420914,26.));
#93970=CARTESIAN_POINT('Ctrl Pts',(105.916086843341,17.6582073520301,31.));
#93971=CARTESIAN_POINT('Ctrl Pts',(105.916086843341,17.6582073520301,26.));
#93972=CARTESIAN_POINT('Ctrl Pts',(105.88848788051,17.667827787931,31.));
#93973=CARTESIAN_POINT('Ctrl Pts',(105.88848788051,17.667827787931,26.));
#93974=CARTESIAN_POINT('Ctrl Pts',(105.860464470601,17.6781275448521,31.));
#93975=CARTESIAN_POINT('Ctrl Pts',(105.860464470601,17.6781275448521,26.));
#93976=CARTESIAN_POINT('Ctrl Pts',(105.832060188363,17.6891092499218,31.));
#93977=CARTESIAN_POINT('Ctrl Pts',(105.832060188363,17.6891092499218,26.));
#93978=CARTESIAN_POINT('Ctrl Pts',(105.8033193371,17.7007764758332,31.));
#93979=CARTESIAN_POINT('Ctrl Pts',(105.8033193371,17.7007764758332,26.));
#93980=CARTESIAN_POINT('Ctrl Pts',(105.774279884316,17.7131338313612,31.));
#93981=CARTESIAN_POINT('Ctrl Pts',(105.774279884316,17.7131338313612,26.));
#93982=CARTESIAN_POINT('Ctrl Pts',(105.744969939469,17.7261866797139,31.));
#93983=CARTESIAN_POINT('Ctrl Pts',(105.744969939469,17.7261866797139,26.));
#93984=CARTESIAN_POINT('Ctrl Pts',(105.715410367441,17.7399403609466,31.));
#93985=CARTESIAN_POINT('Ctrl Pts',(105.715410367441,17.7399403609466,26.));
#93986=CARTESIAN_POINT('Ctrl Pts',(105.685615951231,17.7543993570954,31.));
#93987=CARTESIAN_POINT('Ctrl Pts',(105.685615951231,17.7543993570954,26.));
#93988=CARTESIAN_POINT('Ctrl Pts',(105.655597099378,17.7695664156946,31.));
#93989=CARTESIAN_POINT('Ctrl Pts',(105.655597099378,17.7695664156946,26.));
#93990=CARTESIAN_POINT('Ctrl Pts',(105.625361451531,17.7854413074674,31.));
#93991=CARTESIAN_POINT('Ctrl Pts',(105.625361451531,17.7854413074674,26.));
#93992=CARTESIAN_POINT('Ctrl Pts',(105.594915191446,17.8020202408531,31.));
#93993=CARTESIAN_POINT('Ctrl Pts',(105.594915191446,17.8020202408531,26.));
#93994=CARTESIAN_POINT('Ctrl Pts',(105.564262914511,17.8192978118943,31.));
#93995=CARTESIAN_POINT('Ctrl Pts',(105.564262914511,17.8192978118943,26.));
#93996=CARTESIAN_POINT('Ctrl Pts',(105.539578802719,17.8336742790972,31.));
#93997=CARTESIAN_POINT('Ctrl Pts',(105.539578802719,17.8336742790972,26.));
#93998=CARTESIAN_POINT('Ctrl Pts',(105.520975232293,17.8447665109225,31.));
#93999=CARTESIAN_POINT('Ctrl Pts',(105.520975232293,17.8447665109225,26.));
#94000=CARTESIAN_POINT('Ctrl Pts',(105.508532708783,17.8522988075826,31.));
#94001=CARTESIAN_POINT('Ctrl Pts',(105.508532708783,17.8522988075826,26.));
#94002=CARTESIAN_POINT('Ctrl Pts',(105.502301411201,17.8560993248145,31.));
#94003=CARTESIAN_POINT('Ctrl Pts',(105.502301411201,17.8560993248145,26.));
#94004=CARTESIAN_POINT('Ctrl Pts',(106.263161448981,17.5945457010101,31.));
#94005=CARTESIAN_POINT('Ctrl Pts',(106.260815767337,17.5943356095479,31.));
#94006=CARTESIAN_POINT('Ctrl Pts',(106.255960106942,17.593975228822,31.));
#94007=CARTESIAN_POINT('Ctrl Pts',(106.248183719866,17.5936140643173,31.));
#94008=CARTESIAN_POINT('Ctrl Pts',(106.236827670445,17.5934919745854,31.));
#94009=CARTESIAN_POINT('Ctrl Pts',(106.220988653687,17.5939428717324,31.));
#94010=CARTESIAN_POINT('Ctrl Pts',(106.203530498282,17.5950039036334,31.));
#94011=CARTESIAN_POINT('Ctrl Pts',(106.184515373837,17.5966833027395,31.));
#94012=CARTESIAN_POINT('Ctrl Pts',(106.164063459768,17.5989901474915,31.));
#94013=CARTESIAN_POINT('Ctrl Pts',(106.142356391658,17.6019337055115,31.));
#94014=CARTESIAN_POINT('Ctrl Pts',(106.119603340517,17.6055231461002,31.));
#94015=CARTESIAN_POINT('Ctrl Pts',(106.096013944054,17.6097670199654,31.));
#94016=CARTESIAN_POINT('Ctrl Pts',(106.071771416337,17.6146727719589,31.));
#94017=CARTESIAN_POINT('Ctrl Pts',(106.046999325018,17.6202458885881,31.));
#94018=CARTESIAN_POINT('Ctrl Pts',(106.021754326667,17.6264897902966,31.));
#94019=CARTESIAN_POINT('Ctrl Pts',(105.996051211954,17.6334066554725,31.));
#94020=CARTESIAN_POINT('Ctrl Pts',(105.969880106239,17.640997861563,31.));
#94021=CARTESIAN_POINT('Ctrl Pts',(105.943225285516,17.6492644420914,31.));
#94022=CARTESIAN_POINT('Ctrl Pts',(105.916086843341,17.6582073520301,31.));
#94023=CARTESIAN_POINT('Ctrl Pts',(105.88848788051,17.667827787931,31.));
#94024=CARTESIAN_POINT('Ctrl Pts',(105.860464470601,17.6781275448521,31.));
#94025=CARTESIAN_POINT('Ctrl Pts',(105.832060188363,17.6891092499218,31.));
#94026=CARTESIAN_POINT('Ctrl Pts',(105.8033193371,17.7007764758332,31.));
#94027=CARTESIAN_POINT('Ctrl Pts',(105.774279884316,17.7131338313612,31.));
#94028=CARTESIAN_POINT('Ctrl Pts',(105.744969939469,17.7261866797139,31.));
#94029=CARTESIAN_POINT('Ctrl Pts',(105.715410367441,17.7399403609466,31.));
#94030=CARTESIAN_POINT('Ctrl Pts',(105.685615951231,17.7543993570954,31.));
#94031=CARTESIAN_POINT('Ctrl Pts',(105.655597099378,17.7695664156946,31.));
#94032=CARTESIAN_POINT('Ctrl Pts',(105.625361451531,17.7854413074674,31.));
#94033=CARTESIAN_POINT('Ctrl Pts',(105.594915191446,17.8020202408531,31.));
#94034=CARTESIAN_POINT('Ctrl Pts',(105.564262914511,17.8192978118943,31.));
#94035=CARTESIAN_POINT('Ctrl Pts',(105.539578802719,17.8336742790972,31.));
#94036=CARTESIAN_POINT('Ctrl Pts',(105.520975232293,17.8447665109225,31.));
#94037=CARTESIAN_POINT('Ctrl Pts',(105.508532708783,17.8522988075826,31.));
#94038=CARTESIAN_POINT('Ctrl Pts',(105.502301411201,17.8560993248145,31.));
#94039=CARTESIAN_POINT('Ctrl Pts',(106.263161448981,17.5945457010101,26.));
#94040=CARTESIAN_POINT('Ctrl Pts',(106.260815767337,17.5943356095479,26.));
#94041=CARTESIAN_POINT('Ctrl Pts',(106.255960106942,17.593975228822,26.));
#94042=CARTESIAN_POINT('Ctrl Pts',(106.248183719866,17.5936140643173,26.));
#94043=CARTESIAN_POINT('Ctrl Pts',(106.236827670445,17.5934919745854,26.));
#94044=CARTESIAN_POINT('Ctrl Pts',(106.220988653687,17.5939428717324,26.));
#94045=CARTESIAN_POINT('Ctrl Pts',(106.203530498282,17.5950039036334,26.));
#94046=CARTESIAN_POINT('Ctrl Pts',(106.184515373837,17.5966833027395,26.));
#94047=CARTESIAN_POINT('Ctrl Pts',(106.164063459768,17.5989901474915,26.));
#94048=CARTESIAN_POINT('Ctrl Pts',(106.142356391658,17.6019337055115,26.));
#94049=CARTESIAN_POINT('Ctrl Pts',(106.119603340517,17.6055231461002,26.));
#94050=CARTESIAN_POINT('Ctrl Pts',(106.096013944054,17.6097670199654,26.));
#94051=CARTESIAN_POINT('Ctrl Pts',(106.071771416337,17.6146727719589,26.));
#94052=CARTESIAN_POINT('Ctrl Pts',(106.046999325018,17.6202458885881,26.));
#94053=CARTESIAN_POINT('Ctrl Pts',(106.021754326667,17.6264897902966,26.));
#94054=CARTESIAN_POINT('Ctrl Pts',(105.996051211954,17.6334066554725,26.));
#94055=CARTESIAN_POINT('Ctrl Pts',(105.969880106239,17.640997861563,26.));
#94056=CARTESIAN_POINT('Ctrl Pts',(105.943225285516,17.6492644420914,26.));
#94057=CARTESIAN_POINT('Ctrl Pts',(105.916086843341,17.6582073520301,26.));
#94058=CARTESIAN_POINT('Ctrl Pts',(105.88848788051,17.667827787931,26.));
#94059=CARTESIAN_POINT('Ctrl Pts',(105.860464470601,17.6781275448521,26.));
#94060=CARTESIAN_POINT('Ctrl Pts',(105.832060188363,17.6891092499218,26.));
#94061=CARTESIAN_POINT('Ctrl Pts',(105.8033193371,17.7007764758332,26.));
#94062=CARTESIAN_POINT('Ctrl Pts',(105.774279884316,17.7131338313612,26.));
#94063=CARTESIAN_POINT('Ctrl Pts',(105.744969939469,17.7261866797139,26.));
#94064=CARTESIAN_POINT('Ctrl Pts',(105.715410367441,17.7399403609466,26.));
#94065=CARTESIAN_POINT('Ctrl Pts',(105.685615951231,17.7543993570954,26.));
#94066=CARTESIAN_POINT('Ctrl Pts',(105.655597099378,17.7695664156946,26.));
#94067=CARTESIAN_POINT('Ctrl Pts',(105.625361451531,17.7854413074674,26.));
#94068=CARTESIAN_POINT('Ctrl Pts',(105.594915191446,17.8020202408531,26.));
#94069=CARTESIAN_POINT('Ctrl Pts',(105.564262914511,17.8192978118943,26.));
#94070=CARTESIAN_POINT('Ctrl Pts',(105.539578802719,17.8336742790972,26.));
#94071=CARTESIAN_POINT('Ctrl Pts',(105.520975232293,17.8447665109225,26.));
#94072=CARTESIAN_POINT('Ctrl Pts',(105.508532708783,17.8522988075826,26.));
#94073=CARTESIAN_POINT('Ctrl Pts',(105.502301411201,17.8560993248145,26.));
#94074=CARTESIAN_POINT('Origin',(106.146908725728,17.999999999984,31.));
#94075=CARTESIAN_POINT('Origin',(106.904746769447,18.9055564249396,31.));
#94076=CARTESIAN_POINT('',(106.39245070361,19.0554352746927,31.));
#94077=CARTESIAN_POINT('',(106.39245070361,19.0554352746927,31.));
#94078=CARTESIAN_POINT('',(106.39245070361,19.0554352746927,26.));
#94079=CARTESIAN_POINT('',(106.39245070361,19.0554352746927,31.));
#94080=CARTESIAN_POINT('',(106.39245070361,19.0554352746927,26.));
#94081=CARTESIAN_POINT('Origin',(106.702771989219,19.8046171311037,31.));
#94082=CARTESIAN_POINT('',(106.702771989219,19.8046171311037,26.));
#94083=CARTESIAN_POINT('',(107.171000362364,19.548349459992,26.));
#94084=CARTESIAN_POINT('',(106.702771989219,19.8046171311037,31.));
#94085=CARTESIAN_POINT('',(106.702771989219,19.8046171311037,31.));
#94086=CARTESIAN_POINT('',(107.171000362364,19.548349459992,31.));
#94087=CARTESIAN_POINT('Ctrl Pts',(105.899736734704,19.8541416222235,31.));
#94088=CARTESIAN_POINT('Ctrl Pts',(105.899736734704,19.8541416222235,26.));
#94089=CARTESIAN_POINT('Ctrl Pts',(105.906948098,19.8552682280105,31.));
#94090=CARTESIAN_POINT('Ctrl Pts',(105.906948098,19.8552682280105,26.));
#94091=CARTESIAN_POINT('Ctrl Pts',(105.921325975979,19.8574656152097,31.));
#94092=CARTESIAN_POINT('Ctrl Pts',(105.921325975979,19.8574656152097,26.));
#94093=CARTESIAN_POINT('Ctrl Pts',(105.942758247312,19.8605942230657,31.));
#94094=CARTESIAN_POINT('Ctrl Pts',(105.942758247312,19.8605942230657,26.));
#94095=CARTESIAN_POINT('Ctrl Pts',(105.971065028804,19.8644301462764,31.));
#94096=CARTESIAN_POINT('Ctrl Pts',(105.971065028804,19.8644301462764,26.));
#94097=CARTESIAN_POINT('Ctrl Pts',(106.005995880259,19.8686624219385,31.));
#94098=CARTESIAN_POINT('Ctrl Pts',(106.005995880259,19.8686624219385,26.));
#94099=CARTESIAN_POINT('Ctrl Pts',(106.040469039886,19.8723280797549,31.));
#94100=CARTESIAN_POINT('Ctrl Pts',(106.040469039886,19.8723280797549,26.));
#94101=CARTESIAN_POINT('Ctrl Pts',(106.074478194113,19.8754238857432,31.));
#94102=CARTESIAN_POINT('Ctrl Pts',(106.074478194113,19.8754238857432,26.));
#94103=CARTESIAN_POINT('Ctrl Pts',(106.108016178941,19.8779487034129,31.));
#94104=CARTESIAN_POINT('Ctrl Pts',(106.108016178941,19.8779487034129,26.));
#94105=CARTESIAN_POINT('Ctrl Pts',(106.141075848522,19.8799052445217,31.));
#94106=CARTESIAN_POINT('Ctrl Pts',(106.141075848522,19.8799052445217,26.));
#94107=CARTESIAN_POINT('Ctrl Pts',(106.173648638053,19.8813000306331,31.));
#94108=CARTESIAN_POINT('Ctrl Pts',(106.173648638053,19.8813000306331,26.));
#94109=CARTESIAN_POINT('Ctrl Pts',(106.20572260502,19.8821428598039,31.));
#94110=CARTESIAN_POINT('Ctrl Pts',(106.20572260502,19.8821428598039,26.));
#94111=CARTESIAN_POINT('Ctrl Pts',(106.237280516328,19.8824466502299,31.));
#94112=CARTESIAN_POINT('Ctrl Pts',(106.237280516328,19.8824466502299,26.));
#94113=CARTESIAN_POINT('Ctrl Pts',(106.26829845463,19.8822271138752,31.));
#94114=CARTESIAN_POINT('Ctrl Pts',(106.26829845463,19.8822271138752,26.));
#94115=CARTESIAN_POINT('Ctrl Pts',(106.298743106222,19.8815030382192,31.));
#94116=CARTESIAN_POINT('Ctrl Pts',(106.298743106222,19.8815030382192,26.));
#94117=CARTESIAN_POINT('Ctrl Pts',(106.328574907399,19.8802946781383,31.));
#94118=CARTESIAN_POINT('Ctrl Pts',(106.328574907399,19.8802946781383,26.));
#94119=CARTESIAN_POINT('Ctrl Pts',(106.357754605704,19.8786211361218,31.));
#94120=CARTESIAN_POINT('Ctrl Pts',(106.357754605704,19.8786211361218,26.));
#94121=CARTESIAN_POINT('Ctrl Pts',(106.386249560435,19.8764978753546,31.));
#94122=CARTESIAN_POINT('Ctrl Pts',(106.386249560435,19.8764978753546,26.));
#94123=CARTESIAN_POINT('Ctrl Pts',(106.414038887147,19.8739348416065,31.));
#94124=CARTESIAN_POINT('Ctrl Pts',(106.414038887147,19.8739348416065,26.));
#94125=CARTESIAN_POINT('Ctrl Pts',(106.441122864858,19.8709329529652,31.));
#94126=CARTESIAN_POINT('Ctrl Pts',(106.441122864858,19.8709329529652,26.));
#94127=CARTESIAN_POINT('Ctrl Pts',(106.467516416169,19.8674871469678,31.));
#94128=CARTESIAN_POINT('Ctrl Pts',(106.467516416169,19.8674871469678,26.));
#94129=CARTESIAN_POINT('Ctrl Pts',(106.493229191184,19.8635949173464,31.));
#94130=CARTESIAN_POINT('Ctrl Pts',(106.493229191184,19.8635949173464,26.));
#94131=CARTESIAN_POINT('Ctrl Pts',(106.518248358736,19.8592639368112,31.));
#94132=CARTESIAN_POINT('Ctrl Pts',(106.518248358736,19.8592639368112,26.));
#94133=CARTESIAN_POINT('Ctrl Pts',(106.542522883926,19.8545190469672,31.));
#94134=CARTESIAN_POINT('Ctrl Pts',(106.542522883926,19.8545190469672,26.));
#94135=CARTESIAN_POINT('Ctrl Pts',(106.565940704725,19.8494126039752,31.));
#94136=CARTESIAN_POINT('Ctrl Pts',(106.565940704725,19.8494126039752,26.));
#94137=CARTESIAN_POINT('Ctrl Pts',(106.588335402423,19.8440215989653,31.));
#94138=CARTESIAN_POINT('Ctrl Pts',(106.588335402423,19.8440215989653,26.));
#94139=CARTESIAN_POINT('Ctrl Pts',(106.609516569245,19.838434156637,31.));
#94140=CARTESIAN_POINT('Ctrl Pts',(106.609516569245,19.838434156637,26.));
#94141=CARTESIAN_POINT('Ctrl Pts',(106.629294465316,19.8327387946007,31.));
#94142=CARTESIAN_POINT('Ctrl Pts',(106.629294465316,19.8327387946007,26.));
#94143=CARTESIAN_POINT('Ctrl Pts',(106.647504827807,19.8270135839562,31.));
#94144=CARTESIAN_POINT('Ctrl Pts',(106.647504827807,19.8270135839562,26.));
#94145=CARTESIAN_POINT('Ctrl Pts',(106.664040099586,19.821312902766,31.));
#94146=CARTESIAN_POINT('Ctrl Pts',(106.664040099586,19.821312902766,26.));
#94147=CARTESIAN_POINT('Ctrl Pts',(106.67884599385,19.8156681481077,31.));
#94148=CARTESIAN_POINT('Ctrl Pts',(106.67884599385,19.8156681481077,26.));
#94149=CARTESIAN_POINT('Ctrl Pts',(106.689290893764,19.811209579937,31.));
#94150=CARTESIAN_POINT('Ctrl Pts',(106.689290893764,19.811209579937,26.));
#94151=CARTESIAN_POINT('Ctrl Pts',(106.696337126951,19.8079000129555,31.));
#94152=CARTESIAN_POINT('Ctrl Pts',(106.696337126951,19.8079000129555,26.));
#94153=CARTESIAN_POINT('Ctrl Pts',(106.700685260478,19.8057088838026,31.));
#94154=CARTESIAN_POINT('Ctrl Pts',(106.700685260478,19.8057088838026,26.));
#94155=CARTESIAN_POINT('Ctrl Pts',(106.702771989219,19.8046171311037,31.));
#94156=CARTESIAN_POINT('Ctrl Pts',(106.702771989219,19.8046171311037,26.));
#94157=CARTESIAN_POINT('',(105.899736734704,19.8541416222235,31.));
#94158=CARTESIAN_POINT('Ctrl Pts',(106.702771989219,19.8046171311037,31.));
#94159=CARTESIAN_POINT('Ctrl Pts',(106.700685260478,19.8057088838026,31.));
#94160=CARTESIAN_POINT('Ctrl Pts',(106.696337126951,19.8079000129555,31.));
#94161=CARTESIAN_POINT('Ctrl Pts',(106.689290893764,19.811209579937,31.));
#94162=CARTESIAN_POINT('Ctrl Pts',(106.67884599385,19.8156681481077,31.));
#94163=CARTESIAN_POINT('Ctrl Pts',(106.664040099586,19.821312902766,31.));
#94164=CARTESIAN_POINT('Ctrl Pts',(106.647504827807,19.8270135839562,31.));
#94165=CARTESIAN_POINT('Ctrl Pts',(106.629294465316,19.8327387946007,31.));
#94166=CARTESIAN_POINT('Ctrl Pts',(106.609516569245,19.838434156637,31.));
#94167=CARTESIAN_POINT('Ctrl Pts',(106.588335402423,19.8440215989653,31.));
#94168=CARTESIAN_POINT('Ctrl Pts',(106.565940704725,19.8494126039752,31.));
#94169=CARTESIAN_POINT('Ctrl Pts',(106.542522883926,19.8545190469672,31.));
#94170=CARTESIAN_POINT('Ctrl Pts',(106.518248358736,19.8592639368112,31.));
#94171=CARTESIAN_POINT('Ctrl Pts',(106.493229191184,19.8635949173464,31.));
#94172=CARTESIAN_POINT('Ctrl Pts',(106.467516416169,19.8674871469678,31.));
#94173=CARTESIAN_POINT('Ctrl Pts',(106.441122864858,19.8709329529652,31.));
#94174=CARTESIAN_POINT('Ctrl Pts',(106.414038887147,19.8739348416065,31.));
#94175=CARTESIAN_POINT('Ctrl Pts',(106.386249560435,19.8764978753546,31.));
#94176=CARTESIAN_POINT('Ctrl Pts',(106.357754605704,19.8786211361218,31.));
#94177=CARTESIAN_POINT('Ctrl Pts',(106.328574907399,19.8802946781383,31.));
#94178=CARTESIAN_POINT('Ctrl Pts',(106.298743106222,19.8815030382192,31.));
#94179=CARTESIAN_POINT('Ctrl Pts',(106.26829845463,19.8822271138752,31.));
#94180=CARTESIAN_POINT('Ctrl Pts',(106.237280516328,19.8824466502299,31.));
#94181=CARTESIAN_POINT('Ctrl Pts',(106.20572260502,19.8821428598039,31.));
#94182=CARTESIAN_POINT('Ctrl Pts',(106.173648638053,19.8813000306331,31.));
#94183=CARTESIAN_POINT('Ctrl Pts',(106.141075848522,19.8799052445217,31.));
#94184=CARTESIAN_POINT('Ctrl Pts',(106.108016178941,19.8779487034129,31.));
#94185=CARTESIAN_POINT('Ctrl Pts',(106.074478194113,19.8754238857432,31.));
#94186=CARTESIAN_POINT('Ctrl Pts',(106.040469039886,19.8723280797549,31.));
#94187=CARTESIAN_POINT('Ctrl Pts',(106.005995880259,19.8686624219385,31.));
#94188=CARTESIAN_POINT('Ctrl Pts',(105.971065028804,19.8644301462764,31.));
#94189=CARTESIAN_POINT('Ctrl Pts',(105.942758247312,19.8605942230657,31.));
#94190=CARTESIAN_POINT('Ctrl Pts',(105.921325975979,19.8574656152097,31.));
#94191=CARTESIAN_POINT('Ctrl Pts',(105.906948098,19.8552682280105,31.));
#94192=CARTESIAN_POINT('Ctrl Pts',(105.899736734704,19.8541416222235,31.));
#94193=CARTESIAN_POINT('',(105.899736734704,19.8541416222235,26.));
#94194=CARTESIAN_POINT('Ctrl Pts',(105.899736734704,19.8541416222235,26.));
#94195=CARTESIAN_POINT('Ctrl Pts',(105.906948098,19.8552682280105,26.));
#94196=CARTESIAN_POINT('Ctrl Pts',(105.921325975979,19.8574656152097,26.));
#94197=CARTESIAN_POINT('Ctrl Pts',(105.942758247312,19.8605942230657,26.));
#94198=CARTESIAN_POINT('Ctrl Pts',(105.971065028804,19.8644301462764,26.));
#94199=CARTESIAN_POINT('Ctrl Pts',(106.005995880259,19.8686624219385,26.));
#94200=CARTESIAN_POINT('Ctrl Pts',(106.040469039886,19.8723280797549,26.));
#94201=CARTESIAN_POINT('Ctrl Pts',(106.074478194113,19.8754238857432,26.));
#94202=CARTESIAN_POINT('Ctrl Pts',(106.108016178941,19.8779487034129,26.));
#94203=CARTESIAN_POINT('Ctrl Pts',(106.141075848522,19.8799052445217,26.));
#94204=CARTESIAN_POINT('Ctrl Pts',(106.173648638053,19.8813000306331,26.));
#94205=CARTESIAN_POINT('Ctrl Pts',(106.20572260502,19.8821428598039,26.));
#94206=CARTESIAN_POINT('Ctrl Pts',(106.237280516328,19.8824466502299,26.));
#94207=CARTESIAN_POINT('Ctrl Pts',(106.26829845463,19.8822271138752,26.));
#94208=CARTESIAN_POINT('Ctrl Pts',(106.298743106222,19.8815030382192,26.));
#94209=CARTESIAN_POINT('Ctrl Pts',(106.328574907399,19.8802946781383,26.));
#94210=CARTESIAN_POINT('Ctrl Pts',(106.357754605704,19.8786211361218,26.));
#94211=CARTESIAN_POINT('Ctrl Pts',(106.386249560435,19.8764978753546,26.));
#94212=CARTESIAN_POINT('Ctrl Pts',(106.414038887147,19.8739348416065,26.));
#94213=CARTESIAN_POINT('Ctrl Pts',(106.441122864858,19.8709329529652,26.));
#94214=CARTESIAN_POINT('Ctrl Pts',(106.467516416169,19.8674871469678,26.));
#94215=CARTESIAN_POINT('Ctrl Pts',(106.493229191184,19.8635949173464,26.));
#94216=CARTESIAN_POINT('Ctrl Pts',(106.518248358736,19.8592639368112,26.));
#94217=CARTESIAN_POINT('Ctrl Pts',(106.542522883926,19.8545190469672,26.));
#94218=CARTESIAN_POINT('Ctrl Pts',(106.565940704725,19.8494126039752,26.));
#94219=CARTESIAN_POINT('Ctrl Pts',(106.588335402423,19.8440215989653,26.));
#94220=CARTESIAN_POINT('Ctrl Pts',(106.609516569245,19.838434156637,26.));
#94221=CARTESIAN_POINT('Ctrl Pts',(106.629294465316,19.8327387946007,26.));
#94222=CARTESIAN_POINT('Ctrl Pts',(106.647504827807,19.8270135839562,26.));
#94223=CARTESIAN_POINT('Ctrl Pts',(106.664040099586,19.821312902766,26.));
#94224=CARTESIAN_POINT('Ctrl Pts',(106.67884599385,19.8156681481077,26.));
#94225=CARTESIAN_POINT('Ctrl Pts',(106.689290893764,19.811209579937,26.));
#94226=CARTESIAN_POINT('Ctrl Pts',(106.696337126951,19.8079000129555,26.));
#94227=CARTESIAN_POINT('Ctrl Pts',(106.700685260478,19.8057088838026,26.));
#94228=CARTESIAN_POINT('Ctrl Pts',(106.702771989219,19.8046171311037,26.));
#94229=CARTESIAN_POINT('',(105.899736734704,19.8541416222235,31.));
#94230=CARTESIAN_POINT('Origin',(110.000000000003,17.9999999999989,31.));
#94231=CARTESIAN_POINT('',(105.789599926104,19.5882478451867,31.));
#94232=CARTESIAN_POINT('Origin',(110.000000000003,17.9999999999989,31.));
#94233=CARTESIAN_POINT('',(105.789599926104,19.5882478451867,26.));
#94234=CARTESIAN_POINT('Origin',(110.000000000003,17.9999999999989,26.));
#94235=CARTESIAN_POINT('',(105.789599926104,19.5882478451867,31.));
#94236=CARTESIAN_POINT('Ctrl Pts',(106.39245070361,19.0554352746927,31.));
#94237=CARTESIAN_POINT('Ctrl Pts',(106.39245070361,19.0554352746927,26.));
#94238=CARTESIAN_POINT('Ctrl Pts',(106.390203177827,19.0561388289937,31.));
#94239=CARTESIAN_POINT('Ctrl Pts',(106.390203177827,19.0561388289937,26.));
#94240=CARTESIAN_POINT('Ctrl Pts',(106.385579220838,19.0576640614035,31.));
#94241=CARTESIAN_POINT('Ctrl Pts',(106.385579220838,19.0576640614035,26.));
#94242=CARTESIAN_POINT('Ctrl Pts',(106.37825656431,19.0603062834071,31.));
#94243=CARTESIAN_POINT('Ctrl Pts',(106.37825656431,19.0603062834071,26.));
#94244=CARTESIAN_POINT('Ctrl Pts',(106.367718220961,19.0645392591734,31.));
#94245=CARTESIAN_POINT('Ctrl Pts',(106.367718220961,19.0645392591734,26.));
#94246=CARTESIAN_POINT('Ctrl Pts',(106.353257428432,19.0710171631169,31.));
#94247=CARTESIAN_POINT('Ctrl Pts',(106.353257428432,19.0710171631169,26.));
#94248=CARTESIAN_POINT('Ctrl Pts',(106.337534235307,19.0786783756069,31.));
#94249=CARTESIAN_POINT('Ctrl Pts',(106.337534235307,19.0786783756069,26.));
#94250=CARTESIAN_POINT('Ctrl Pts',(106.320609229239,19.0875067111573,31.));
#94251=CARTESIAN_POINT('Ctrl Pts',(106.320609229239,19.0875067111573,26.));
#94252=CARTESIAN_POINT('Ctrl Pts',(106.302596915698,19.0974645664826,31.));
#94253=CARTESIAN_POINT('Ctrl Pts',(106.302596915698,19.0974645664826,26.));
#94254=CARTESIAN_POINT('Ctrl Pts',(106.283668650646,19.108490994821,31.));
#94255=CARTESIAN_POINT('Ctrl Pts',(106.283668650646,19.108490994821,26.));
#94256=CARTESIAN_POINT('Ctrl Pts',(106.26402119184,19.1205144212215,31.));
#94257=CARTESIAN_POINT('Ctrl Pts',(106.26402119184,19.1205144212215,26.));
#94258=CARTESIAN_POINT('Ctrl Pts',(106.24385149148,19.1334625206302,31.));
#94259=CARTESIAN_POINT('Ctrl Pts',(106.24385149148,19.1334625206302,26.));
#94260=CARTESIAN_POINT('Ctrl Pts',(106.223331666318,19.1472720582043,31.));
#94261=CARTESIAN_POINT('Ctrl Pts',(106.223331666318,19.1472720582043,26.));
#94262=CARTESIAN_POINT('Ctrl Pts',(106.202577977571,19.1619008155231,31.));
#94263=CARTESIAN_POINT('Ctrl Pts',(106.202577977571,19.1619008155231,26.));
#94264=CARTESIAN_POINT('Ctrl Pts',(106.181644078033,19.1773302711338,31.));
#94265=CARTESIAN_POINT('Ctrl Pts',(106.181644078033,19.1773302711338,26.));
#94266=CARTESIAN_POINT('Ctrl Pts',(106.160544466135,19.1935567774596,31.));
#94267=CARTESIAN_POINT('Ctrl Pts',(106.160544466135,19.1935567774596,26.));
#94268=CARTESIAN_POINT('Ctrl Pts',(106.139270546025,19.2105853859574,31.));
#94269=CARTESIAN_POINT('Ctrl Pts',(106.139270546025,19.2105853859574,26.));
#94270=CARTESIAN_POINT('Ctrl Pts',(106.117808186126,19.228423068795,31.));
#94271=CARTESIAN_POINT('Ctrl Pts',(106.117808186126,19.228423068795,26.));
#94272=CARTESIAN_POINT('Ctrl Pts',(106.096157838327,19.2470706724489,31.));
#94273=CARTESIAN_POINT('Ctrl Pts',(106.096157838327,19.2470706724489,26.));
#94274=CARTESIAN_POINT('Ctrl Pts',(106.07434130288,19.2665204620976,31.));
#94275=CARTESIAN_POINT('Ctrl Pts',(106.07434130288,19.2665204620976,26.));
#94276=CARTESIAN_POINT('Ctrl Pts',(106.052392594365,19.2867602913975,31.));
#94277=CARTESIAN_POINT('Ctrl Pts',(106.052392594365,19.2867602913975,26.));
#94278=CARTESIAN_POINT('Ctrl Pts',(106.030352975959,19.3077759121639,31.));
#94279=CARTESIAN_POINT('Ctrl Pts',(106.030352975959,19.3077759121639,26.));
#94280=CARTESIAN_POINT('Ctrl Pts',(106.008264745788,19.3295536709952,31.));
#94281=CARTESIAN_POINT('Ctrl Pts',(106.008264745788,19.3295536709952,26.));
#94282=CARTESIAN_POINT('Ctrl Pts',(105.986164744955,19.3520832963087,31.));
#94283=CARTESIAN_POINT('Ctrl Pts',(105.986164744955,19.3520832963087,26.));
#94284=CARTESIAN_POINT('Ctrl Pts',(105.964080995621,19.3753589860392,31.));
#94285=CARTESIAN_POINT('Ctrl Pts',(105.964080995621,19.3753589860392,26.));
#94286=CARTESIAN_POINT('Ctrl Pts',(105.942034817977,19.3993776891096,31.));
#94287=CARTESIAN_POINT('Ctrl Pts',(105.942034817977,19.3993776891096,26.));
#94288=CARTESIAN_POINT('Ctrl Pts',(105.920041584931,19.4241378891729,31.));
#94289=CARTESIAN_POINT('Ctrl Pts',(105.920041584931,19.4241378891729,26.));
#94290=CARTESIAN_POINT('Ctrl Pts',(105.898111964159,19.4496381414438,31.));
#94291=CARTESIAN_POINT('Ctrl Pts',(105.898111964159,19.4496381414438,26.));
#94292=CARTESIAN_POINT('Ctrl Pts',(105.876252926033,19.4758753105314,31.));
#94293=CARTESIAN_POINT('Ctrl Pts',(105.876252926033,19.4758753105314,26.));
#94294=CARTESIAN_POINT('Ctrl Pts',(105.854468732632,19.5028435270694,31.));
#94295=CARTESIAN_POINT('Ctrl Pts',(105.854468732632,19.5028435270694,26.));
#94296=CARTESIAN_POINT('Ctrl Pts',(105.832761561535,19.5305360398732,31.));
#94297=CARTESIAN_POINT('Ctrl Pts',(105.832761561535,19.5305360398732,26.));
#94298=CARTESIAN_POINT('Ctrl Pts',(105.815458051687,19.5532643642971,31.));
#94299=CARTESIAN_POINT('Ctrl Pts',(105.815458051687,19.5532643642971,26.));
#94300=CARTESIAN_POINT('Ctrl Pts',(105.802515407086,19.5706315284352,31.));
#94301=CARTESIAN_POINT('Ctrl Pts',(105.802515407086,19.5706315284352,26.));
#94302=CARTESIAN_POINT('Ctrl Pts',(105.793902499422,19.5823520107564,31.));
#94303=CARTESIAN_POINT('Ctrl Pts',(105.793902499422,19.5823520107564,26.));
#94304=CARTESIAN_POINT('Ctrl Pts',(105.789599926104,19.5882478451867,31.));
#94305=CARTESIAN_POINT('Ctrl Pts',(105.789599926104,19.5882478451867,26.));
#94306=CARTESIAN_POINT('Ctrl Pts',(106.39245070361,19.0554352746927,31.));
#94307=CARTESIAN_POINT('Ctrl Pts',(106.390203177827,19.0561388289937,31.));
#94308=CARTESIAN_POINT('Ctrl Pts',(106.385579220838,19.0576640614035,31.));
#94309=CARTESIAN_POINT('Ctrl Pts',(106.37825656431,19.0603062834071,31.));
#94310=CARTESIAN_POINT('Ctrl Pts',(106.367718220961,19.0645392591734,31.));
#94311=CARTESIAN_POINT('Ctrl Pts',(106.353257428432,19.0710171631169,31.));
#94312=CARTESIAN_POINT('Ctrl Pts',(106.337534235307,19.0786783756069,31.));
#94313=CARTESIAN_POINT('Ctrl Pts',(106.320609229239,19.0875067111573,31.));
#94314=CARTESIAN_POINT('Ctrl Pts',(106.302596915698,19.0974645664826,31.));
#94315=CARTESIAN_POINT('Ctrl Pts',(106.283668650646,19.108490994821,31.));
#94316=CARTESIAN_POINT('Ctrl Pts',(106.26402119184,19.1205144212215,31.));
#94317=CARTESIAN_POINT('Ctrl Pts',(106.24385149148,19.1334625206302,31.));
#94318=CARTESIAN_POINT('Ctrl Pts',(106.223331666318,19.1472720582043,31.));
#94319=CARTESIAN_POINT('Ctrl Pts',(106.202577977571,19.1619008155231,31.));
#94320=CARTESIAN_POINT('Ctrl Pts',(106.181644078033,19.1773302711338,31.));
#94321=CARTESIAN_POINT('Ctrl Pts',(106.160544466135,19.1935567774596,31.));
#94322=CARTESIAN_POINT('Ctrl Pts',(106.139270546025,19.2105853859574,31.));
#94323=CARTESIAN_POINT('Ctrl Pts',(106.117808186126,19.228423068795,31.));
#94324=CARTESIAN_POINT('Ctrl Pts',(106.096157838327,19.2470706724489,31.));
#94325=CARTESIAN_POINT('Ctrl Pts',(106.07434130288,19.2665204620976,31.));
#94326=CARTESIAN_POINT('Ctrl Pts',(106.052392594365,19.2867602913975,31.));
#94327=CARTESIAN_POINT('Ctrl Pts',(106.030352975959,19.3077759121639,31.));
#94328=CARTESIAN_POINT('Ctrl Pts',(106.008264745788,19.3295536709952,31.));
#94329=CARTESIAN_POINT('Ctrl Pts',(105.986164744955,19.3520832963087,31.));
#94330=CARTESIAN_POINT('Ctrl Pts',(105.964080995621,19.3753589860392,31.));
#94331=CARTESIAN_POINT('Ctrl Pts',(105.942034817977,19.3993776891096,31.));
#94332=CARTESIAN_POINT('Ctrl Pts',(105.920041584931,19.4241378891729,31.));
#94333=CARTESIAN_POINT('Ctrl Pts',(105.898111964159,19.4496381414438,31.));
#94334=CARTESIAN_POINT('Ctrl Pts',(105.876252926033,19.4758753105314,31.));
#94335=CARTESIAN_POINT('Ctrl Pts',(105.854468732632,19.5028435270694,31.));
#94336=CARTESIAN_POINT('Ctrl Pts',(105.832761561535,19.5305360398732,31.));
#94337=CARTESIAN_POINT('Ctrl Pts',(105.815458051687,19.5532643642971,31.));
#94338=CARTESIAN_POINT('Ctrl Pts',(105.802515407086,19.5706315284352,31.));
#94339=CARTESIAN_POINT('Ctrl Pts',(105.793902499422,19.5823520107564,31.));
#94340=CARTESIAN_POINT('Ctrl Pts',(105.789599926104,19.5882478451867,31.));
#94341=CARTESIAN_POINT('Ctrl Pts',(106.39245070361,19.0554352746927,26.));
#94342=CARTESIAN_POINT('Ctrl Pts',(106.390203177827,19.0561388289937,26.));
#94343=CARTESIAN_POINT('Ctrl Pts',(106.385579220838,19.0576640614035,26.));
#94344=CARTESIAN_POINT('Ctrl Pts',(106.37825656431,19.0603062834071,26.));
#94345=CARTESIAN_POINT('Ctrl Pts',(106.367718220961,19.0645392591734,26.));
#94346=CARTESIAN_POINT('Ctrl Pts',(106.353257428432,19.0710171631169,26.));
#94347=CARTESIAN_POINT('Ctrl Pts',(106.337534235307,19.0786783756069,26.));
#94348=CARTESIAN_POINT('Ctrl Pts',(106.320609229239,19.0875067111573,26.));
#94349=CARTESIAN_POINT('Ctrl Pts',(106.302596915698,19.0974645664826,26.));
#94350=CARTESIAN_POINT('Ctrl Pts',(106.283668650646,19.108490994821,26.));
#94351=CARTESIAN_POINT('Ctrl Pts',(106.26402119184,19.1205144212215,26.));
#94352=CARTESIAN_POINT('Ctrl Pts',(106.24385149148,19.1334625206302,26.));
#94353=CARTESIAN_POINT('Ctrl Pts',(106.223331666318,19.1472720582043,26.));
#94354=CARTESIAN_POINT('Ctrl Pts',(106.202577977571,19.1619008155231,26.));
#94355=CARTESIAN_POINT('Ctrl Pts',(106.181644078033,19.1773302711338,26.));
#94356=CARTESIAN_POINT('Ctrl Pts',(106.160544466135,19.1935567774596,26.));
#94357=CARTESIAN_POINT('Ctrl Pts',(106.139270546025,19.2105853859574,26.));
#94358=CARTESIAN_POINT('Ctrl Pts',(106.117808186126,19.228423068795,26.));
#94359=CARTESIAN_POINT('Ctrl Pts',(106.096157838327,19.2470706724489,26.));
#94360=CARTESIAN_POINT('Ctrl Pts',(106.07434130288,19.2665204620976,26.));
#94361=CARTESIAN_POINT('Ctrl Pts',(106.052392594365,19.2867602913975,26.));
#94362=CARTESIAN_POINT('Ctrl Pts',(106.030352975959,19.3077759121639,26.));
#94363=CARTESIAN_POINT('Ctrl Pts',(106.008264745788,19.3295536709952,26.));
#94364=CARTESIAN_POINT('Ctrl Pts',(105.986164744955,19.3520832963087,26.));
#94365=CARTESIAN_POINT('Ctrl Pts',(105.964080995621,19.3753589860392,26.));
#94366=CARTESIAN_POINT('Ctrl Pts',(105.942034817977,19.3993776891096,26.));
#94367=CARTESIAN_POINT('Ctrl Pts',(105.920041584931,19.4241378891729,26.));
#94368=CARTESIAN_POINT('Ctrl Pts',(105.898111964159,19.4496381414438,26.));
#94369=CARTESIAN_POINT('Ctrl Pts',(105.876252926033,19.4758753105314,26.));
#94370=CARTESIAN_POINT('Ctrl Pts',(105.854468732632,19.5028435270694,26.));
#94371=CARTESIAN_POINT('Ctrl Pts',(105.832761561535,19.5305360398732,26.));
#94372=CARTESIAN_POINT('Ctrl Pts',(105.815458051687,19.5532643642971,26.));
#94373=CARTESIAN_POINT('Ctrl Pts',(105.802515407086,19.5706315284352,26.));
#94374=CARTESIAN_POINT('Ctrl Pts',(105.793902499422,19.5823520107564,26.));
#94375=CARTESIAN_POINT('Ctrl Pts',(105.789599926104,19.5882478451867,26.));
#94376=CARTESIAN_POINT('Origin',(106.440207834796,19.4745141940396,31.));
#94377=CARTESIAN_POINT('Origin',(107.486900333248,20.0211271768431,31.));
#94378=CARTESIAN_POINT('',(107.070956636098,20.3556443953479,31.));
#94379=CARTESIAN_POINT('',(107.070956636098,20.3556443953479,31.));
#94380=CARTESIAN_POINT('',(107.070956636098,20.3556443953479,26.));
#94381=CARTESIAN_POINT('',(107.070956636098,20.3556443953479,31.));
#94382=CARTESIAN_POINT('',(107.070956636098,20.3556443953479,26.));
#94383=CARTESIAN_POINT('Origin',(107.644355604652,20.9290433639019,31.));
#94384=CARTESIAN_POINT('',(107.644355604652,20.9290433639019,26.));
#94385=CARTESIAN_POINT('',(107.978872823157,20.5130996667515,26.));
#94386=CARTESIAN_POINT('',(107.644355604652,20.9290433639019,31.));
#94387=CARTESIAN_POINT('',(107.644355604652,20.9290433639019,31.));
#94388=CARTESIAN_POINT('',(107.978872823157,20.5130996667515,31.));
#94389=CARTESIAN_POINT('Ctrl Pts',(106.921399971368,21.2821063151137,31.));
#94390=CARTESIAN_POINT('Ctrl Pts',(106.921399971368,21.2821063151137,26.));
#94391=CARTESIAN_POINT('Ctrl Pts',(106.928493535689,21.2803874938831,31.));
#94392=CARTESIAN_POINT('Ctrl Pts',(106.928493535689,21.2803874938831,26.));
#94393=CARTESIAN_POINT('Ctrl Pts',(106.942617866551,21.2769154392463,31.));
#94394=CARTESIAN_POINT('Ctrl Pts',(106.942617866551,21.2769154392463,26.));
#94395=CARTESIAN_POINT('Ctrl Pts',(106.963615969762,21.2716041208528,31.));
#94396=CARTESIAN_POINT('Ctrl Pts',(106.963615969762,21.2716041208528,26.));
#94397=CARTESIAN_POINT('Ctrl Pts',(106.991235970075,21.2643155154947,31.));
#94398=CARTESIAN_POINT('Ctrl Pts',(106.991235970075,21.2643155154947,26.));
#94399=CARTESIAN_POINT('Ctrl Pts',(107.025127490565,21.2548581702248,31.));
#94400=CARTESIAN_POINT('Ctrl Pts',(107.025127490565,21.2548581702248,26.));
#94401=CARTESIAN_POINT('Ctrl Pts',(107.05837932368,21.2450524894041,31.));
#94402=CARTESIAN_POINT('Ctrl Pts',(107.05837932368,21.2450524894041,26.));
#94403=CARTESIAN_POINT('Ctrl Pts',(107.09098439885,21.2348979013219,31.));
#94404=CARTESIAN_POINT('Ctrl Pts',(107.09098439885,21.2348979013219,26.));
#94405=CARTESIAN_POINT('Ctrl Pts',(107.122935662486,21.2243960975415,31.));
#94406=CARTESIAN_POINT('Ctrl Pts',(107.122935662486,21.2243960975415,26.));
#94407=CARTESIAN_POINT('Ctrl Pts',(107.154227550431,21.2135523179983,31.));
#94408=CARTESIAN_POINT('Ctrl Pts',(107.154227550431,21.2135523179983,26.));
#94409=CARTESIAN_POINT('Ctrl Pts',(107.184854645532,21.2023758654395,31.));
#94410=CARTESIAN_POINT('Ctrl Pts',(107.184854645532,21.2023758654395,26.));
#94411=CARTESIAN_POINT('Ctrl Pts',(107.214809663899,21.1908803622914,31.));
#94412=CARTESIAN_POINT('Ctrl Pts',(107.214809663899,21.1908803622914,26.));
#94413=CARTESIAN_POINT('Ctrl Pts',(107.244081627808,21.1790843382305,31.));
#94414=CARTESIAN_POINT('Ctrl Pts',(107.244081627808,21.1790843382305,26.));
#94415=CARTESIAN_POINT('Ctrl Pts',(107.27265445322,21.1670114619914,31.));
#94416=CARTESIAN_POINT('Ctrl Pts',(107.27265445322,21.1670114619914,26.));
#94417=CARTESIAN_POINT('Ctrl Pts',(107.300504551943,21.1546918395446,31.));
#94418=CARTESIAN_POINT('Ctrl Pts',(107.300504551943,21.1546918395446,26.));
#94419=CARTESIAN_POINT('Ctrl Pts',(107.327603123085,21.1421593243297,31.));
#94420=CARTESIAN_POINT('Ctrl Pts',(107.327603123085,21.1421593243297,26.));
#94421=CARTESIAN_POINT('Ctrl Pts',(107.353921212311,21.1294465860113,31.));
#94422=CARTESIAN_POINT('Ctrl Pts',(107.353921212311,21.1294465860113,26.));
#94423=CARTESIAN_POINT('Ctrl Pts',(107.379434581049,21.1165804017645,31.));
#94424=CARTESIAN_POINT('Ctrl Pts',(107.379434581049,21.1165804017645,26.));
#94425=CARTESIAN_POINT('Ctrl Pts',(107.404127740668,21.1035779524142,31.));
#94426=CARTESIAN_POINT('Ctrl Pts',(107.404127740668,21.1035779524142,26.));
#94427=CARTESIAN_POINT('Ctrl Pts',(107.428001300286,21.0904399793871,31.));
#94428=CARTESIAN_POINT('Ctrl Pts',(107.428001300286,21.0904399793871,26.));
#94429=CARTESIAN_POINT('Ctrl Pts',(107.451067109266,21.0771560949453,31.));
#94430=CARTESIAN_POINT('Ctrl Pts',(107.451067109266,21.0771560949453,26.));
#94431=CARTESIAN_POINT('Ctrl Pts',(107.473333124035,21.0637202906639,31.));
#94432=CARTESIAN_POINT('Ctrl Pts',(107.473333124035,21.0637202906639,26.));
#94433=CARTESIAN_POINT('Ctrl Pts',(107.49479042636,21.0501445654779,31.));
#94434=CARTESIAN_POINT('Ctrl Pts',(107.49479042636,21.0501445654779,26.));
#94435=CARTESIAN_POINT('Ctrl Pts',(107.515401372613,21.0364714002482,31.));
#94436=CARTESIAN_POINT('Ctrl Pts',(107.515401372613,21.0364714002482,26.));
#94437=CARTESIAN_POINT('Ctrl Pts',(107.535082466814,21.0227920500422,31.));
#94438=CARTESIAN_POINT('Ctrl Pts',(107.535082466814,21.0227920500422,26.));
#94439=CARTESIAN_POINT('Ctrl Pts',(107.553709421352,21.0092413310722,31.));
#94440=CARTESIAN_POINT('Ctrl Pts',(107.553709421352,21.0092413310722,26.));
#94441=CARTESIAN_POINT('Ctrl Pts',(107.571140046246,20.9959735258449,31.));
#94442=CARTESIAN_POINT('Ctrl Pts',(107.571140046246,20.9959735258449,26.));
#94443=CARTESIAN_POINT('Ctrl Pts',(107.58723291893,20.9831430242758,31.));
#94444=CARTESIAN_POINT('Ctrl Pts',(107.58723291893,20.9831430242758,26.));
#94445=CARTESIAN_POINT('Ctrl Pts',(107.601866156854,20.9708848153193,31.));
#94446=CARTESIAN_POINT('Ctrl Pts',(107.601866156854,20.9708848153193,26.));
#94447=CARTESIAN_POINT('Ctrl Pts',(107.614961199771,20.9592902980868,31.));
#94448=CARTESIAN_POINT('Ctrl Pts',(107.614961199771,20.9592902980868,26.));
#94449=CARTESIAN_POINT('Ctrl Pts',(107.626479908354,20.9484092543561,31.));
#94450=CARTESIAN_POINT('Ctrl Pts',(107.626479908354,20.9484092543561,26.));
#94451=CARTESIAN_POINT('Ctrl Pts',(107.634423517433,20.9402929843288,31.));
#94452=CARTESIAN_POINT('Ctrl Pts',(107.634423517433,20.9402929843288,26.));
#94453=CARTESIAN_POINT('Ctrl Pts',(107.639666871604,20.9345388664318,31.));
#94454=CARTESIAN_POINT('Ctrl Pts',(107.639666871604,20.9345388664318,26.));
#94455=CARTESIAN_POINT('Ctrl Pts',(107.642845514348,20.9308505683922,31.));
#94456=CARTESIAN_POINT('Ctrl Pts',(107.642845514348,20.9308505683922,26.));
#94457=CARTESIAN_POINT('Ctrl Pts',(107.644355604652,20.9290433639019,31.));
#94458=CARTESIAN_POINT('Ctrl Pts',(107.644355604652,20.9290433639019,26.));
#94459=CARTESIAN_POINT('',(106.921399971368,21.2821063151137,31.));
#94460=CARTESIAN_POINT('Ctrl Pts',(107.644355604652,20.9290433639019,31.));
#94461=CARTESIAN_POINT('Ctrl Pts',(107.642845514348,20.9308505683922,31.));
#94462=CARTESIAN_POINT('Ctrl Pts',(107.639666871604,20.9345388664318,31.));
#94463=CARTESIAN_POINT('Ctrl Pts',(107.634423517433,20.9402929843288,31.));
#94464=CARTESIAN_POINT('Ctrl Pts',(107.626479908354,20.9484092543561,31.));
#94465=CARTESIAN_POINT('Ctrl Pts',(107.614961199771,20.9592902980868,31.));
#94466=CARTESIAN_POINT('Ctrl Pts',(107.601866156854,20.9708848153193,31.));
#94467=CARTESIAN_POINT('Ctrl Pts',(107.58723291893,20.9831430242758,31.));
#94468=CARTESIAN_POINT('Ctrl Pts',(107.571140046246,20.9959735258449,31.));
#94469=CARTESIAN_POINT('Ctrl Pts',(107.553709421352,21.0092413310722,31.));
#94470=CARTESIAN_POINT('Ctrl Pts',(107.535082466814,21.0227920500422,31.));
#94471=CARTESIAN_POINT('Ctrl Pts',(107.515401372613,21.0364714002482,31.));
#94472=CARTESIAN_POINT('Ctrl Pts',(107.49479042636,21.0501445654779,31.));
#94473=CARTESIAN_POINT('Ctrl Pts',(107.473333124035,21.0637202906639,31.));
#94474=CARTESIAN_POINT('Ctrl Pts',(107.451067109266,21.0771560949453,31.));
#94475=CARTESIAN_POINT('Ctrl Pts',(107.428001300286,21.0904399793871,31.));
#94476=CARTESIAN_POINT('Ctrl Pts',(107.404127740668,21.1035779524142,31.));
#94477=CARTESIAN_POINT('Ctrl Pts',(107.379434581049,21.1165804017645,31.));
#94478=CARTESIAN_POINT('Ctrl Pts',(107.353921212311,21.1294465860113,31.));
#94479=CARTESIAN_POINT('Ctrl Pts',(107.327603123085,21.1421593243297,31.));
#94480=CARTESIAN_POINT('Ctrl Pts',(107.300504551943,21.1546918395446,31.));
#94481=CARTESIAN_POINT('Ctrl Pts',(107.27265445322,21.1670114619914,31.));
#94482=CARTESIAN_POINT('Ctrl Pts',(107.244081627808,21.1790843382305,31.));
#94483=CARTESIAN_POINT('Ctrl Pts',(107.214809663899,21.1908803622914,31.));
#94484=CARTESIAN_POINT('Ctrl Pts',(107.184854645532,21.2023758654395,31.));
#94485=CARTESIAN_POINT('Ctrl Pts',(107.154227550431,21.2135523179983,31.));
#94486=CARTESIAN_POINT('Ctrl Pts',(107.122935662486,21.2243960975415,31.));
#94487=CARTESIAN_POINT('Ctrl Pts',(107.09098439885,21.2348979013219,31.));
#94488=CARTESIAN_POINT('Ctrl Pts',(107.05837932368,21.2450524894041,31.));
#94489=CARTESIAN_POINT('Ctrl Pts',(107.025127490565,21.2548581702248,31.));
#94490=CARTESIAN_POINT('Ctrl Pts',(106.991235970075,21.2643155154947,31.));
#94491=CARTESIAN_POINT('Ctrl Pts',(106.963615969762,21.2716041208528,31.));
#94492=CARTESIAN_POINT('Ctrl Pts',(106.942617866551,21.2769154392463,31.));
#94493=CARTESIAN_POINT('Ctrl Pts',(106.928493535689,21.2803874938831,31.));
#94494=CARTESIAN_POINT('Ctrl Pts',(106.921399971368,21.2821063151137,31.));
#94495=CARTESIAN_POINT('',(106.921399971368,21.2821063151137,26.));
#94496=CARTESIAN_POINT('Ctrl Pts',(106.921399971368,21.2821063151137,26.));
#94497=CARTESIAN_POINT('Ctrl Pts',(106.928493535689,21.2803874938831,26.));
#94498=CARTESIAN_POINT('Ctrl Pts',(106.942617866551,21.2769154392463,26.));
#94499=CARTESIAN_POINT('Ctrl Pts',(106.963615969762,21.2716041208528,26.));
#94500=CARTESIAN_POINT('Ctrl Pts',(106.991235970075,21.2643155154947,26.));
#94501=CARTESIAN_POINT('Ctrl Pts',(107.025127490565,21.2548581702248,26.));
#94502=CARTESIAN_POINT('Ctrl Pts',(107.05837932368,21.2450524894041,26.));
#94503=CARTESIAN_POINT('Ctrl Pts',(107.09098439885,21.2348979013219,26.));
#94504=CARTESIAN_POINT('Ctrl Pts',(107.122935662486,21.2243960975415,26.));
#94505=CARTESIAN_POINT('Ctrl Pts',(107.154227550431,21.2135523179983,26.));
#94506=CARTESIAN_POINT('Ctrl Pts',(107.184854645532,21.2023758654395,26.));
#94507=CARTESIAN_POINT('Ctrl Pts',(107.214809663899,21.1908803622914,26.));
#94508=CARTESIAN_POINT('Ctrl Pts',(107.244081627808,21.1790843382305,26.));
#94509=CARTESIAN_POINT('Ctrl Pts',(107.27265445322,21.1670114619914,26.));
#94510=CARTESIAN_POINT('Ctrl Pts',(107.300504551943,21.1546918395446,26.));
#94511=CARTESIAN_POINT('Ctrl Pts',(107.327603123085,21.1421593243297,26.));
#94512=CARTESIAN_POINT('Ctrl Pts',(107.353921212311,21.1294465860113,26.));
#94513=CARTESIAN_POINT('Ctrl Pts',(107.379434581049,21.1165804017645,26.));
#94514=CARTESIAN_POINT('Ctrl Pts',(107.404127740668,21.1035779524142,26.));
#94515=CARTESIAN_POINT('Ctrl Pts',(107.428001300286,21.0904399793871,26.));
#94516=CARTESIAN_POINT('Ctrl Pts',(107.451067109266,21.0771560949453,26.));
#94517=CARTESIAN_POINT('Ctrl Pts',(107.473333124035,21.0637202906639,26.));
#94518=CARTESIAN_POINT('Ctrl Pts',(107.49479042636,21.0501445654779,26.));
#94519=CARTESIAN_POINT('Ctrl Pts',(107.515401372613,21.0364714002482,26.));
#94520=CARTESIAN_POINT('Ctrl Pts',(107.535082466814,21.0227920500422,26.));
#94521=CARTESIAN_POINT('Ctrl Pts',(107.553709421352,21.0092413310722,26.));
#94522=CARTESIAN_POINT('Ctrl Pts',(107.571140046246,20.9959735258449,26.));
#94523=CARTESIAN_POINT('Ctrl Pts',(107.58723291893,20.9831430242758,26.));
#94524=CARTESIAN_POINT('Ctrl Pts',(107.601866156854,20.9708848153193,26.));
#94525=CARTESIAN_POINT('Ctrl Pts',(107.614961199771,20.9592902980868,26.));
#94526=CARTESIAN_POINT('Ctrl Pts',(107.626479908354,20.9484092543561,26.));
#94527=CARTESIAN_POINT('Ctrl Pts',(107.634423517433,20.9402929843288,26.));
#94528=CARTESIAN_POINT('Ctrl Pts',(107.639666871604,20.9345388664318,26.));
#94529=CARTESIAN_POINT('Ctrl Pts',(107.642845514348,20.9308505683922,26.));
#94530=CARTESIAN_POINT('Ctrl Pts',(107.644355604652,20.9290433639019,26.));
#94531=CARTESIAN_POINT('',(106.921399971368,21.2821063151137,31.));
#94532=CARTESIAN_POINT('Origin',(110.000000000002,17.9999999999979,31.));
#94533=CARTESIAN_POINT('',(106.717893684886,21.0786000286317,31.));
#94534=CARTESIAN_POINT('Origin',(110.000000000002,17.9999999999979,31.));
#94535=CARTESIAN_POINT('',(106.717893684886,21.0786000286317,26.));
#94536=CARTESIAN_POINT('Origin',(110.000000000002,17.9999999999979,26.));
#94537=CARTESIAN_POINT('',(106.717893684886,21.0786000286317,31.));
#94538=CARTESIAN_POINT('Ctrl Pts',(107.070956636098,20.3556443953479,31.));
#94539=CARTESIAN_POINT('Ctrl Pts',(107.070956636098,20.3556443953479,26.));
#94540=CARTESIAN_POINT('Ctrl Pts',(107.069149431603,20.3571544856476,31.));
#94541=CARTESIAN_POINT('Ctrl Pts',(107.069149431603,20.3571544856476,26.));
#94542=CARTESIAN_POINT('Ctrl Pts',(107.065461133556,20.3603331283848,31.));
#94543=CARTESIAN_POINT('Ctrl Pts',(107.065461133556,20.3603331283848,26.));
#94544=CARTESIAN_POINT('Ctrl Pts',(107.059707015651,20.3655764825486,31.));
#94545=CARTESIAN_POINT('Ctrl Pts',(107.059707015651,20.3655764825486,26.));
#94546=CARTESIAN_POINT('Ctrl Pts',(107.05159074562,20.3735200916247,31.));
#94547=CARTESIAN_POINT('Ctrl Pts',(107.05159074562,20.3735200916247,26.));
#94548=CARTESIAN_POINT('Ctrl Pts',(107.040709701894,20.3850388002116,31.));
#94549=CARTESIAN_POINT('Ctrl Pts',(107.040709701894,20.3850388002116,26.));
#94550=CARTESIAN_POINT('Ctrl Pts',(107.029115184672,20.3981338431379,31.));
#94551=CARTESIAN_POINT('Ctrl Pts',(107.029115184672,20.3981338431379,26.));
#94552=CARTESIAN_POINT('Ctrl Pts',(107.016856975728,20.4127670810742,31.));
#94553=CARTESIAN_POINT('Ctrl Pts',(107.016856975728,20.4127670810742,26.));
#94554=CARTESIAN_POINT('Ctrl Pts',(107.004026474169,20.4288599537678,31.));
#94555=CARTESIAN_POINT('Ctrl Pts',(107.004026474169,20.4288599537678,26.));
#94556=CARTESIAN_POINT('Ctrl Pts',(106.990758668946,20.4462905786649,31.));
#94557=CARTESIAN_POINT('Ctrl Pts',(106.990758668946,20.4462905786649,26.));
#94558=CARTESIAN_POINT('Ctrl Pts',(106.977207949972,20.4649175332003,31.));
#94559=CARTESIAN_POINT('Ctrl Pts',(106.977207949972,20.4649175332003,26.));
#94560=CARTESIAN_POINT('Ctrl Pts',(106.963528599757,20.4845986273924,31.));
#94561=CARTESIAN_POINT('Ctrl Pts',(106.963528599757,20.4845986273924,26.));
#94562=CARTESIAN_POINT('Ctrl Pts',(106.949855434517,20.5052095736352,31.));
#94563=CARTESIAN_POINT('Ctrl Pts',(106.949855434517,20.5052095736352,26.));
#94564=CARTESIAN_POINT('Ctrl Pts',(106.936279709323,20.5266668759518,31.));
#94565=CARTESIAN_POINT('Ctrl Pts',(106.936279709323,20.5266668759518,26.));
#94566=CARTESIAN_POINT('Ctrl Pts',(106.922843905036,20.5489328907163,31.));
#94567=CARTESIAN_POINT('Ctrl Pts',(106.922843905036,20.5489328907163,26.));
#94568=CARTESIAN_POINT('Ctrl Pts',(106.909560020596,20.5719986996976,31.));
#94569=CARTESIAN_POINT('Ctrl Pts',(106.909560020596,20.5719986996976,26.));
#94570=CARTESIAN_POINT('Ctrl Pts',(106.896422047578,20.5958722593236,31.));
#94571=CARTESIAN_POINT('Ctrl Pts',(106.896422047578,20.5958722593236,26.));
#94572=CARTESIAN_POINT('Ctrl Pts',(106.883419598242,20.6205654189573,31.));
#94573=CARTESIAN_POINT('Ctrl Pts',(106.883419598242,20.6205654189573,26.));
#94574=CARTESIAN_POINT('Ctrl Pts',(106.87055341401,20.6460787877111,31.));
#94575=CARTESIAN_POINT('Ctrl Pts',(106.87055341401,20.6460787877111,26.));
#94576=CARTESIAN_POINT('Ctrl Pts',(106.857840675702,20.6723968769464,31.));
#94577=CARTESIAN_POINT('Ctrl Pts',(106.857840675702,20.6723968769464,26.));
#94578=CARTESIAN_POINT('Ctrl Pts',(106.845308160487,20.6994954480886,31.));
#94579=CARTESIAN_POINT('Ctrl Pts',(106.845308160487,20.6994954480886,26.));
#94580=CARTESIAN_POINT('Ctrl Pts',(106.832988538026,20.7273455467972,31.));
#94581=CARTESIAN_POINT('Ctrl Pts',(106.832988538026,20.7273455467972,26.));
#94582=CARTESIAN_POINT('Ctrl Pts',(106.82091566176,20.7559183721823,31.));
#94583=CARTESIAN_POINT('Ctrl Pts',(106.82091566176,20.7559183721823,26.));
#94584=CARTESIAN_POINT('Ctrl Pts',(106.809119637666,20.7851903360588,31.));
#94585=CARTESIAN_POINT('Ctrl Pts',(106.809119637666,20.7851903360588,26.));
#94586=CARTESIAN_POINT('Ctrl Pts',(106.797624134493,20.8151453544004,31.));
#94587=CARTESIAN_POINT('Ctrl Pts',(106.797624134493,20.8151453544004,26.));
#94588=CARTESIAN_POINT('Ctrl Pts',(106.786447681929,20.8457724494961,31.));
#94589=CARTESIAN_POINT('Ctrl Pts',(106.786447681929,20.8457724494961,26.));
#94590=CARTESIAN_POINT('Ctrl Pts',(106.775603902411,20.8770643374659,31.));
#94591=CARTESIAN_POINT('Ctrl Pts',(106.775603902411,20.8770643374659,26.));
#94592=CARTESIAN_POINT('Ctrl Pts',(106.765102098688,20.9090156011607,31.));
#94593=CARTESIAN_POINT('Ctrl Pts',(106.765102098688,20.9090156011607,26.));
#94594=CARTESIAN_POINT('Ctrl Pts',(106.754947510685,20.9416206764099,31.));
#94595=CARTESIAN_POINT('Ctrl Pts',(106.754947510685,20.9416206764099,26.));
#94596=CARTESIAN_POINT('Ctrl Pts',(106.745141829939,20.9748725095998,31.));
#94597=CARTESIAN_POINT('Ctrl Pts',(106.745141829939,20.9748725095998,26.));
#94598=CARTESIAN_POINT('Ctrl Pts',(106.735684484705,21.0087640301252,31.));
#94599=CARTESIAN_POINT('Ctrl Pts',(106.735684484705,21.0087640301252,26.));
#94600=CARTESIAN_POINT('Ctrl Pts',(106.728395879318,21.0363840304093,31.));
#94601=CARTESIAN_POINT('Ctrl Pts',(106.728395879318,21.0363840304093,26.));
#94602=CARTESIAN_POINT('Ctrl Pts',(106.723084560858,21.057382133554,31.));
#94603=CARTESIAN_POINT('Ctrl Pts',(106.723084560858,21.057382133554,26.));
#94604=CARTESIAN_POINT('Ctrl Pts',(106.719612506155,21.0715064643493,31.));
#94605=CARTESIAN_POINT('Ctrl Pts',(106.719612506155,21.0715064643493,26.));
#94606=CARTESIAN_POINT('Ctrl Pts',(106.717893684886,21.0786000286317,31.));
#94607=CARTESIAN_POINT('Ctrl Pts',(106.717893684886,21.0786000286317,26.));
#94608=CARTESIAN_POINT('Ctrl Pts',(107.070956636098,20.3556443953479,31.));
#94609=CARTESIAN_POINT('Ctrl Pts',(107.069149431603,20.3571544856476,31.));
#94610=CARTESIAN_POINT('Ctrl Pts',(107.065461133556,20.3603331283848,31.));
#94611=CARTESIAN_POINT('Ctrl Pts',(107.059707015651,20.3655764825486,31.));
#94612=CARTESIAN_POINT('Ctrl Pts',(107.05159074562,20.3735200916247,31.));
#94613=CARTESIAN_POINT('Ctrl Pts',(107.040709701894,20.3850388002116,31.));
#94614=CARTESIAN_POINT('Ctrl Pts',(107.029115184672,20.3981338431379,31.));
#94615=CARTESIAN_POINT('Ctrl Pts',(107.016856975728,20.4127670810742,31.));
#94616=CARTESIAN_POINT('Ctrl Pts',(107.004026474169,20.4288599537678,31.));
#94617=CARTESIAN_POINT('Ctrl Pts',(106.990758668946,20.4462905786649,31.));
#94618=CARTESIAN_POINT('Ctrl Pts',(106.977207949972,20.4649175332003,31.));
#94619=CARTESIAN_POINT('Ctrl Pts',(106.963528599757,20.4845986273924,31.));
#94620=CARTESIAN_POINT('Ctrl Pts',(106.949855434517,20.5052095736352,31.));
#94621=CARTESIAN_POINT('Ctrl Pts',(106.936279709323,20.5266668759518,31.));
#94622=CARTESIAN_POINT('Ctrl Pts',(106.922843905036,20.5489328907163,31.));
#94623=CARTESIAN_POINT('Ctrl Pts',(106.909560020596,20.5719986996976,31.));
#94624=CARTESIAN_POINT('Ctrl Pts',(106.896422047578,20.5958722593236,31.));
#94625=CARTESIAN_POINT('Ctrl Pts',(106.883419598242,20.6205654189573,31.));
#94626=CARTESIAN_POINT('Ctrl Pts',(106.87055341401,20.6460787877111,31.));
#94627=CARTESIAN_POINT('Ctrl Pts',(106.857840675702,20.6723968769464,31.));
#94628=CARTESIAN_POINT('Ctrl Pts',(106.845308160487,20.6994954480886,31.));
#94629=CARTESIAN_POINT('Ctrl Pts',(106.832988538026,20.7273455467972,31.));
#94630=CARTESIAN_POINT('Ctrl Pts',(106.82091566176,20.7559183721823,31.));
#94631=CARTESIAN_POINT('Ctrl Pts',(106.809119637666,20.7851903360588,31.));
#94632=CARTESIAN_POINT('Ctrl Pts',(106.797624134493,20.8151453544004,31.));
#94633=CARTESIAN_POINT('Ctrl Pts',(106.786447681929,20.8457724494961,31.));
#94634=CARTESIAN_POINT('Ctrl Pts',(106.775603902411,20.8770643374659,31.));
#94635=CARTESIAN_POINT('Ctrl Pts',(106.765102098688,20.9090156011607,31.));
#94636=CARTESIAN_POINT('Ctrl Pts',(106.754947510685,20.9416206764099,31.));
#94637=CARTESIAN_POINT('Ctrl Pts',(106.745141829939,20.9748725095998,31.));
#94638=CARTESIAN_POINT('Ctrl Pts',(106.735684484705,21.0087640301252,31.));
#94639=CARTESIAN_POINT('Ctrl Pts',(106.728395879318,21.0363840304093,31.));
#94640=CARTESIAN_POINT('Ctrl Pts',(106.723084560858,21.057382133554,31.));
#94641=CARTESIAN_POINT('Ctrl Pts',(106.719612506155,21.0715064643493,31.));
#94642=CARTESIAN_POINT('Ctrl Pts',(106.717893684886,21.0786000286317,31.));
#94643=CARTESIAN_POINT('Ctrl Pts',(107.070956636098,20.3556443953479,26.));
#94644=CARTESIAN_POINT('Ctrl Pts',(107.069149431603,20.3571544856476,26.));
#94645=CARTESIAN_POINT('Ctrl Pts',(107.065461133556,20.3603331283848,26.));
#94646=CARTESIAN_POINT('Ctrl Pts',(107.059707015651,20.3655764825486,26.));
#94647=CARTESIAN_POINT('Ctrl Pts',(107.05159074562,20.3735200916247,26.));
#94648=CARTESIAN_POINT('Ctrl Pts',(107.040709701894,20.3850388002116,26.));
#94649=CARTESIAN_POINT('Ctrl Pts',(107.029115184672,20.3981338431379,26.));
#94650=CARTESIAN_POINT('Ctrl Pts',(107.016856975728,20.4127670810742,26.));
#94651=CARTESIAN_POINT('Ctrl Pts',(107.004026474169,20.4288599537678,26.));
#94652=CARTESIAN_POINT('Ctrl Pts',(106.990758668946,20.4462905786649,26.));
#94653=CARTESIAN_POINT('Ctrl Pts',(106.977207949972,20.4649175332003,26.));
#94654=CARTESIAN_POINT('Ctrl Pts',(106.963528599757,20.4845986273924,26.));
#94655=CARTESIAN_POINT('Ctrl Pts',(106.949855434517,20.5052095736352,26.));
#94656=CARTESIAN_POINT('Ctrl Pts',(106.936279709323,20.5266668759518,26.));
#94657=CARTESIAN_POINT('Ctrl Pts',(106.922843905036,20.5489328907163,26.));
#94658=CARTESIAN_POINT('Ctrl Pts',(106.909560020596,20.5719986996976,26.));
#94659=CARTESIAN_POINT('Ctrl Pts',(106.896422047578,20.5958722593236,26.));
#94660=CARTESIAN_POINT('Ctrl Pts',(106.883419598242,20.6205654189573,26.));
#94661=CARTESIAN_POINT('Ctrl Pts',(106.87055341401,20.6460787877111,26.));
#94662=CARTESIAN_POINT('Ctrl Pts',(106.857840675702,20.6723968769464,26.));
#94663=CARTESIAN_POINT('Ctrl Pts',(106.845308160487,20.6994954480886,26.));
#94664=CARTESIAN_POINT('Ctrl Pts',(106.832988538026,20.7273455467972,26.));
#94665=CARTESIAN_POINT('Ctrl Pts',(106.82091566176,20.7559183721823,26.));
#94666=CARTESIAN_POINT('Ctrl Pts',(106.809119637666,20.7851903360588,26.));
#94667=CARTESIAN_POINT('Ctrl Pts',(106.797624134493,20.8151453544004,26.));
#94668=CARTESIAN_POINT('Ctrl Pts',(106.786447681929,20.8457724494961,26.));
#94669=CARTESIAN_POINT('Ctrl Pts',(106.775603902411,20.8770643374659,26.));
#94670=CARTESIAN_POINT('Ctrl Pts',(106.765102098688,20.9090156011607,26.));
#94671=CARTESIAN_POINT('Ctrl Pts',(106.754947510685,20.9416206764099,26.));
#94672=CARTESIAN_POINT('Ctrl Pts',(106.745141829939,20.9748725095998,26.));
#94673=CARTESIAN_POINT('Ctrl Pts',(106.735684484705,21.0087640301252,26.));
#94674=CARTESIAN_POINT('Ctrl Pts',(106.728395879318,21.0363840304093,26.));
#94675=CARTESIAN_POINT('Ctrl Pts',(106.723084560858,21.057382133554,26.));
#94676=CARTESIAN_POINT('Ctrl Pts',(106.719612506155,21.0715064643493,26.));
#94677=CARTESIAN_POINT('Ctrl Pts',(106.717893684886,21.0786000286317,26.));
#94678=CARTESIAN_POINT('Origin',(107.27545303142,20.7245469685571,31.));
#94679=CARTESIAN_POINT('Origin',(108.451650540008,20.8289996376356,31.));
#94680=CARTESIAN_POINT('',(108.195382868896,21.297228010781,31.));
#94681=CARTESIAN_POINT('',(108.195382868896,21.297228010781,31.));
#94682=CARTESIAN_POINT('',(108.195382868896,21.297228010781,26.));
#94683=CARTESIAN_POINT('',(108.195382868896,21.297228010781,31.));
#94684=CARTESIAN_POINT('',(108.195382868896,21.297228010781,26.));
#94685=CARTESIAN_POINT('Origin',(108.944564725307,21.6075492963903,31.));
#94686=CARTESIAN_POINT('',(108.944564725307,21.6075492963903,26.));
#94687=CARTESIAN_POINT('',(109.09444357506,21.0952532305533,26.));
#94688=CARTESIAN_POINT('',(108.944564725307,21.6075492963903,31.));
#94689=CARTESIAN_POINT('',(108.944564725307,21.6075492963903,31.));
#94690=CARTESIAN_POINT('',(109.09444357506,21.0952532305533,31.));
#94691=CARTESIAN_POINT('Ctrl Pts',(108.411752154813,22.2104000738956,31.));
#94692=CARTESIAN_POINT('Ctrl Pts',(108.411752154813,22.2104000738956,26.));
#94693=CARTESIAN_POINT('Ctrl Pts',(108.417647989294,22.2060975005986,31.));
#94694=CARTESIAN_POINT('Ctrl Pts',(108.417647989294,22.2060975005986,26.));
#94695=CARTESIAN_POINT('Ctrl Pts',(108.429368471701,22.19748459297,31.));
#94696=CARTESIAN_POINT('Ctrl Pts',(108.429368471701,22.19748459297,26.));
#94697=CARTESIAN_POINT('Ctrl Pts',(108.446735635927,22.1845419484054,31.));
#94698=CARTESIAN_POINT('Ctrl Pts',(108.446735635927,22.1845419484054,26.));
#94699=CARTESIAN_POINT('Ctrl Pts',(108.469463960389,22.1672384385728,31.));
#94700=CARTESIAN_POINT('Ctrl Pts',(108.469463960389,22.1672384385728,26.));
#94701=CARTESIAN_POINT('Ctrl Pts',(108.497156473145,22.1455312674571,31.));
#94702=CARTESIAN_POINT('Ctrl Pts',(108.497156473145,22.1455312674571,26.));
#94703=CARTESIAN_POINT('Ctrl Pts',(108.524124689586,22.1237470740155,31.));
#94704=CARTESIAN_POINT('Ctrl Pts',(108.524124689586,22.1237470740155,26.));
#94705=CARTESIAN_POINT('Ctrl Pts',(108.55036185857,22.1018880358469,31.));
#94706=CARTESIAN_POINT('Ctrl Pts',(108.55036185857,22.1018880358469,26.));
#94707=CARTESIAN_POINT('Ctrl Pts',(108.575862110765,22.0799584150428,31.));
#94708=CARTESIAN_POINT('Ctrl Pts',(108.575862110765,22.0799584150428,26.));
#94709=CARTESIAN_POINT('Ctrl Pts',(108.600622310795,22.0579651819841,31.));
#94710=CARTESIAN_POINT('Ctrl Pts',(108.600622310795,22.0579651819841,26.));
#94711=CARTESIAN_POINT('Ctrl Pts',(108.624641013872,22.0359190043423,31.));
#94712=CARTESIAN_POINT('Ctrl Pts',(108.624641013872,22.0359190043423,26.));
#94713=CARTESIAN_POINT('Ctrl Pts',(108.647916703636,22.0138352550225,31.));
#94714=CARTESIAN_POINT('Ctrl Pts',(108.647916703636,22.0138352550225,26.));
#94715=CARTESIAN_POINT('Ctrl Pts',(108.670446328992,21.9917352542068,31.));
#94716=CARTESIAN_POINT('Ctrl Pts',(108.670446328992,21.9917352542068,26.));
#94717=CARTESIAN_POINT('Ctrl Pts',(108.692224087859,21.9696470240499,31.));
#94718=CARTESIAN_POINT('Ctrl Pts',(108.692224087859,21.9696470240499,26.));
#94719=CARTESIAN_POINT('Ctrl Pts',(108.713239708644,21.947607405652,31.));
#94720=CARTESIAN_POINT('Ctrl Pts',(108.713239708644,21.947607405652,26.));
#94721=CARTESIAN_POINT('Ctrl Pts',(108.733479537944,21.9256586971371,31.));
#94722=CARTESIAN_POINT('Ctrl Pts',(108.733479537944,21.9256586971371,26.));
#94723=CARTESIAN_POINT('Ctrl Pts',(108.75292932758,21.9038421616846,31.));
#94724=CARTESIAN_POINT('Ctrl Pts',(108.75292932758,21.9038421616846,26.));
#94725=CARTESIAN_POINT('Ctrl Pts',(108.771576931213,21.8821918138775,31.));
#94726=CARTESIAN_POINT('Ctrl Pts',(108.771576931213,21.8821918138775,26.));
#94727=CARTESIAN_POINT('Ctrl Pts',(108.789414614032,21.8607294539711,31.));
#94728=CARTESIAN_POINT('Ctrl Pts',(108.789414614032,21.8607294539711,26.));
#94729=CARTESIAN_POINT('Ctrl Pts',(108.806443222519,21.8394555338556,31.));
#94730=CARTESIAN_POINT('Ctrl Pts',(108.806443222519,21.8394555338556,26.));
#94731=CARTESIAN_POINT('Ctrl Pts',(108.822669728842,21.8183559219568,31.));
#94732=CARTESIAN_POINT('Ctrl Pts',(108.822669728842,21.8183559219568,26.));
#94733=CARTESIAN_POINT('Ctrl Pts',(108.838099184459,21.7974220224214,31.));
#94734=CARTESIAN_POINT('Ctrl Pts',(108.838099184459,21.7974220224214,26.));
#94735=CARTESIAN_POINT('Ctrl Pts',(108.85272794179,21.7766683336798,31.));
#94736=CARTESIAN_POINT('Ctrl Pts',(108.85272794179,21.7766683336798,26.));
#94737=CARTESIAN_POINT('Ctrl Pts',(108.866537479377,21.7561485085232,31.));
#94738=CARTESIAN_POINT('Ctrl Pts',(108.866537479377,21.7561485085232,26.));
#94739=CARTESIAN_POINT('Ctrl Pts',(108.879485578797,21.7359788081685,31.));
#94740=CARTESIAN_POINT('Ctrl Pts',(108.879485578797,21.7359788081685,26.));
#94741=CARTESIAN_POINT('Ctrl Pts',(108.891509005202,21.7163313493639,31.));
#94742=CARTESIAN_POINT('Ctrl Pts',(108.891509005202,21.7163313493639,26.));
#94743=CARTESIAN_POINT('Ctrl Pts',(108.902535433535,21.6974030843105,31.));
#94744=CARTESIAN_POINT('Ctrl Pts',(108.902535433535,21.6974030843105,26.));
#94745=CARTESIAN_POINT('Ctrl Pts',(108.912493288848,21.6793907707637,31.));
#94746=CARTESIAN_POINT('Ctrl Pts',(108.912493288848,21.6793907707637,26.));
#94747=CARTESIAN_POINT('Ctrl Pts',(108.921321624383,21.6624657646879,31.));
#94748=CARTESIAN_POINT('Ctrl Pts',(108.921321624383,21.6624657646879,26.));
#94749=CARTESIAN_POINT('Ctrl Pts',(108.92898283686,21.6467425715572,31.));
#94750=CARTESIAN_POINT('Ctrl Pts',(108.92898283686,21.6467425715572,26.));
#94751=CARTESIAN_POINT('Ctrl Pts',(108.935460740798,21.6322817790252,31.));
#94752=CARTESIAN_POINT('Ctrl Pts',(108.935460740798,21.6322817790252,26.));
#94753=CARTESIAN_POINT('Ctrl Pts',(108.939693716568,21.6217434356788,31.));
#94754=CARTESIAN_POINT('Ctrl Pts',(108.939693716568,21.6217434356788,26.));
#94755=CARTESIAN_POINT('Ctrl Pts',(108.942335938581,21.6144207791549,31.));
#94756=CARTESIAN_POINT('Ctrl Pts',(108.942335938581,21.6144207791549,26.));
#94757=CARTESIAN_POINT('Ctrl Pts',(108.943861171001,21.6097968221706,31.));
#94758=CARTESIAN_POINT('Ctrl Pts',(108.943861171001,21.6097968221706,26.));
#94759=CARTESIAN_POINT('Ctrl Pts',(108.944564725307,21.6075492963903,31.));
#94760=CARTESIAN_POINT('Ctrl Pts',(108.944564725307,21.6075492963903,26.));
#94761=CARTESIAN_POINT('',(108.411752154813,22.2104000738956,31.));
#94762=CARTESIAN_POINT('Ctrl Pts',(108.944564725307,21.6075492963903,31.));
#94763=CARTESIAN_POINT('Ctrl Pts',(108.943861171001,21.6097968221706,31.));
#94764=CARTESIAN_POINT('Ctrl Pts',(108.942335938581,21.6144207791549,31.));
#94765=CARTESIAN_POINT('Ctrl Pts',(108.939693716568,21.6217434356788,31.));
#94766=CARTESIAN_POINT('Ctrl Pts',(108.935460740798,21.6322817790252,31.));
#94767=CARTESIAN_POINT('Ctrl Pts',(108.92898283686,21.6467425715572,31.));
#94768=CARTESIAN_POINT('Ctrl Pts',(108.921321624383,21.6624657646879,31.));
#94769=CARTESIAN_POINT('Ctrl Pts',(108.912493288848,21.6793907707637,31.));
#94770=CARTESIAN_POINT('Ctrl Pts',(108.902535433535,21.6974030843105,31.));
#94771=CARTESIAN_POINT('Ctrl Pts',(108.891509005202,21.7163313493639,31.));
#94772=CARTESIAN_POINT('Ctrl Pts',(108.879485578797,21.7359788081685,31.));
#94773=CARTESIAN_POINT('Ctrl Pts',(108.866537479377,21.7561485085232,31.));
#94774=CARTESIAN_POINT('Ctrl Pts',(108.85272794179,21.7766683336798,31.));
#94775=CARTESIAN_POINT('Ctrl Pts',(108.838099184459,21.7974220224214,31.));
#94776=CARTESIAN_POINT('Ctrl Pts',(108.822669728842,21.8183559219568,31.));
#94777=CARTESIAN_POINT('Ctrl Pts',(108.806443222519,21.8394555338556,31.));
#94778=CARTESIAN_POINT('Ctrl Pts',(108.789414614032,21.8607294539711,31.));
#94779=CARTESIAN_POINT('Ctrl Pts',(108.771576931213,21.8821918138775,31.));
#94780=CARTESIAN_POINT('Ctrl Pts',(108.75292932758,21.9038421616846,31.));
#94781=CARTESIAN_POINT('Ctrl Pts',(108.733479537944,21.9256586971371,31.));
#94782=CARTESIAN_POINT('Ctrl Pts',(108.713239708644,21.947607405652,31.));
#94783=CARTESIAN_POINT('Ctrl Pts',(108.692224087859,21.9696470240499,31.));
#94784=CARTESIAN_POINT('Ctrl Pts',(108.670446328992,21.9917352542068,31.));
#94785=CARTESIAN_POINT('Ctrl Pts',(108.647916703636,22.0138352550225,31.));
#94786=CARTESIAN_POINT('Ctrl Pts',(108.624641013872,22.0359190043423,31.));
#94787=CARTESIAN_POINT('Ctrl Pts',(108.600622310795,22.0579651819841,31.));
#94788=CARTESIAN_POINT('Ctrl Pts',(108.575862110765,22.0799584150428,31.));
#94789=CARTESIAN_POINT('Ctrl Pts',(108.55036185857,22.1018880358469,31.));
#94790=CARTESIAN_POINT('Ctrl Pts',(108.524124689586,22.1237470740155,31.));
#94791=CARTESIAN_POINT('Ctrl Pts',(108.497156473145,22.1455312674571,31.));
#94792=CARTESIAN_POINT('Ctrl Pts',(108.469463960389,22.1672384385728,31.));
#94793=CARTESIAN_POINT('Ctrl Pts',(108.446735635927,22.1845419484054,31.));
#94794=CARTESIAN_POINT('Ctrl Pts',(108.429368471701,22.19748459297,31.));
#94795=CARTESIAN_POINT('Ctrl Pts',(108.417647989294,22.2060975005986,31.));
#94796=CARTESIAN_POINT('Ctrl Pts',(108.411752154813,22.2104000738956,31.));
#94797=CARTESIAN_POINT('',(108.411752154813,22.2104000738956,26.));
#94798=CARTESIAN_POINT('Ctrl Pts',(108.411752154813,22.2104000738956,26.));
#94799=CARTESIAN_POINT('Ctrl Pts',(108.417647989294,22.2060975005986,26.));
#94800=CARTESIAN_POINT('Ctrl Pts',(108.429368471701,22.19748459297,26.));
#94801=CARTESIAN_POINT('Ctrl Pts',(108.446735635927,22.1845419484054,26.));
#94802=CARTESIAN_POINT('Ctrl Pts',(108.469463960389,22.1672384385728,26.));
#94803=CARTESIAN_POINT('Ctrl Pts',(108.497156473145,22.1455312674571,26.));
#94804=CARTESIAN_POINT('Ctrl Pts',(108.524124689586,22.1237470740155,26.));
#94805=CARTESIAN_POINT('Ctrl Pts',(108.55036185857,22.1018880358469,26.));
#94806=CARTESIAN_POINT('Ctrl Pts',(108.575862110765,22.0799584150428,26.));
#94807=CARTESIAN_POINT('Ctrl Pts',(108.600622310795,22.0579651819841,26.));
#94808=CARTESIAN_POINT('Ctrl Pts',(108.624641013872,22.0359190043423,26.));
#94809=CARTESIAN_POINT('Ctrl Pts',(108.647916703636,22.0138352550225,26.));
#94810=CARTESIAN_POINT('Ctrl Pts',(108.670446328992,21.9917352542068,26.));
#94811=CARTESIAN_POINT('Ctrl Pts',(108.692224087859,21.9696470240499,26.));
#94812=CARTESIAN_POINT('Ctrl Pts',(108.713239708644,21.947607405652,26.));
#94813=CARTESIAN_POINT('Ctrl Pts',(108.733479537944,21.9256586971371,26.));
#94814=CARTESIAN_POINT('Ctrl Pts',(108.75292932758,21.9038421616846,26.));
#94815=CARTESIAN_POINT('Ctrl Pts',(108.771576931213,21.8821918138775,26.));
#94816=CARTESIAN_POINT('Ctrl Pts',(108.789414614032,21.8607294539711,26.));
#94817=CARTESIAN_POINT('Ctrl Pts',(108.806443222519,21.8394555338556,26.));
#94818=CARTESIAN_POINT('Ctrl Pts',(108.822669728842,21.8183559219568,26.));
#94819=CARTESIAN_POINT('Ctrl Pts',(108.838099184459,21.7974220224214,26.));
#94820=CARTESIAN_POINT('Ctrl Pts',(108.85272794179,21.7766683336798,26.));
#94821=CARTESIAN_POINT('Ctrl Pts',(108.866537479377,21.7561485085232,26.));
#94822=CARTESIAN_POINT('Ctrl Pts',(108.879485578797,21.7359788081685,26.));
#94823=CARTESIAN_POINT('Ctrl Pts',(108.891509005202,21.7163313493639,26.));
#94824=CARTESIAN_POINT('Ctrl Pts',(108.902535433535,21.6974030843105,26.));
#94825=CARTESIAN_POINT('Ctrl Pts',(108.912493288848,21.6793907707637,26.));
#94826=CARTESIAN_POINT('Ctrl Pts',(108.921321624383,21.6624657646879,26.));
#94827=CARTESIAN_POINT('Ctrl Pts',(108.92898283686,21.6467425715572,26.));
#94828=CARTESIAN_POINT('Ctrl Pts',(108.935460740798,21.6322817790252,26.));
#94829=CARTESIAN_POINT('Ctrl Pts',(108.939693716568,21.6217434356788,26.));
#94830=CARTESIAN_POINT('Ctrl Pts',(108.942335938581,21.6144207791549,26.));
#94831=CARTESIAN_POINT('Ctrl Pts',(108.943861171001,21.6097968221706,26.));
#94832=CARTESIAN_POINT('Ctrl Pts',(108.944564725307,21.6075492963903,26.));
#94833=CARTESIAN_POINT('',(108.411752154813,22.2104000738956,31.));
#94834=CARTESIAN_POINT('Origin',(110.000000000001,17.9999999999972,31.));
#94835=CARTESIAN_POINT('',(108.145858377777,22.1002632652963,31.));
#94836=CARTESIAN_POINT('Origin',(110.000000000001,17.9999999999972,31.));
#94837=CARTESIAN_POINT('',(108.145858377777,22.1002632652963,26.));
#94838=CARTESIAN_POINT('Origin',(110.000000000001,17.9999999999972,26.));
#94839=CARTESIAN_POINT('',(108.145858377777,22.1002632652963,31.));
#94840=CARTESIAN_POINT('Ctrl Pts',(108.195382868896,21.297228010781,31.));
#94841=CARTESIAN_POINT('Ctrl Pts',(108.195382868896,21.297228010781,26.));
#94842=CARTESIAN_POINT('Ctrl Pts',(108.194291116192,21.2993147395202,31.));
#94843=CARTESIAN_POINT('Ctrl Pts',(108.194291116192,21.2993147395202,26.));
#94844=CARTESIAN_POINT('Ctrl Pts',(108.192099987029,21.3036628730427,31.));
#94845=CARTESIAN_POINT('Ctrl Pts',(108.192099987029,21.3036628730427,26.));
#94846=CARTESIAN_POINT('Ctrl Pts',(108.188790420037,21.3107091062263,31.));
#94847=CARTESIAN_POINT('Ctrl Pts',(108.188790420037,21.3107091062263,26.));
#94848=CARTESIAN_POINT('Ctrl Pts',(108.184331851862,21.3211540061394,31.));
#94849=CARTESIAN_POINT('Ctrl Pts',(108.184331851862,21.3211540061394,26.));
#94850=CARTESIAN_POINT('Ctrl Pts',(108.17868709721,21.3359599004046,31.));
#94851=CARTESIAN_POINT('Ctrl Pts',(108.17868709721,21.3359599004046,26.));
#94852=CARTESIAN_POINT('Ctrl Pts',(108.172986416033,21.3524951721887,31.));
#94853=CARTESIAN_POINT('Ctrl Pts',(108.172986416033,21.3524951721887,26.));
#94854=CARTESIAN_POINT('Ctrl Pts',(108.167261205405,21.3707055346857,31.));
#94855=CARTESIAN_POINT('Ctrl Pts',(108.167261205405,21.3707055346857,26.));
#94856=CARTESIAN_POINT('Ctrl Pts',(108.161565843382,21.3904834307621,31.));
#94857=CARTESIAN_POINT('Ctrl Pts',(108.161565843382,21.3904834307621,26.));
#94858=CARTESIAN_POINT('Ctrl Pts',(108.155978401058,21.4116645975863,31.));
#94859=CARTESIAN_POINT('Ctrl Pts',(108.155978401058,21.4116645975863,26.));
#94860=CARTESIAN_POINT('Ctrl Pts',(108.150587396044,21.4340592952825,31.));
#94861=CARTESIAN_POINT('Ctrl Pts',(108.150587396044,21.4340592952825,26.));
#94862=CARTESIAN_POINT('Ctrl Pts',(108.14548095304,21.4574771160767,31.));
#94863=CARTESIAN_POINT('Ctrl Pts',(108.14548095304,21.4574771160767,26.));
#94864=CARTESIAN_POINT('Ctrl Pts',(108.140736063183,21.4817516412614,31.));
#94865=CARTESIAN_POINT('Ctrl Pts',(108.140736063183,21.4817516412614,26.));
#94866=CARTESIAN_POINT('Ctrl Pts',(108.136405082636,21.5067708088092,31.));
#94867=CARTESIAN_POINT('Ctrl Pts',(108.136405082636,21.5067708088092,26.));
#94868=CARTESIAN_POINT('Ctrl Pts',(108.132512853008,21.5324835838215,31.));
#94869=CARTESIAN_POINT('Ctrl Pts',(108.132512853008,21.5324835838215,26.));
#94870=CARTESIAN_POINT('Ctrl Pts',(108.129067047013,21.5588771351329,31.));
#94871=CARTESIAN_POINT('Ctrl Pts',(108.129067047013,21.5588771351329,26.));
#94872=CARTESIAN_POINT('Ctrl Pts',(108.126065158383,21.5859611128485,31.));
#94873=CARTESIAN_POINT('Ctrl Pts',(108.126065158383,21.5859611128485,26.));
#94874=CARTESIAN_POINT('Ctrl Pts',(108.123502124654,21.6137504395681,31.));
#94875=CARTESIAN_POINT('Ctrl Pts',(108.123502124654,21.6137504395681,26.));
#94876=CARTESIAN_POINT('Ctrl Pts',(108.121378863907,21.6422453943083,31.));
#94877=CARTESIAN_POINT('Ctrl Pts',(108.121378863907,21.6422453943083,26.));
#94878=CARTESIAN_POINT('Ctrl Pts',(108.119705321903,21.6714250926182,31.));
#94879=CARTESIAN_POINT('Ctrl Pts',(108.119705321903,21.6714250926182,26.));
#94880=CARTESIAN_POINT('Ctrl Pts',(108.118496961822,21.7012568937955,31.));
#94881=CARTESIAN_POINT('Ctrl Pts',(108.118496961822,21.7012568937955,26.));
#94882=CARTESIAN_POINT('Ctrl Pts',(108.117772886147,21.7317015453796,31.));
#94883=CARTESIAN_POINT('Ctrl Pts',(108.117772886147,21.7317015453796,26.));
#94884=CARTESIAN_POINT('Ctrl Pts',(108.117553349757,21.7627194836669,31.));
#94885=CARTESIAN_POINT('Ctrl Pts',(108.117553349757,21.7627194836669,26.));
#94886=CARTESIAN_POINT('Ctrl Pts',(108.117857140141,21.7942773949572,31.));
#94887=CARTESIAN_POINT('Ctrl Pts',(108.117857140141,21.7942773949572,26.));
#94888=CARTESIAN_POINT('Ctrl Pts',(108.118699969278,21.8263513619102,31.));
#94889=CARTESIAN_POINT('Ctrl Pts',(108.118699969278,21.8263513619102,26.));
#94890=CARTESIAN_POINT('Ctrl Pts',(108.120094755383,21.8589241514383,31.));
#94891=CARTESIAN_POINT('Ctrl Pts',(108.120094755383,21.8589241514383,26.));
#94892=CARTESIAN_POINT('Ctrl Pts',(108.122051296525,21.8919838210329,31.));
#94893=CARTESIAN_POINT('Ctrl Pts',(108.122051296525,21.8919838210329,26.));
#94894=CARTESIAN_POINT('Ctrl Pts',(108.12457611427,21.925521805893,31.));
#94895=CARTESIAN_POINT('Ctrl Pts',(108.12457611427,21.925521805893,26.));
#94896=CARTESIAN_POINT('Ctrl Pts',(108.127671920362,21.9595309601629,31.));
#94897=CARTESIAN_POINT('Ctrl Pts',(108.127671920362,21.9595309601629,26.));
#94898=CARTESIAN_POINT('Ctrl Pts',(108.131337578276,21.9940041198301,31.));
#94899=CARTESIAN_POINT('Ctrl Pts',(108.131337578276,21.9940041198301,26.));
#94900=CARTESIAN_POINT('Ctrl Pts',(108.135569853985,22.0289349713044,31.));
#94901=CARTESIAN_POINT('Ctrl Pts',(108.135569853985,22.0289349713044,26.));
#94902=CARTESIAN_POINT('Ctrl Pts',(108.139405777158,22.0572417527814,31.));
#94903=CARTESIAN_POINT('Ctrl Pts',(108.139405777158,22.0572417527814,26.));
#94904=CARTESIAN_POINT('Ctrl Pts',(108.142534384927,22.0786740240772,31.));
#94905=CARTESIAN_POINT('Ctrl Pts',(108.142534384927,22.0786740240772,26.));
#94906=CARTESIAN_POINT('Ctrl Pts',(108.14473177204,22.0930519020204,31.));
#94907=CARTESIAN_POINT('Ctrl Pts',(108.14473177204,22.0930519020204,26.));
#94908=CARTESIAN_POINT('Ctrl Pts',(108.145858377777,22.1002632652963,31.));
#94909=CARTESIAN_POINT('Ctrl Pts',(108.145858377777,22.1002632652963,26.));
#94910=CARTESIAN_POINT('Ctrl Pts',(108.195382868896,21.297228010781,31.));
#94911=CARTESIAN_POINT('Ctrl Pts',(108.194291116192,21.2993147395202,31.));
#94912=CARTESIAN_POINT('Ctrl Pts',(108.192099987029,21.3036628730427,31.));
#94913=CARTESIAN_POINT('Ctrl Pts',(108.188790420037,21.3107091062263,31.));
#94914=CARTESIAN_POINT('Ctrl Pts',(108.184331851862,21.3211540061394,31.));
#94915=CARTESIAN_POINT('Ctrl Pts',(108.17868709721,21.3359599004046,31.));
#94916=CARTESIAN_POINT('Ctrl Pts',(108.172986416033,21.3524951721887,31.));
#94917=CARTESIAN_POINT('Ctrl Pts',(108.167261205405,21.3707055346857,31.));
#94918=CARTESIAN_POINT('Ctrl Pts',(108.161565843382,21.3904834307621,31.));
#94919=CARTESIAN_POINT('Ctrl Pts',(108.155978401058,21.4116645975863,31.));
#94920=CARTESIAN_POINT('Ctrl Pts',(108.150587396044,21.4340592952825,31.));
#94921=CARTESIAN_POINT('Ctrl Pts',(108.14548095304,21.4574771160767,31.));
#94922=CARTESIAN_POINT('Ctrl Pts',(108.140736063183,21.4817516412614,31.));
#94923=CARTESIAN_POINT('Ctrl Pts',(108.136405082636,21.5067708088092,31.));
#94924=CARTESIAN_POINT('Ctrl Pts',(108.132512853008,21.5324835838215,31.));
#94925=CARTESIAN_POINT('Ctrl Pts',(108.129067047013,21.5588771351329,31.));
#94926=CARTESIAN_POINT('Ctrl Pts',(108.126065158383,21.5859611128485,31.));
#94927=CARTESIAN_POINT('Ctrl Pts',(108.123502124654,21.6137504395681,31.));
#94928=CARTESIAN_POINT('Ctrl Pts',(108.121378863907,21.6422453943083,31.));
#94929=CARTESIAN_POINT('Ctrl Pts',(108.119705321903,21.6714250926182,31.));
#94930=CARTESIAN_POINT('Ctrl Pts',(108.118496961822,21.7012568937955,31.));
#94931=CARTESIAN_POINT('Ctrl Pts',(108.117772886147,21.7317015453796,31.));
#94932=CARTESIAN_POINT('Ctrl Pts',(108.117553349757,21.7627194836669,31.));
#94933=CARTESIAN_POINT('Ctrl Pts',(108.117857140141,21.7942773949572,31.));
#94934=CARTESIAN_POINT('Ctrl Pts',(108.118699969278,21.8263513619102,31.));
#94935=CARTESIAN_POINT('Ctrl Pts',(108.120094755383,21.8589241514383,31.));
#94936=CARTESIAN_POINT('Ctrl Pts',(108.122051296525,21.8919838210329,31.));
#94937=CARTESIAN_POINT('Ctrl Pts',(108.12457611427,21.925521805893,31.));
#94938=CARTESIAN_POINT('Ctrl Pts',(108.127671920362,21.9595309601629,31.));
#94939=CARTESIAN_POINT('Ctrl Pts',(108.131337578276,21.9940041198301,31.));
#94940=CARTESIAN_POINT('Ctrl Pts',(108.135569853985,22.0289349713044,31.));
#94941=CARTESIAN_POINT('Ctrl Pts',(108.139405777158,22.0572417527814,31.));
#94942=CARTESIAN_POINT('Ctrl Pts',(108.142534384927,22.0786740240772,31.));
#94943=CARTESIAN_POINT('Ctrl Pts',(108.14473177204,22.0930519020204,31.));
#94944=CARTESIAN_POINT('Ctrl Pts',(108.145858377777,22.1002632652963,31.));
#94945=CARTESIAN_POINT('Ctrl Pts',(108.195382868896,21.297228010781,26.));
#94946=CARTESIAN_POINT('Ctrl Pts',(108.194291116192,21.2993147395202,26.));
#94947=CARTESIAN_POINT('Ctrl Pts',(108.192099987029,21.3036628730427,26.));
#94948=CARTESIAN_POINT('Ctrl Pts',(108.188790420037,21.3107091062263,26.));
#94949=CARTESIAN_POINT('Ctrl Pts',(108.184331851862,21.3211540061394,26.));
#94950=CARTESIAN_POINT('Ctrl Pts',(108.17868709721,21.3359599004046,26.));
#94951=CARTESIAN_POINT('Ctrl Pts',(108.172986416033,21.3524951721887,26.));
#94952=CARTESIAN_POINT('Ctrl Pts',(108.167261205405,21.3707055346857,26.));
#94953=CARTESIAN_POINT('Ctrl Pts',(108.161565843382,21.3904834307621,26.));
#94954=CARTESIAN_POINT('Ctrl Pts',(108.155978401058,21.4116645975863,26.));
#94955=CARTESIAN_POINT('Ctrl Pts',(108.150587396044,21.4340592952825,26.));
#94956=CARTESIAN_POINT('Ctrl Pts',(108.14548095304,21.4574771160767,26.));
#94957=CARTESIAN_POINT('Ctrl Pts',(108.140736063183,21.4817516412614,26.));
#94958=CARTESIAN_POINT('Ctrl Pts',(108.136405082636,21.5067708088092,26.));
#94959=CARTESIAN_POINT('Ctrl Pts',(108.132512853008,21.5324835838215,26.));
#94960=CARTESIAN_POINT('Ctrl Pts',(108.129067047013,21.5588771351329,26.));
#94961=CARTESIAN_POINT('Ctrl Pts',(108.126065158383,21.5859611128485,26.));
#94962=CARTESIAN_POINT('Ctrl Pts',(108.123502124654,21.6137504395681,26.));
#94963=CARTESIAN_POINT('Ctrl Pts',(108.121378863907,21.6422453943083,26.));
#94964=CARTESIAN_POINT('Ctrl Pts',(108.119705321903,21.6714250926182,26.));
#94965=CARTESIAN_POINT('Ctrl Pts',(108.118496961822,21.7012568937955,26.));
#94966=CARTESIAN_POINT('Ctrl Pts',(108.117772886147,21.7317015453796,26.));
#94967=CARTESIAN_POINT('Ctrl Pts',(108.117553349757,21.7627194836669,26.));
#94968=CARTESIAN_POINT('Ctrl Pts',(108.117857140141,21.7942773949572,26.));
#94969=CARTESIAN_POINT('Ctrl Pts',(108.118699969278,21.8263513619102,26.));
#94970=CARTESIAN_POINT('Ctrl Pts',(108.120094755383,21.8589241514383,26.));
#94971=CARTESIAN_POINT('Ctrl Pts',(108.122051296525,21.8919838210329,26.));
#94972=CARTESIAN_POINT('Ctrl Pts',(108.12457611427,21.925521805893,26.));
#94973=CARTESIAN_POINT('Ctrl Pts',(108.127671920362,21.9595309601629,26.));
#94974=CARTESIAN_POINT('Ctrl Pts',(108.131337578276,21.9940041198301,26.));
#94975=CARTESIAN_POINT('Ctrl Pts',(108.135569853985,22.0289349713044,26.));
#94976=CARTESIAN_POINT('Ctrl Pts',(108.139405777158,22.0572417527814,26.));
#94977=CARTESIAN_POINT('Ctrl Pts',(108.142534384927,22.0786740240772,26.));
#94978=CARTESIAN_POINT('Ctrl Pts',(108.14473177204,22.0930519020204,26.));
#94979=CARTESIAN_POINT('Ctrl Pts',(108.145858377777,22.1002632652963,26.));
#94980=CARTESIAN_POINT('Origin',(108.525485805931,21.5597921651915,31.));
#94981=CARTESIAN_POINT('Origin',(109.652122916228,21.2061825485438,31.));
#94982=CARTESIAN_POINT('',(109.59454570101,21.7368385510191,31.));
#94983=CARTESIAN_POINT('',(109.59454570101,21.7368385510191,31.));
#94984=CARTESIAN_POINT('',(109.59454570101,21.7368385510191,26.));
#94985=CARTESIAN_POINT('',(109.59454570101,21.7368385510191,31.));
#94986=CARTESIAN_POINT('',(109.59454570101,21.7368385510191,26.));
#94987=CARTESIAN_POINT('Origin',(110.40545429899,21.7368385510191,31.));
#94988=CARTESIAN_POINT('',(110.40545429899,21.7368385510191,26.));
#94989=CARTESIAN_POINT('',(110.347877083772,21.2061825485438,26.));
#94990=CARTESIAN_POINT('',(110.40545429899,21.7368385510191,31.));
#94991=CARTESIAN_POINT('',(110.40545429899,21.7368385510191,31.));
#94992=CARTESIAN_POINT('',(110.347877083772,21.2061825485438,31.));
#94993=CARTESIAN_POINT('Ctrl Pts',(110.143900675185,22.4976985887986,31.));
#94994=CARTESIAN_POINT('Ctrl Pts',(110.143900675185,22.4976985887986,26.));
#94995=CARTESIAN_POINT('Ctrl Pts',(110.147701192472,22.4914672912168,31.));
#94996=CARTESIAN_POINT('Ctrl Pts',(110.147701192472,22.4914672912168,26.));
#94997=CARTESIAN_POINT('Ctrl Pts',(110.155233489225,22.4790247677066,31.));
#94998=CARTESIAN_POINT('Ctrl Pts',(110.155233489225,22.4790247677066,26.));
#94999=CARTESIAN_POINT('Ctrl Pts',(110.166325721145,22.4604211972804,31.));
#95000=CARTESIAN_POINT('Ctrl Pts',(110.166325721145,22.4604211972804,26.));
#95001=CARTESIAN_POINT('Ctrl Pts',(110.180702188389,22.4357370854887,31.));
#95002=CARTESIAN_POINT('Ctrl Pts',(110.180702188389,22.4357370854887,26.));
#95003=CARTESIAN_POINT('Ctrl Pts',(110.197979759379,22.4050848085535,31.));
#95004=CARTESIAN_POINT('Ctrl Pts',(110.197979759379,22.4050848085535,26.));
#95005=CARTESIAN_POINT('Ctrl Pts',(110.214558692659,22.3746385484685,31.));
#95006=CARTESIAN_POINT('Ctrl Pts',(110.214558692659,22.3746385484685,26.));
#95007=CARTESIAN_POINT('Ctrl Pts',(110.23043358432,22.3444029006218,31.));
#95008=CARTESIAN_POINT('Ctrl Pts',(110.23043358432,22.3444029006218,26.));
#95009=CARTESIAN_POINT('Ctrl Pts',(110.245600642837,22.314384048769,31.));
#95010=CARTESIAN_POINT('Ctrl Pts',(110.245600642837,22.314384048769,26.));
#95011=CARTESIAN_POINT('Ctrl Pts',(110.26005963895,22.2845896325587,31.));
#95012=CARTESIAN_POINT('Ctrl Pts',(110.26005963895,22.2845896325587,26.));
#95013=CARTESIAN_POINT('Ctrl Pts',(110.27381332019,22.2550300605308,31.));
#95014=CARTESIAN_POINT('Ctrl Pts',(110.27381332019,22.2550300605308,26.));
#95015=CARTESIAN_POINT('Ctrl Pts',(110.286866168579,22.2257201156837,31.));
#95016=CARTESIAN_POINT('Ctrl Pts',(110.286866168579,22.2257201156837,26.));
#95017=CARTESIAN_POINT('Ctrl Pts',(110.299223524153,22.1966806629003,31.));
#95018=CARTESIAN_POINT('Ctrl Pts',(110.299223524153,22.1966806629003,26.));
#95019=CARTESIAN_POINT('Ctrl Pts',(110.310890750103,22.1679398116366,31.));
#95020=CARTESIAN_POINT('Ctrl Pts',(110.310890750103,22.1679398116366,26.));
#95021=CARTESIAN_POINT('Ctrl Pts',(110.321872455192,22.1395355293992,31.));
#95022=CARTESIAN_POINT('Ctrl Pts',(110.321872455192,22.1395355293992,26.));
#95023=CARTESIAN_POINT('Ctrl Pts',(110.332172212114,22.1115121194901,31.));
#95024=CARTESIAN_POINT('Ctrl Pts',(110.332172212114,22.1115121194901,26.));
#95025=CARTESIAN_POINT('Ctrl Pts',(110.341792648001,22.0839131566587,31.));
#95026=CARTESIAN_POINT('Ctrl Pts',(110.341792648001,22.0839131566587,26.));
#95027=CARTESIAN_POINT('Ctrl Pts',(110.350735557918,22.056774714484,31.));
#95028=CARTESIAN_POINT('Ctrl Pts',(110.350735557918,22.056774714484,26.));
#95029=CARTESIAN_POINT('Ctrl Pts',(110.359002138426,22.0301198937606,31.));
#95030=CARTESIAN_POINT('Ctrl Pts',(110.359002138426,22.0301198937606,26.));
#95031=CARTESIAN_POINT('Ctrl Pts',(110.366593344504,22.0039487880456,31.));
#95032=CARTESIAN_POINT('Ctrl Pts',(110.366593344504,22.0039487880456,26.));
#95033=CARTESIAN_POINT('Ctrl Pts',(110.373510209678,21.978245673333,31.));
#95034=CARTESIAN_POINT('Ctrl Pts',(110.373510209678,21.978245673333,26.));
#95035=CARTESIAN_POINT('Ctrl Pts',(110.379754111393,21.9530006749816,31.));
#95036=CARTESIAN_POINT('Ctrl Pts',(110.379754111393,21.9530006749816,26.));
#95037=CARTESIAN_POINT('Ctrl Pts',(110.385327228035,21.9282285836627,31.));
#95038=CARTESIAN_POINT('Ctrl Pts',(110.385327228035,21.9282285836627,26.));
#95039=CARTESIAN_POINT('Ctrl Pts',(110.390232980042,21.9039860559466,31.));
#95040=CARTESIAN_POINT('Ctrl Pts',(110.390232980042,21.9039860559466,26.));
#95041=CARTESIAN_POINT('Ctrl Pts',(110.39447685392,21.8803966594834,31.));
#95042=CARTESIAN_POINT('Ctrl Pts',(110.39447685392,21.8803966594834,26.));
#95043=CARTESIAN_POINT('Ctrl Pts',(110.398066294513,21.8576436083425,31.));
#95044=CARTESIAN_POINT('Ctrl Pts',(110.398066294513,21.8576436083425,26.));
#95045=CARTESIAN_POINT('Ctrl Pts',(110.401009852528,21.8359365402324,31.));
#95046=CARTESIAN_POINT('Ctrl Pts',(110.401009852528,21.8359365402324,26.));
#95047=CARTESIAN_POINT('Ctrl Pts',(110.403316697266,21.8154846261632,31.));
#95048=CARTESIAN_POINT('Ctrl Pts',(110.403316697266,21.8154846261632,26.));
#95049=CARTESIAN_POINT('Ctrl Pts',(110.404996096355,21.7964695017177,31.));
#95050=CARTESIAN_POINT('Ctrl Pts',(110.404996096355,21.7964695017177,26.));
#95051=CARTESIAN_POINT('Ctrl Pts',(110.406057128242,21.7790113463118,31.));
#95052=CARTESIAN_POINT('Ctrl Pts',(110.406057128242,21.7790113463118,26.));
#95053=CARTESIAN_POINT('Ctrl Pts',(110.406508025383,21.7631723295541,31.));
#95054=CARTESIAN_POINT('Ctrl Pts',(110.406508025383,21.7631723295541,26.));
#95055=CARTESIAN_POINT('Ctrl Pts',(110.406385935655,21.7518162801327,31.));
#95056=CARTESIAN_POINT('Ctrl Pts',(110.406385935655,21.7518162801327,26.));
#95057=CARTESIAN_POINT('Ctrl Pts',(110.406024771161,21.7440398930577,31.));
#95058=CARTESIAN_POINT('Ctrl Pts',(110.406024771161,21.7440398930577,26.));
#95059=CARTESIAN_POINT('Ctrl Pts',(110.405664390446,21.7391842326632,31.));
#95060=CARTESIAN_POINT('Ctrl Pts',(110.405664390446,21.7391842326632,26.));
#95061=CARTESIAN_POINT('Ctrl Pts',(110.40545429899,21.7368385510191,31.));
#95062=CARTESIAN_POINT('Ctrl Pts',(110.40545429899,21.7368385510191,26.));
#95063=CARTESIAN_POINT('',(110.143900675185,22.4976985887986,31.));
#95064=CARTESIAN_POINT('Ctrl Pts',(110.40545429899,21.7368385510191,31.));
#95065=CARTESIAN_POINT('Ctrl Pts',(110.405664390446,21.7391842326632,31.));
#95066=CARTESIAN_POINT('Ctrl Pts',(110.406024771161,21.7440398930577,31.));
#95067=CARTESIAN_POINT('Ctrl Pts',(110.406385935655,21.7518162801327,31.));
#95068=CARTESIAN_POINT('Ctrl Pts',(110.406508025383,21.7631723295541,31.));
#95069=CARTESIAN_POINT('Ctrl Pts',(110.406057128242,21.7790113463118,31.));
#95070=CARTESIAN_POINT('Ctrl Pts',(110.404996096355,21.7964695017177,31.));
#95071=CARTESIAN_POINT('Ctrl Pts',(110.403316697266,21.8154846261632,31.));
#95072=CARTESIAN_POINT('Ctrl Pts',(110.401009852528,21.8359365402324,31.));
#95073=CARTESIAN_POINT('Ctrl Pts',(110.398066294513,21.8576436083425,31.));
#95074=CARTESIAN_POINT('Ctrl Pts',(110.39447685392,21.8803966594834,31.));
#95075=CARTESIAN_POINT('Ctrl Pts',(110.390232980042,21.9039860559466,31.));
#95076=CARTESIAN_POINT('Ctrl Pts',(110.385327228035,21.9282285836627,31.));
#95077=CARTESIAN_POINT('Ctrl Pts',(110.379754111393,21.9530006749816,31.));
#95078=CARTESIAN_POINT('Ctrl Pts',(110.373510209678,21.978245673333,31.));
#95079=CARTESIAN_POINT('Ctrl Pts',(110.366593344504,22.0039487880456,31.));
#95080=CARTESIAN_POINT('Ctrl Pts',(110.359002138426,22.0301198937606,31.));
#95081=CARTESIAN_POINT('Ctrl Pts',(110.350735557918,22.056774714484,31.));
#95082=CARTESIAN_POINT('Ctrl Pts',(110.341792648001,22.0839131566587,31.));
#95083=CARTESIAN_POINT('Ctrl Pts',(110.332172212114,22.1115121194901,31.));
#95084=CARTESIAN_POINT('Ctrl Pts',(110.321872455192,22.1395355293992,31.));
#95085=CARTESIAN_POINT('Ctrl Pts',(110.310890750103,22.1679398116366,31.));
#95086=CARTESIAN_POINT('Ctrl Pts',(110.299223524153,22.1966806629003,31.));
#95087=CARTESIAN_POINT('Ctrl Pts',(110.286866168579,22.2257201156837,31.));
#95088=CARTESIAN_POINT('Ctrl Pts',(110.27381332019,22.2550300605308,31.));
#95089=CARTESIAN_POINT('Ctrl Pts',(110.26005963895,22.2845896325587,31.));
#95090=CARTESIAN_POINT('Ctrl Pts',(110.245600642837,22.314384048769,31.));
#95091=CARTESIAN_POINT('Ctrl Pts',(110.23043358432,22.3444029006218,31.));
#95092=CARTESIAN_POINT('Ctrl Pts',(110.214558692659,22.3746385484685,31.));
#95093=CARTESIAN_POINT('Ctrl Pts',(110.197979759379,22.4050848085535,31.));
#95094=CARTESIAN_POINT('Ctrl Pts',(110.180702188389,22.4357370854887,31.));
#95095=CARTESIAN_POINT('Ctrl Pts',(110.166325721145,22.4604211972804,31.));
#95096=CARTESIAN_POINT('Ctrl Pts',(110.155233489225,22.4790247677066,31.));
#95097=CARTESIAN_POINT('Ctrl Pts',(110.147701192472,22.4914672912168,31.));
#95098=CARTESIAN_POINT('Ctrl Pts',(110.143900675185,22.4976985887986,31.));
#95099=CARTESIAN_POINT('',(110.143900675185,22.4976985887986,26.));
#95100=CARTESIAN_POINT('Ctrl Pts',(110.143900675185,22.4976985887986,26.));
#95101=CARTESIAN_POINT('Ctrl Pts',(110.147701192472,22.4914672912168,26.));
#95102=CARTESIAN_POINT('Ctrl Pts',(110.155233489225,22.4790247677066,26.));
#95103=CARTESIAN_POINT('Ctrl Pts',(110.166325721145,22.4604211972804,26.));
#95104=CARTESIAN_POINT('Ctrl Pts',(110.180702188389,22.4357370854887,26.));
#95105=CARTESIAN_POINT('Ctrl Pts',(110.197979759379,22.4050848085535,26.));
#95106=CARTESIAN_POINT('Ctrl Pts',(110.214558692659,22.3746385484685,26.));
#95107=CARTESIAN_POINT('Ctrl Pts',(110.23043358432,22.3444029006218,26.));
#95108=CARTESIAN_POINT('Ctrl Pts',(110.245600642837,22.314384048769,26.));
#95109=CARTESIAN_POINT('Ctrl Pts',(110.26005963895,22.2845896325587,26.));
#95110=CARTESIAN_POINT('Ctrl Pts',(110.27381332019,22.2550300605308,26.));
#95111=CARTESIAN_POINT('Ctrl Pts',(110.286866168579,22.2257201156837,26.));
#95112=CARTESIAN_POINT('Ctrl Pts',(110.299223524153,22.1966806629003,26.));
#95113=CARTESIAN_POINT('Ctrl Pts',(110.310890750103,22.1679398116366,26.));
#95114=CARTESIAN_POINT('Ctrl Pts',(110.321872455192,22.1395355293992,26.));
#95115=CARTESIAN_POINT('Ctrl Pts',(110.332172212114,22.1115121194901,26.));
#95116=CARTESIAN_POINT('Ctrl Pts',(110.341792648001,22.0839131566587,26.));
#95117=CARTESIAN_POINT('Ctrl Pts',(110.350735557918,22.056774714484,26.));
#95118=CARTESIAN_POINT('Ctrl Pts',(110.359002138426,22.0301198937606,26.));
#95119=CARTESIAN_POINT('Ctrl Pts',(110.366593344504,22.0039487880456,26.));
#95120=CARTESIAN_POINT('Ctrl Pts',(110.373510209678,21.978245673333,26.));
#95121=CARTESIAN_POINT('Ctrl Pts',(110.379754111393,21.9530006749816,26.));
#95122=CARTESIAN_POINT('Ctrl Pts',(110.385327228035,21.9282285836627,26.));
#95123=CARTESIAN_POINT('Ctrl Pts',(110.390232980042,21.9039860559466,26.));
#95124=CARTESIAN_POINT('Ctrl Pts',(110.39447685392,21.8803966594834,26.));
#95125=CARTESIAN_POINT('Ctrl Pts',(110.398066294513,21.8576436083425,26.));
#95126=CARTESIAN_POINT('Ctrl Pts',(110.401009852528,21.8359365402324,26.));
#95127=CARTESIAN_POINT('Ctrl Pts',(110.403316697266,21.8154846261632,26.));
#95128=CARTESIAN_POINT('Ctrl Pts',(110.404996096355,21.7964695017177,26.));
#95129=CARTESIAN_POINT('Ctrl Pts',(110.406057128242,21.7790113463118,26.));
#95130=CARTESIAN_POINT('Ctrl Pts',(110.406508025383,21.7631723295541,26.));
#95131=CARTESIAN_POINT('Ctrl Pts',(110.406385935655,21.7518162801327,26.));
#95132=CARTESIAN_POINT('Ctrl Pts',(110.406024771161,21.7440398930577,26.));
#95133=CARTESIAN_POINT('Ctrl Pts',(110.405664390446,21.7391842326632,26.));
#95134=CARTESIAN_POINT('Ctrl Pts',(110.40545429899,21.7368385510191,26.));
#95135=CARTESIAN_POINT('',(110.143900675185,22.4976985887986,31.));
#95136=CARTESIAN_POINT('Origin',(110.,17.999999999997,31.));
#95137=CARTESIAN_POINT('',(109.856099324815,22.4976985887986,31.));
#95138=CARTESIAN_POINT('Origin',(110.,17.999999999997,31.));
#95139=CARTESIAN_POINT('',(109.856099324815,22.4976985887986,26.));
#95140=CARTESIAN_POINT('Origin',(110.,17.999999999997,26.));
#95141=CARTESIAN_POINT('',(109.856099324815,22.4976985887986,31.));
#95142=CARTESIAN_POINT('Ctrl Pts',(109.59454570101,21.7368385510191,31.));
#95143=CARTESIAN_POINT('Ctrl Pts',(109.59454570101,21.7368385510191,26.));
#95144=CARTESIAN_POINT('Ctrl Pts',(109.594335609548,21.7391842326635,31.));
#95145=CARTESIAN_POINT('Ctrl Pts',(109.594335609548,21.7391842326635,26.));
#95146=CARTESIAN_POINT('Ctrl Pts',(109.593975228822,21.7440398930583,31.));
#95147=CARTESIAN_POINT('Ctrl Pts',(109.593975228822,21.7440398930583,26.));
#95148=CARTESIAN_POINT('Ctrl Pts',(109.593614064317,21.7518162801338,31.));
#95149=CARTESIAN_POINT('Ctrl Pts',(109.593614064317,21.7518162801338,26.));
#95150=CARTESIAN_POINT('Ctrl Pts',(109.593491974585,21.7631723295554,31.));
#95151=CARTESIAN_POINT('Ctrl Pts',(109.593491974585,21.7631723295554,26.));
#95152=CARTESIAN_POINT('Ctrl Pts',(109.593942871732,21.7790113463128,31.));
#95153=CARTESIAN_POINT('Ctrl Pts',(109.593942871732,21.7790113463128,26.));
#95154=CARTESIAN_POINT('Ctrl Pts',(109.595003903633,21.7964695017181,31.));
#95155=CARTESIAN_POINT('Ctrl Pts',(109.595003903633,21.7964695017181,26.));
#95156=CARTESIAN_POINT('Ctrl Pts',(109.59668330274,21.815484626163,31.));
#95157=CARTESIAN_POINT('Ctrl Pts',(109.59668330274,21.815484626163,26.));
#95158=CARTESIAN_POINT('Ctrl Pts',(109.598990147492,21.8359365402318,31.));
#95159=CARTESIAN_POINT('Ctrl Pts',(109.598990147492,21.8359365402318,26.));
#95160=CARTESIAN_POINT('Ctrl Pts',(109.601933705511,21.8576436083419,31.));
#95161=CARTESIAN_POINT('Ctrl Pts',(109.601933705511,21.8576436083419,26.));
#95162=CARTESIAN_POINT('Ctrl Pts',(109.6055231461,21.8803966594829,31.));
#95163=CARTESIAN_POINT('Ctrl Pts',(109.6055231461,21.8803966594829,26.));
#95164=CARTESIAN_POINT('Ctrl Pts',(109.609767019965,21.9039860559465,31.));
#95165=CARTESIAN_POINT('Ctrl Pts',(109.609767019965,21.9039860559465,26.));
#95166=CARTESIAN_POINT('Ctrl Pts',(109.614672771959,21.9282285836629,31.));
#95167=CARTESIAN_POINT('Ctrl Pts',(109.614672771959,21.9282285836629,26.));
#95168=CARTESIAN_POINT('Ctrl Pts',(109.620245888588,21.9530006749818,31.));
#95169=CARTESIAN_POINT('Ctrl Pts',(109.620245888588,21.9530006749818,26.));
#95170=CARTESIAN_POINT('Ctrl Pts',(109.626489790297,21.9782456733333,31.));
#95171=CARTESIAN_POINT('Ctrl Pts',(109.626489790297,21.9782456733333,26.));
#95172=CARTESIAN_POINT('Ctrl Pts',(109.633406655472,22.0039487880458,31.));
#95173=CARTESIAN_POINT('Ctrl Pts',(109.633406655472,22.0039487880458,26.));
#95174=CARTESIAN_POINT('Ctrl Pts',(109.640997861563,22.0301198937606,31.));
#95175=CARTESIAN_POINT('Ctrl Pts',(109.640997861563,22.0301198937606,26.));
#95176=CARTESIAN_POINT('Ctrl Pts',(109.649264442091,22.056774714484,31.));
#95177=CARTESIAN_POINT('Ctrl Pts',(109.649264442091,22.056774714484,26.));
#95178=CARTESIAN_POINT('Ctrl Pts',(109.65820735203,22.0839131566587,31.));
#95179=CARTESIAN_POINT('Ctrl Pts',(109.65820735203,22.0839131566587,26.));
#95180=CARTESIAN_POINT('Ctrl Pts',(109.667827787931,22.1115121194901,31.));
#95181=CARTESIAN_POINT('Ctrl Pts',(109.667827787931,22.1115121194901,26.));
#95182=CARTESIAN_POINT('Ctrl Pts',(109.678127544852,22.1395355293993,31.));
#95183=CARTESIAN_POINT('Ctrl Pts',(109.678127544852,22.1395355293993,26.));
#95184=CARTESIAN_POINT('Ctrl Pts',(109.689109249922,22.1679398116367,31.));
#95185=CARTESIAN_POINT('Ctrl Pts',(109.689109249922,22.1679398116367,26.));
#95186=CARTESIAN_POINT('Ctrl Pts',(109.700776475833,22.1966806629002,31.));
#95187=CARTESIAN_POINT('Ctrl Pts',(109.700776475833,22.1966806629002,26.));
#95188=CARTESIAN_POINT('Ctrl Pts',(109.713133831361,22.2257201156836,31.));
#95189=CARTESIAN_POINT('Ctrl Pts',(109.713133831361,22.2257201156836,26.));
#95190=CARTESIAN_POINT('Ctrl Pts',(109.726186679714,22.2550300605307,31.));
#95191=CARTESIAN_POINT('Ctrl Pts',(109.726186679714,22.2550300605307,26.));
#95192=CARTESIAN_POINT('Ctrl Pts',(109.739940360947,22.2845896325585,31.));
#95193=CARTESIAN_POINT('Ctrl Pts',(109.739940360947,22.2845896325585,26.));
#95194=CARTESIAN_POINT('Ctrl Pts',(109.754399357095,22.3143840487689,31.));
#95195=CARTESIAN_POINT('Ctrl Pts',(109.754399357095,22.3143840487689,26.));
#95196=CARTESIAN_POINT('Ctrl Pts',(109.769566415695,22.3444029006219,31.));
#95197=CARTESIAN_POINT('Ctrl Pts',(109.769566415695,22.3444029006219,26.));
#95198=CARTESIAN_POINT('Ctrl Pts',(109.785441307467,22.3746385484687,31.));
#95199=CARTESIAN_POINT('Ctrl Pts',(109.785441307467,22.3746385484687,26.));
#95200=CARTESIAN_POINT('Ctrl Pts',(109.802020240853,22.4050848085539,31.));
#95201=CARTESIAN_POINT('Ctrl Pts',(109.802020240853,22.4050848085539,26.));
#95202=CARTESIAN_POINT('Ctrl Pts',(109.819297811894,22.435737085489,31.));
#95203=CARTESIAN_POINT('Ctrl Pts',(109.819297811894,22.435737085489,26.));
#95204=CARTESIAN_POINT('Ctrl Pts',(109.833674279097,22.4604211972807,31.));
#95205=CARTESIAN_POINT('Ctrl Pts',(109.833674279097,22.4604211972807,26.));
#95206=CARTESIAN_POINT('Ctrl Pts',(109.844766510922,22.4790247677067,31.));
#95207=CARTESIAN_POINT('Ctrl Pts',(109.844766510922,22.4790247677067,26.));
#95208=CARTESIAN_POINT('Ctrl Pts',(109.852298807583,22.4914672912169,31.));
#95209=CARTESIAN_POINT('Ctrl Pts',(109.852298807583,22.4914672912169,26.));
#95210=CARTESIAN_POINT('Ctrl Pts',(109.856099324815,22.4976985887986,31.));
#95211=CARTESIAN_POINT('Ctrl Pts',(109.856099324815,22.4976985887986,26.));
#95212=CARTESIAN_POINT('Ctrl Pts',(109.59454570101,21.7368385510191,31.));
#95213=CARTESIAN_POINT('Ctrl Pts',(109.594335609548,21.7391842326635,31.));
#95214=CARTESIAN_POINT('Ctrl Pts',(109.593975228822,21.7440398930583,31.));
#95215=CARTESIAN_POINT('Ctrl Pts',(109.593614064317,21.7518162801338,31.));
#95216=CARTESIAN_POINT('Ctrl Pts',(109.593491974585,21.7631723295554,31.));
#95217=CARTESIAN_POINT('Ctrl Pts',(109.593942871732,21.7790113463128,31.));
#95218=CARTESIAN_POINT('Ctrl Pts',(109.595003903633,21.7964695017181,31.));
#95219=CARTESIAN_POINT('Ctrl Pts',(109.59668330274,21.815484626163,31.));
#95220=CARTESIAN_POINT('Ctrl Pts',(109.598990147492,21.8359365402318,31.));
#95221=CARTESIAN_POINT('Ctrl Pts',(109.601933705511,21.8576436083419,31.));
#95222=CARTESIAN_POINT('Ctrl Pts',(109.6055231461,21.8803966594829,31.));
#95223=CARTESIAN_POINT('Ctrl Pts',(109.609767019965,21.9039860559465,31.));
#95224=CARTESIAN_POINT('Ctrl Pts',(109.614672771959,21.9282285836629,31.));
#95225=CARTESIAN_POINT('Ctrl Pts',(109.620245888588,21.9530006749818,31.));
#95226=CARTESIAN_POINT('Ctrl Pts',(109.626489790297,21.9782456733333,31.));
#95227=CARTESIAN_POINT('Ctrl Pts',(109.633406655472,22.0039487880458,31.));
#95228=CARTESIAN_POINT('Ctrl Pts',(109.640997861563,22.0301198937606,31.));
#95229=CARTESIAN_POINT('Ctrl Pts',(109.649264442091,22.056774714484,31.));
#95230=CARTESIAN_POINT('Ctrl Pts',(109.65820735203,22.0839131566587,31.));
#95231=CARTESIAN_POINT('Ctrl Pts',(109.667827787931,22.1115121194901,31.));
#95232=CARTESIAN_POINT('Ctrl Pts',(109.678127544852,22.1395355293993,31.));
#95233=CARTESIAN_POINT('Ctrl Pts',(109.689109249922,22.1679398116367,31.));
#95234=CARTESIAN_POINT('Ctrl Pts',(109.700776475833,22.1966806629002,31.));
#95235=CARTESIAN_POINT('Ctrl Pts',(109.713133831361,22.2257201156836,31.));
#95236=CARTESIAN_POINT('Ctrl Pts',(109.726186679714,22.2550300605307,31.));
#95237=CARTESIAN_POINT('Ctrl Pts',(109.739940360947,22.2845896325585,31.));
#95238=CARTESIAN_POINT('Ctrl Pts',(109.754399357095,22.3143840487689,31.));
#95239=CARTESIAN_POINT('Ctrl Pts',(109.769566415695,22.3444029006219,31.));
#95240=CARTESIAN_POINT('Ctrl Pts',(109.785441307467,22.3746385484687,31.));
#95241=CARTESIAN_POINT('Ctrl Pts',(109.802020240853,22.4050848085539,31.));
#95242=CARTESIAN_POINT('Ctrl Pts',(109.819297811894,22.435737085489,31.));
#95243=CARTESIAN_POINT('Ctrl Pts',(109.833674279097,22.4604211972807,31.));
#95244=CARTESIAN_POINT('Ctrl Pts',(109.844766510922,22.4790247677067,31.));
#95245=CARTESIAN_POINT('Ctrl Pts',(109.852298807583,22.4914672912169,31.));
#95246=CARTESIAN_POINT('Ctrl Pts',(109.856099324815,22.4976985887986,31.));
#95247=CARTESIAN_POINT('Ctrl Pts',(109.59454570101,21.7368385510191,26.));
#95248=CARTESIAN_POINT('Ctrl Pts',(109.594335609548,21.7391842326635,26.));
#95249=CARTESIAN_POINT('Ctrl Pts',(109.593975228822,21.7440398930583,26.));
#95250=CARTESIAN_POINT('Ctrl Pts',(109.593614064317,21.7518162801338,26.));
#95251=CARTESIAN_POINT('Ctrl Pts',(109.593491974585,21.7631723295554,26.));
#95252=CARTESIAN_POINT('Ctrl Pts',(109.593942871732,21.7790113463128,26.));
#95253=CARTESIAN_POINT('Ctrl Pts',(109.595003903633,21.7964695017181,26.));
#95254=CARTESIAN_POINT('Ctrl Pts',(109.59668330274,21.815484626163,26.));
#95255=CARTESIAN_POINT('Ctrl Pts',(109.598990147492,21.8359365402318,26.));
#95256=CARTESIAN_POINT('Ctrl Pts',(109.601933705511,21.8576436083419,26.));
#95257=CARTESIAN_POINT('Ctrl Pts',(109.6055231461,21.8803966594829,26.));
#95258=CARTESIAN_POINT('Ctrl Pts',(109.609767019965,21.9039860559465,26.));
#95259=CARTESIAN_POINT('Ctrl Pts',(109.614672771959,21.9282285836629,26.));
#95260=CARTESIAN_POINT('Ctrl Pts',(109.620245888588,21.9530006749818,26.));
#95261=CARTESIAN_POINT('Ctrl Pts',(109.626489790297,21.9782456733333,26.));
#95262=CARTESIAN_POINT('Ctrl Pts',(109.633406655472,22.0039487880458,26.));
#95263=CARTESIAN_POINT('Ctrl Pts',(109.640997861563,22.0301198937606,26.));
#95264=CARTESIAN_POINT('Ctrl Pts',(109.649264442091,22.056774714484,26.));
#95265=CARTESIAN_POINT('Ctrl Pts',(109.65820735203,22.0839131566587,26.));
#95266=CARTESIAN_POINT('Ctrl Pts',(109.667827787931,22.1115121194901,26.));
#95267=CARTESIAN_POINT('Ctrl Pts',(109.678127544852,22.1395355293993,26.));
#95268=CARTESIAN_POINT('Ctrl Pts',(109.689109249922,22.1679398116367,26.));
#95269=CARTESIAN_POINT('Ctrl Pts',(109.700776475833,22.1966806629002,26.));
#95270=CARTESIAN_POINT('Ctrl Pts',(109.713133831361,22.2257201156836,26.));
#95271=CARTESIAN_POINT('Ctrl Pts',(109.726186679714,22.2550300605307,26.));
#95272=CARTESIAN_POINT('Ctrl Pts',(109.739940360947,22.2845896325585,26.));
#95273=CARTESIAN_POINT('Ctrl Pts',(109.754399357095,22.3143840487689,26.));
#95274=CARTESIAN_POINT('Ctrl Pts',(109.769566415695,22.3444029006219,26.));
#95275=CARTESIAN_POINT('Ctrl Pts',(109.785441307467,22.3746385484687,26.));
#95276=CARTESIAN_POINT('Ctrl Pts',(109.802020240853,22.4050848085539,26.));
#95277=CARTESIAN_POINT('Ctrl Pts',(109.819297811894,22.435737085489,26.));
#95278=CARTESIAN_POINT('Ctrl Pts',(109.833674279097,22.4604211972807,26.));
#95279=CARTESIAN_POINT('Ctrl Pts',(109.844766510922,22.4790247677067,26.));
#95280=CARTESIAN_POINT('Ctrl Pts',(109.852298807583,22.4914672912169,26.));
#95281=CARTESIAN_POINT('Ctrl Pts',(109.856099324815,22.4976985887986,26.));
#95282=CARTESIAN_POINT('Origin',(109.999999999984,21.8530912742719,31.));
#95283=CARTESIAN_POINT('Origin',(110.90555642494,21.0952532305533,31.));
#95284=CARTESIAN_POINT('',(111.055435274693,21.6075492963903,31.));
#95285=CARTESIAN_POINT('',(111.055435274693,21.6075492963903,31.));
#95286=CARTESIAN_POINT('',(111.055435274693,21.6075492963903,26.));
#95287=CARTESIAN_POINT('',(111.055435274693,21.6075492963903,31.));
#95288=CARTESIAN_POINT('',(111.055435274693,21.6075492963903,26.));
#95289=CARTESIAN_POINT('Origin',(111.804617131104,21.297228010781,31.));
#95290=CARTESIAN_POINT('',(111.804617131104,21.297228010781,26.));
#95291=CARTESIAN_POINT('',(111.548349459992,20.8289996376356,26.));
#95292=CARTESIAN_POINT('',(111.804617131104,21.297228010781,31.));
#95293=CARTESIAN_POINT('',(111.804617131104,21.297228010781,31.));
#95294=CARTESIAN_POINT('',(111.548349459992,20.8289996376356,31.));
#95295=CARTESIAN_POINT('Ctrl Pts',(111.854141622223,22.1002632652963,31.));
#95296=CARTESIAN_POINT('Ctrl Pts',(111.854141622223,22.1002632652963,26.));
#95297=CARTESIAN_POINT('Ctrl Pts',(111.855268228011,22.0930519019996,31.));
#95298=CARTESIAN_POINT('Ctrl Pts',(111.855268228011,22.0930519019996,26.));
#95299=CARTESIAN_POINT('Ctrl Pts',(111.85746561521,22.0786740240205,31.));
#95300=CARTESIAN_POINT('Ctrl Pts',(111.85746561521,22.0786740240205,26.));
#95301=CARTESIAN_POINT('Ctrl Pts',(111.860594223066,22.0572417526884,31.));
#95302=CARTESIAN_POINT('Ctrl Pts',(111.860594223066,22.0572417526884,26.));
#95303=CARTESIAN_POINT('Ctrl Pts',(111.864430146276,22.0289349711957,31.));
#95304=CARTESIAN_POINT('Ctrl Pts',(111.864430146276,22.0289349711957,26.));
#95305=CARTESIAN_POINT('Ctrl Pts',(111.868662421939,21.994004119741,31.));
#95306=CARTESIAN_POINT('Ctrl Pts',(111.868662421939,21.994004119741,26.));
#95307=CARTESIAN_POINT('Ctrl Pts',(111.872328079755,21.9595309601143,31.));
#95308=CARTESIAN_POINT('Ctrl Pts',(111.872328079755,21.9595309601143,26.));
#95309=CARTESIAN_POINT('Ctrl Pts',(111.875423885743,21.9255218058874,31.));
#95310=CARTESIAN_POINT('Ctrl Pts',(111.875423885743,21.9255218058874,26.));
#95311=CARTESIAN_POINT('Ctrl Pts',(111.877948703413,21.8919838210589,31.));
#95312=CARTESIAN_POINT('Ctrl Pts',(111.877948703413,21.8919838210589,26.));
#95313=CARTESIAN_POINT('Ctrl Pts',(111.879905244522,21.858924151478,31.));
#95314=CARTESIAN_POINT('Ctrl Pts',(111.879905244522,21.858924151478,26.));
#95315=CARTESIAN_POINT('Ctrl Pts',(111.881300030633,21.8263513619471,31.));
#95316=CARTESIAN_POINT('Ctrl Pts',(111.881300030633,21.8263513619471,26.));
#95317=CARTESIAN_POINT('Ctrl Pts',(111.882142859804,21.7942773949803,31.));
#95318=CARTESIAN_POINT('Ctrl Pts',(111.882142859804,21.7942773949803,26.));
#95319=CARTESIAN_POINT('Ctrl Pts',(111.88244665023,21.7627194836722,31.));
#95320=CARTESIAN_POINT('Ctrl Pts',(111.88244665023,21.7627194836722,26.));
#95321=CARTESIAN_POINT('Ctrl Pts',(111.882227113875,21.7317015453702,31.));
#95322=CARTESIAN_POINT('Ctrl Pts',(111.882227113875,21.7317015453702,26.));
#95323=CARTESIAN_POINT('Ctrl Pts',(111.881503038219,21.7012568937784,31.));
#95324=CARTESIAN_POINT('Ctrl Pts',(111.881503038219,21.7012568937784,26.));
#95325=CARTESIAN_POINT('Ctrl Pts',(111.880294678138,21.6714250926009,31.));
#95326=CARTESIAN_POINT('Ctrl Pts',(111.880294678138,21.6714250926009,26.));
#95327=CARTESIAN_POINT('Ctrl Pts',(111.878621136122,21.6422453942965,31.));
#95328=CARTESIAN_POINT('Ctrl Pts',(111.878621136122,21.6422453942965,26.));
#95329=CARTESIAN_POINT('Ctrl Pts',(111.876497875355,21.6137504395647,31.));
#95330=CARTESIAN_POINT('Ctrl Pts',(111.876497875355,21.6137504395647,26.));
#95331=CARTESIAN_POINT('Ctrl Pts',(111.873934841606,21.5859611128528,31.));
#95332=CARTESIAN_POINT('Ctrl Pts',(111.873934841606,21.5859611128528,26.));
#95333=CARTESIAN_POINT('Ctrl Pts',(111.870932952965,21.5588771351418,31.));
#95334=CARTESIAN_POINT('Ctrl Pts',(111.870932952965,21.5588771351418,26.));
#95335=CARTESIAN_POINT('Ctrl Pts',(111.867487146968,21.5324835838312,31.));
#95336=CARTESIAN_POINT('Ctrl Pts',(111.867487146968,21.5324835838312,26.));
#95337=CARTESIAN_POINT('Ctrl Pts',(111.863594917346,21.5067708088162,31.));
#95338=CARTESIAN_POINT('Ctrl Pts',(111.863594917346,21.5067708088162,26.));
#95339=CARTESIAN_POINT('Ctrl Pts',(111.859263936811,21.4817516412638,31.));
#95340=CARTESIAN_POINT('Ctrl Pts',(111.859263936811,21.4817516412638,26.));
#95341=CARTESIAN_POINT('Ctrl Pts',(111.854519046967,21.4574771160738,31.));
#95342=CARTESIAN_POINT('Ctrl Pts',(111.854519046967,21.4574771160738,26.));
#95343=CARTESIAN_POINT('Ctrl Pts',(111.849412603975,21.4340592952752,31.));
#95344=CARTESIAN_POINT('Ctrl Pts',(111.849412603975,21.4340592952752,26.));
#95345=CARTESIAN_POINT('Ctrl Pts',(111.844021598965,21.4116645975774,31.));
#95346=CARTESIAN_POINT('Ctrl Pts',(111.844021598965,21.4116645975774,26.));
#95347=CARTESIAN_POINT('Ctrl Pts',(111.838434156637,21.3904834307551,31.));
#95348=CARTESIAN_POINT('Ctrl Pts',(111.838434156637,21.3904834307551,26.));
#95349=CARTESIAN_POINT('Ctrl Pts',(111.832738794601,21.3707055346837,31.));
#95350=CARTESIAN_POINT('Ctrl Pts',(111.832738794601,21.3707055346837,26.));
#95351=CARTESIAN_POINT('Ctrl Pts',(111.827013583956,21.3524951721927,31.));
#95352=CARTESIAN_POINT('Ctrl Pts',(111.827013583956,21.3524951721927,26.));
#95353=CARTESIAN_POINT('Ctrl Pts',(111.821312902766,21.3359599004136,31.));
#95354=CARTESIAN_POINT('Ctrl Pts',(111.821312902766,21.3359599004136,26.));
#95355=CARTESIAN_POINT('Ctrl Pts',(111.815668148108,21.3211540061504,31.));
#95356=CARTESIAN_POINT('Ctrl Pts',(111.815668148108,21.3211540061504,26.));
#95357=CARTESIAN_POINT('Ctrl Pts',(111.811209579937,21.3107091062357,31.));
#95358=CARTESIAN_POINT('Ctrl Pts',(111.811209579937,21.3107091062357,26.));
#95359=CARTESIAN_POINT('Ctrl Pts',(111.807900012956,21.3036628730485,31.));
#95360=CARTESIAN_POINT('Ctrl Pts',(111.807900012956,21.3036628730485,26.));
#95361=CARTESIAN_POINT('Ctrl Pts',(111.805708883803,21.2993147395223,31.));
#95362=CARTESIAN_POINT('Ctrl Pts',(111.805708883803,21.2993147395223,26.));
#95363=CARTESIAN_POINT('Ctrl Pts',(111.804617131104,21.297228010781,31.));
#95364=CARTESIAN_POINT('Ctrl Pts',(111.804617131104,21.297228010781,26.));
#95365=CARTESIAN_POINT('',(111.854141622223,22.1002632652963,31.));
#95366=CARTESIAN_POINT('Ctrl Pts',(111.804617131104,21.297228010781,31.));
#95367=CARTESIAN_POINT('Ctrl Pts',(111.805708883803,21.2993147395223,31.));
#95368=CARTESIAN_POINT('Ctrl Pts',(111.807900012956,21.3036628730485,31.));
#95369=CARTESIAN_POINT('Ctrl Pts',(111.811209579937,21.3107091062357,31.));
#95370=CARTESIAN_POINT('Ctrl Pts',(111.815668148108,21.3211540061504,31.));
#95371=CARTESIAN_POINT('Ctrl Pts',(111.821312902766,21.3359599004136,31.));
#95372=CARTESIAN_POINT('Ctrl Pts',(111.827013583956,21.3524951721927,31.));
#95373=CARTESIAN_POINT('Ctrl Pts',(111.832738794601,21.3707055346837,31.));
#95374=CARTESIAN_POINT('Ctrl Pts',(111.838434156637,21.3904834307551,31.));
#95375=CARTESIAN_POINT('Ctrl Pts',(111.844021598965,21.4116645975774,31.));
#95376=CARTESIAN_POINT('Ctrl Pts',(111.849412603975,21.4340592952752,31.));
#95377=CARTESIAN_POINT('Ctrl Pts',(111.854519046967,21.4574771160738,31.));
#95378=CARTESIAN_POINT('Ctrl Pts',(111.859263936811,21.4817516412638,31.));
#95379=CARTESIAN_POINT('Ctrl Pts',(111.863594917346,21.5067708088162,31.));
#95380=CARTESIAN_POINT('Ctrl Pts',(111.867487146968,21.5324835838312,31.));
#95381=CARTESIAN_POINT('Ctrl Pts',(111.870932952965,21.5588771351418,31.));
#95382=CARTESIAN_POINT('Ctrl Pts',(111.873934841606,21.5859611128528,31.));
#95383=CARTESIAN_POINT('Ctrl Pts',(111.876497875355,21.6137504395647,31.));
#95384=CARTESIAN_POINT('Ctrl Pts',(111.878621136122,21.6422453942965,31.));
#95385=CARTESIAN_POINT('Ctrl Pts',(111.880294678138,21.6714250926009,31.));
#95386=CARTESIAN_POINT('Ctrl Pts',(111.881503038219,21.7012568937784,31.));
#95387=CARTESIAN_POINT('Ctrl Pts',(111.882227113875,21.7317015453702,31.));
#95388=CARTESIAN_POINT('Ctrl Pts',(111.88244665023,21.7627194836722,31.));
#95389=CARTESIAN_POINT('Ctrl Pts',(111.882142859804,21.7942773949803,31.));
#95390=CARTESIAN_POINT('Ctrl Pts',(111.881300030633,21.8263513619471,31.));
#95391=CARTESIAN_POINT('Ctrl Pts',(111.879905244522,21.858924151478,31.));
#95392=CARTESIAN_POINT('Ctrl Pts',(111.877948703413,21.8919838210589,31.));
#95393=CARTESIAN_POINT('Ctrl Pts',(111.875423885743,21.9255218058874,31.));
#95394=CARTESIAN_POINT('Ctrl Pts',(111.872328079755,21.9595309601143,31.));
#95395=CARTESIAN_POINT('Ctrl Pts',(111.868662421939,21.994004119741,31.));
#95396=CARTESIAN_POINT('Ctrl Pts',(111.864430146276,22.0289349711957,31.));
#95397=CARTESIAN_POINT('Ctrl Pts',(111.860594223066,22.0572417526884,31.));
#95398=CARTESIAN_POINT('Ctrl Pts',(111.85746561521,22.0786740240205,31.));
#95399=CARTESIAN_POINT('Ctrl Pts',(111.855268228011,22.0930519019996,31.));
#95400=CARTESIAN_POINT('Ctrl Pts',(111.854141622223,22.1002632652963,31.));
#95401=CARTESIAN_POINT('',(111.854141622223,22.1002632652963,26.));
#95402=CARTESIAN_POINT('Ctrl Pts',(111.854141622223,22.1002632652963,26.));
#95403=CARTESIAN_POINT('Ctrl Pts',(111.855268228011,22.0930519019996,26.));
#95404=CARTESIAN_POINT('Ctrl Pts',(111.85746561521,22.0786740240205,26.));
#95405=CARTESIAN_POINT('Ctrl Pts',(111.860594223066,22.0572417526884,26.));
#95406=CARTESIAN_POINT('Ctrl Pts',(111.864430146276,22.0289349711957,26.));
#95407=CARTESIAN_POINT('Ctrl Pts',(111.868662421939,21.994004119741,26.));
#95408=CARTESIAN_POINT('Ctrl Pts',(111.872328079755,21.9595309601143,26.));
#95409=CARTESIAN_POINT('Ctrl Pts',(111.875423885743,21.9255218058874,26.));
#95410=CARTESIAN_POINT('Ctrl Pts',(111.877948703413,21.8919838210589,26.));
#95411=CARTESIAN_POINT('Ctrl Pts',(111.879905244522,21.858924151478,26.));
#95412=CARTESIAN_POINT('Ctrl Pts',(111.881300030633,21.8263513619471,26.));
#95413=CARTESIAN_POINT('Ctrl Pts',(111.882142859804,21.7942773949803,26.));
#95414=CARTESIAN_POINT('Ctrl Pts',(111.88244665023,21.7627194836722,26.));
#95415=CARTESIAN_POINT('Ctrl Pts',(111.882227113875,21.7317015453702,26.));
#95416=CARTESIAN_POINT('Ctrl Pts',(111.881503038219,21.7012568937784,26.));
#95417=CARTESIAN_POINT('Ctrl Pts',(111.880294678138,21.6714250926009,26.));
#95418=CARTESIAN_POINT('Ctrl Pts',(111.878621136122,21.6422453942965,26.));
#95419=CARTESIAN_POINT('Ctrl Pts',(111.876497875355,21.6137504395647,26.));
#95420=CARTESIAN_POINT('Ctrl Pts',(111.873934841606,21.5859611128528,26.));
#95421=CARTESIAN_POINT('Ctrl Pts',(111.870932952965,21.5588771351418,26.));
#95422=CARTESIAN_POINT('Ctrl Pts',(111.867487146968,21.5324835838312,26.));
#95423=CARTESIAN_POINT('Ctrl Pts',(111.863594917346,21.5067708088162,26.));
#95424=CARTESIAN_POINT('Ctrl Pts',(111.859263936811,21.4817516412638,26.));
#95425=CARTESIAN_POINT('Ctrl Pts',(111.854519046967,21.4574771160738,26.));
#95426=CARTESIAN_POINT('Ctrl Pts',(111.849412603975,21.4340592952752,26.));
#95427=CARTESIAN_POINT('Ctrl Pts',(111.844021598965,21.4116645975774,26.));
#95428=CARTESIAN_POINT('Ctrl Pts',(111.838434156637,21.3904834307551,26.));
#95429=CARTESIAN_POINT('Ctrl Pts',(111.832738794601,21.3707055346837,26.));
#95430=CARTESIAN_POINT('Ctrl Pts',(111.827013583956,21.3524951721927,26.));
#95431=CARTESIAN_POINT('Ctrl Pts',(111.821312902766,21.3359599004136,26.));
#95432=CARTESIAN_POINT('Ctrl Pts',(111.815668148108,21.3211540061504,26.));
#95433=CARTESIAN_POINT('Ctrl Pts',(111.811209579937,21.3107091062357,26.));
#95434=CARTESIAN_POINT('Ctrl Pts',(111.807900012956,21.3036628730485,26.));
#95435=CARTESIAN_POINT('Ctrl Pts',(111.805708883803,21.2993147395223,26.));
#95436=CARTESIAN_POINT('Ctrl Pts',(111.804617131104,21.297228010781,26.));
#95437=CARTESIAN_POINT('',(111.854141622223,22.1002632652963,31.));
#95438=CARTESIAN_POINT('Origin',(109.999999999999,17.9999999999972,31.));
#95439=CARTESIAN_POINT('',(111.588247845187,22.2104000738956,31.));
#95440=CARTESIAN_POINT('Origin',(109.999999999999,17.9999999999972,31.));
#95441=CARTESIAN_POINT('',(111.588247845187,22.2104000738956,26.));
#95442=CARTESIAN_POINT('Origin',(109.999999999999,17.9999999999972,26.));
#95443=CARTESIAN_POINT('',(111.588247845187,22.2104000738956,31.));
#95444=CARTESIAN_POINT('Ctrl Pts',(111.055435274693,21.6075492963903,31.));
#95445=CARTESIAN_POINT('Ctrl Pts',(111.055435274693,21.6075492963903,26.));
#95446=CARTESIAN_POINT('Ctrl Pts',(111.056138828994,21.6097968221732,31.));
#95447=CARTESIAN_POINT('Ctrl Pts',(111.056138828994,21.6097968221732,26.));
#95448=CARTESIAN_POINT('Ctrl Pts',(111.057664061403,21.6144207791619,31.));
#95449=CARTESIAN_POINT('Ctrl Pts',(111.057664061403,21.6144207791619,26.));
#95450=CARTESIAN_POINT('Ctrl Pts',(111.060306283407,21.6217434356902,31.));
#95451=CARTESIAN_POINT('Ctrl Pts',(111.060306283407,21.6217434356902,26.));
#95452=CARTESIAN_POINT('Ctrl Pts',(111.064539259173,21.6322817790386,31.));
#95453=CARTESIAN_POINT('Ctrl Pts',(111.064539259173,21.6322817790386,26.));
#95454=CARTESIAN_POINT('Ctrl Pts',(111.071017163117,21.6467425715681,31.));
#95455=CARTESIAN_POINT('Ctrl Pts',(111.071017163117,21.6467425715681,26.));
#95456=CARTESIAN_POINT('Ctrl Pts',(111.078678375607,21.6624657646927,31.));
#95457=CARTESIAN_POINT('Ctrl Pts',(111.078678375607,21.6624657646927,26.));
#95458=CARTESIAN_POINT('Ctrl Pts',(111.087506711157,21.6793907707612,31.));
#95459=CARTESIAN_POINT('Ctrl Pts',(111.087506711157,21.6793907707612,26.));
#95460=CARTESIAN_POINT('Ctrl Pts',(111.097464566483,21.6974030843025,31.));
#95461=CARTESIAN_POINT('Ctrl Pts',(111.097464566483,21.6974030843025,26.));
#95462=CARTESIAN_POINT('Ctrl Pts',(111.108490994821,21.7163313493538,31.));
#95463=CARTESIAN_POINT('Ctrl Pts',(111.108490994821,21.7163313493538,26.));
#95464=CARTESIAN_POINT('Ctrl Pts',(111.120514421221,21.7359788081604,31.));
#95465=CARTESIAN_POINT('Ctrl Pts',(111.120514421221,21.7359788081604,26.));
#95466=CARTESIAN_POINT('Ctrl Pts',(111.13346252063,21.7561485085201,31.));
#95467=CARTESIAN_POINT('Ctrl Pts',(111.13346252063,21.7561485085201,26.));
#95468=CARTESIAN_POINT('Ctrl Pts',(111.147272058204,21.7766683336824,31.));
#95469=CARTESIAN_POINT('Ctrl Pts',(111.147272058204,21.7766683336824,26.));
#95470=CARTESIAN_POINT('Ctrl Pts',(111.161900815523,21.7974220224288,31.));
#95471=CARTESIAN_POINT('Ctrl Pts',(111.161900815523,21.7974220224288,26.));
#95472=CARTESIAN_POINT('Ctrl Pts',(111.177330271134,21.8183559219669,31.));
#95473=CARTESIAN_POINT('Ctrl Pts',(111.177330271134,21.8183559219669,26.));
#95474=CARTESIAN_POINT('Ctrl Pts',(111.19355677746,21.8394555338648,31.));
#95475=CARTESIAN_POINT('Ctrl Pts',(111.19355677746,21.8394555338648,26.));
#95476=CARTESIAN_POINT('Ctrl Pts',(111.210585385957,21.8607294539754,31.));
#95477=CARTESIAN_POINT('Ctrl Pts',(111.210585385957,21.8607294539754,26.));
#95478=CARTESIAN_POINT('Ctrl Pts',(111.228423068795,21.882191813874,31.));
#95479=CARTESIAN_POINT('Ctrl Pts',(111.228423068795,21.882191813874,26.));
#95480=CARTESIAN_POINT('Ctrl Pts',(111.247070672449,21.9038421616728,31.));
#95481=CARTESIAN_POINT('Ctrl Pts',(111.247070672449,21.9038421616728,26.));
#95482=CARTESIAN_POINT('Ctrl Pts',(111.266520462098,21.9256586971199,31.));
#95483=CARTESIAN_POINT('Ctrl Pts',(111.266520462098,21.9256586971199,26.));
#95484=CARTESIAN_POINT('Ctrl Pts',(111.286760291397,21.9476074056351,31.));
#95485=CARTESIAN_POINT('Ctrl Pts',(111.286760291397,21.9476074056351,26.));
#95486=CARTESIAN_POINT('Ctrl Pts',(111.307775912164,21.9696470240406,31.));
#95487=CARTESIAN_POINT('Ctrl Pts',(111.307775912164,21.9696470240406,26.));
#95488=CARTESIAN_POINT('Ctrl Pts',(111.329553670995,21.991735254212,31.));
#95489=CARTESIAN_POINT('Ctrl Pts',(111.329553670995,21.991735254212,26.));
#95490=CARTESIAN_POINT('Ctrl Pts',(111.352083296309,22.0138352550454,31.));
#95491=CARTESIAN_POINT('Ctrl Pts',(111.352083296309,22.0138352550454,26.));
#95492=CARTESIAN_POINT('Ctrl Pts',(111.375358986039,22.0359190043789,31.));
#95493=CARTESIAN_POINT('Ctrl Pts',(111.375358986039,22.0359190043789,26.));
#95494=CARTESIAN_POINT('Ctrl Pts',(111.39937768911,22.0579651820235,31.));
#95495=CARTESIAN_POINT('Ctrl Pts',(111.39937768911,22.0579651820235,26.));
#95496=CARTESIAN_POINT('Ctrl Pts',(111.424137889173,22.0799584150686,31.));
#95497=CARTESIAN_POINT('Ctrl Pts',(111.424137889173,22.0799584150686,26.));
#95498=CARTESIAN_POINT('Ctrl Pts',(111.449638141444,22.1018880358414,31.));
#95499=CARTESIAN_POINT('Ctrl Pts',(111.449638141444,22.1018880358414,26.));
#95500=CARTESIAN_POINT('Ctrl Pts',(111.475875310531,22.1237470739672,31.));
#95501=CARTESIAN_POINT('Ctrl Pts',(111.475875310531,22.1237470739672,26.));
#95502=CARTESIAN_POINT('Ctrl Pts',(111.502843527069,22.1455312673685,31.));
#95503=CARTESIAN_POINT('Ctrl Pts',(111.502843527069,22.1455312673685,26.));
#95504=CARTESIAN_POINT('Ctrl Pts',(111.530536039873,22.1672384384647,31.));
#95505=CARTESIAN_POINT('Ctrl Pts',(111.530536039873,22.1672384384647,26.));
#95506=CARTESIAN_POINT('Ctrl Pts',(111.553264364297,22.1845419483128,31.));
#95507=CARTESIAN_POINT('Ctrl Pts',(111.553264364297,22.1845419483128,26.));
#95508=CARTESIAN_POINT('Ctrl Pts',(111.570631528435,22.1974845929136,31.));
#95509=CARTESIAN_POINT('Ctrl Pts',(111.570631528435,22.1974845929136,26.));
#95510=CARTESIAN_POINT('Ctrl Pts',(111.582352010756,22.2060975005779,31.));
#95511=CARTESIAN_POINT('Ctrl Pts',(111.582352010756,22.2060975005779,26.));
#95512=CARTESIAN_POINT('Ctrl Pts',(111.588247845187,22.2104000738956,31.));
#95513=CARTESIAN_POINT('Ctrl Pts',(111.588247845187,22.2104000738956,26.));
#95514=CARTESIAN_POINT('Ctrl Pts',(111.055435274693,21.6075492963903,31.));
#95515=CARTESIAN_POINT('Ctrl Pts',(111.056138828994,21.6097968221732,31.));
#95516=CARTESIAN_POINT('Ctrl Pts',(111.057664061403,21.6144207791619,31.));
#95517=CARTESIAN_POINT('Ctrl Pts',(111.060306283407,21.6217434356902,31.));
#95518=CARTESIAN_POINT('Ctrl Pts',(111.064539259173,21.6322817790386,31.));
#95519=CARTESIAN_POINT('Ctrl Pts',(111.071017163117,21.6467425715681,31.));
#95520=CARTESIAN_POINT('Ctrl Pts',(111.078678375607,21.6624657646927,31.));
#95521=CARTESIAN_POINT('Ctrl Pts',(111.087506711157,21.6793907707612,31.));
#95522=CARTESIAN_POINT('Ctrl Pts',(111.097464566483,21.6974030843025,31.));
#95523=CARTESIAN_POINT('Ctrl Pts',(111.108490994821,21.7163313493538,31.));
#95524=CARTESIAN_POINT('Ctrl Pts',(111.120514421221,21.7359788081604,31.));
#95525=CARTESIAN_POINT('Ctrl Pts',(111.13346252063,21.7561485085201,31.));
#95526=CARTESIAN_POINT('Ctrl Pts',(111.147272058204,21.7766683336824,31.));
#95527=CARTESIAN_POINT('Ctrl Pts',(111.161900815523,21.7974220224288,31.));
#95528=CARTESIAN_POINT('Ctrl Pts',(111.177330271134,21.8183559219669,31.));
#95529=CARTESIAN_POINT('Ctrl Pts',(111.19355677746,21.8394555338648,31.));
#95530=CARTESIAN_POINT('Ctrl Pts',(111.210585385957,21.8607294539754,31.));
#95531=CARTESIAN_POINT('Ctrl Pts',(111.228423068795,21.882191813874,31.));
#95532=CARTESIAN_POINT('Ctrl Pts',(111.247070672449,21.9038421616728,31.));
#95533=CARTESIAN_POINT('Ctrl Pts',(111.266520462098,21.9256586971199,31.));
#95534=CARTESIAN_POINT('Ctrl Pts',(111.286760291397,21.9476074056351,31.));
#95535=CARTESIAN_POINT('Ctrl Pts',(111.307775912164,21.9696470240406,31.));
#95536=CARTESIAN_POINT('Ctrl Pts',(111.329553670995,21.991735254212,31.));
#95537=CARTESIAN_POINT('Ctrl Pts',(111.352083296309,22.0138352550454,31.));
#95538=CARTESIAN_POINT('Ctrl Pts',(111.375358986039,22.0359190043789,31.));
#95539=CARTESIAN_POINT('Ctrl Pts',(111.39937768911,22.0579651820235,31.));
#95540=CARTESIAN_POINT('Ctrl Pts',(111.424137889173,22.0799584150686,31.));
#95541=CARTESIAN_POINT('Ctrl Pts',(111.449638141444,22.1018880358414,31.));
#95542=CARTESIAN_POINT('Ctrl Pts',(111.475875310531,22.1237470739672,31.));
#95543=CARTESIAN_POINT('Ctrl Pts',(111.502843527069,22.1455312673685,31.));
#95544=CARTESIAN_POINT('Ctrl Pts',(111.530536039873,22.1672384384647,31.));
#95545=CARTESIAN_POINT('Ctrl Pts',(111.553264364297,22.1845419483128,31.));
#95546=CARTESIAN_POINT('Ctrl Pts',(111.570631528435,22.1974845929136,31.));
#95547=CARTESIAN_POINT('Ctrl Pts',(111.582352010756,22.2060975005779,31.));
#95548=CARTESIAN_POINT('Ctrl Pts',(111.588247845187,22.2104000738956,31.));
#95549=CARTESIAN_POINT('Ctrl Pts',(111.055435274693,21.6075492963903,26.));
#95550=CARTESIAN_POINT('Ctrl Pts',(111.056138828994,21.6097968221732,26.));
#95551=CARTESIAN_POINT('Ctrl Pts',(111.057664061403,21.6144207791619,26.));
#95552=CARTESIAN_POINT('Ctrl Pts',(111.060306283407,21.6217434356902,26.));
#95553=CARTESIAN_POINT('Ctrl Pts',(111.064539259173,21.6322817790386,26.));
#95554=CARTESIAN_POINT('Ctrl Pts',(111.071017163117,21.6467425715681,26.));
#95555=CARTESIAN_POINT('Ctrl Pts',(111.078678375607,21.6624657646927,26.));
#95556=CARTESIAN_POINT('Ctrl Pts',(111.087506711157,21.6793907707612,26.));
#95557=CARTESIAN_POINT('Ctrl Pts',(111.097464566483,21.6974030843025,26.));
#95558=CARTESIAN_POINT('Ctrl Pts',(111.108490994821,21.7163313493538,26.));
#95559=CARTESIAN_POINT('Ctrl Pts',(111.120514421221,21.7359788081604,26.));
#95560=CARTESIAN_POINT('Ctrl Pts',(111.13346252063,21.7561485085201,26.));
#95561=CARTESIAN_POINT('Ctrl Pts',(111.147272058204,21.7766683336824,26.));
#95562=CARTESIAN_POINT('Ctrl Pts',(111.161900815523,21.7974220224288,26.));
#95563=CARTESIAN_POINT('Ctrl Pts',(111.177330271134,21.8183559219669,26.));
#95564=CARTESIAN_POINT('Ctrl Pts',(111.19355677746,21.8394555338648,26.));
#95565=CARTESIAN_POINT('Ctrl Pts',(111.210585385957,21.8607294539754,26.));
#95566=CARTESIAN_POINT('Ctrl Pts',(111.228423068795,21.882191813874,26.));
#95567=CARTESIAN_POINT('Ctrl Pts',(111.247070672449,21.9038421616728,26.));
#95568=CARTESIAN_POINT('Ctrl Pts',(111.266520462098,21.9256586971199,26.));
#95569=CARTESIAN_POINT('Ctrl Pts',(111.286760291397,21.9476074056351,26.));
#95570=CARTESIAN_POINT('Ctrl Pts',(111.307775912164,21.9696470240406,26.));
#95571=CARTESIAN_POINT('Ctrl Pts',(111.329553670995,21.991735254212,26.));
#95572=CARTESIAN_POINT('Ctrl Pts',(111.352083296309,22.0138352550454,26.));
#95573=CARTESIAN_POINT('Ctrl Pts',(111.375358986039,22.0359190043789,26.));
#95574=CARTESIAN_POINT('Ctrl Pts',(111.39937768911,22.0579651820235,26.));
#95575=CARTESIAN_POINT('Ctrl Pts',(111.424137889173,22.0799584150686,26.));
#95576=CARTESIAN_POINT('Ctrl Pts',(111.449638141444,22.1018880358414,26.));
#95577=CARTESIAN_POINT('Ctrl Pts',(111.475875310531,22.1237470739672,26.));
#95578=CARTESIAN_POINT('Ctrl Pts',(111.502843527069,22.1455312673685,26.));
#95579=CARTESIAN_POINT('Ctrl Pts',(111.530536039873,22.1672384384647,26.));
#95580=CARTESIAN_POINT('Ctrl Pts',(111.553264364297,22.1845419483128,26.));
#95581=CARTESIAN_POINT('Ctrl Pts',(111.570631528435,22.1974845929136,26.));
#95582=CARTESIAN_POINT('Ctrl Pts',(111.582352010756,22.2060975005779,26.));
#95583=CARTESIAN_POINT('Ctrl Pts',(111.588247845187,22.2104000738956,26.));
#95584=CARTESIAN_POINT('Origin',(111.47451419404,21.5597921652037,31.));
#95585=CARTESIAN_POINT('Origin',(112.021127176843,20.5130996667515,31.));
#95586=CARTESIAN_POINT('',(112.355644395348,20.9290433639019,31.));
#95587=CARTESIAN_POINT('',(112.355644395348,20.9290433639019,31.));
#95588=CARTESIAN_POINT('',(112.355644395348,20.9290433639019,26.));
#95589=CARTESIAN_POINT('',(112.355644395348,20.9290433639019,31.));
#95590=CARTESIAN_POINT('',(112.355644395348,20.9290433639019,26.));
#95591=CARTESIAN_POINT('Origin',(112.929043363902,20.3556443953479,31.));
#95592=CARTESIAN_POINT('',(112.929043363902,20.3556443953479,26.));
#95593=CARTESIAN_POINT('',(112.513099666752,20.021127176843,26.));
#95594=CARTESIAN_POINT('',(112.929043363902,20.3556443953479,31.));
#95595=CARTESIAN_POINT('',(112.929043363902,20.3556443953479,31.));
#95596=CARTESIAN_POINT('',(112.513099666752,20.021127176843,31.));
#95597=CARTESIAN_POINT('Ctrl Pts',(113.282106315114,21.0786000286317,31.));
#95598=CARTESIAN_POINT('Ctrl Pts',(113.282106315114,21.0786000286317,26.));
#95599=CARTESIAN_POINT('Ctrl Pts',(113.280387493883,21.0715064643109,31.));
#95600=CARTESIAN_POINT('Ctrl Pts',(113.280387493883,21.0715064643109,26.));
#95601=CARTESIAN_POINT('Ctrl Pts',(113.276915439246,21.0573821334494,31.));
#95602=CARTESIAN_POINT('Ctrl Pts',(113.276915439246,21.0573821334494,26.));
#95603=CARTESIAN_POINT('Ctrl Pts',(113.271604120853,21.0363840302376,31.));
#95604=CARTESIAN_POINT('Ctrl Pts',(113.271604120853,21.0363840302376,26.));
#95605=CARTESIAN_POINT('Ctrl Pts',(113.264315515495,21.0087640299247,31.));
#95606=CARTESIAN_POINT('Ctrl Pts',(113.264315515495,21.0087640299247,26.));
#95607=CARTESIAN_POINT('Ctrl Pts',(113.254858170225,20.9748725094354,31.));
#95608=CARTESIAN_POINT('Ctrl Pts',(113.254858170225,20.9748725094354,26.));
#95609=CARTESIAN_POINT('Ctrl Pts',(113.245052489404,20.9416206763202,31.));
#95610=CARTESIAN_POINT('Ctrl Pts',(113.245052489404,20.9416206763202,26.));
#95611=CARTESIAN_POINT('Ctrl Pts',(113.234897901322,20.9090156011505,31.));
#95612=CARTESIAN_POINT('Ctrl Pts',(113.234897901322,20.9090156011505,26.));
#95613=CARTESIAN_POINT('Ctrl Pts',(113.224396097542,20.8770643375138,31.));
#95614=CARTESIAN_POINT('Ctrl Pts',(113.224396097542,20.8770643375138,26.));
#95615=CARTESIAN_POINT('Ctrl Pts',(113.213552317998,20.8457724495694,31.));
#95616=CARTESIAN_POINT('Ctrl Pts',(113.213552317998,20.8457724495694,26.));
#95617=CARTESIAN_POINT('Ctrl Pts',(113.20237586544,20.8151453544684,31.));
#95618=CARTESIAN_POINT('Ctrl Pts',(113.20237586544,20.8151453544684,26.));
#95619=CARTESIAN_POINT('Ctrl Pts',(113.190880362291,20.7851903361014,31.));
#95620=CARTESIAN_POINT('Ctrl Pts',(113.190880362291,20.7851903361014,26.));
#95621=CARTESIAN_POINT('Ctrl Pts',(113.179084338231,20.755918372192,31.));
#95622=CARTESIAN_POINT('Ctrl Pts',(113.179084338231,20.755918372192,26.));
#95623=CARTESIAN_POINT('Ctrl Pts',(113.167011461991,20.7273455467799,31.));
#95624=CARTESIAN_POINT('Ctrl Pts',(113.167011461991,20.7273455467799,26.));
#95625=CARTESIAN_POINT('Ctrl Pts',(113.154691839545,20.6994954480571,31.));
#95626=CARTESIAN_POINT('Ctrl Pts',(113.154691839545,20.6994954480571,26.));
#95627=CARTESIAN_POINT('Ctrl Pts',(113.14215932433,20.6723968769145,31.));
#95628=CARTESIAN_POINT('Ctrl Pts',(113.14215932433,20.6723968769145,26.));
#95629=CARTESIAN_POINT('Ctrl Pts',(113.129446586011,20.6460787876893,31.));
#95630=CARTESIAN_POINT('Ctrl Pts',(113.129446586011,20.6460787876893,26.));
#95631=CARTESIAN_POINT('Ctrl Pts',(113.116580401765,20.620565418951,31.));
#95632=CARTESIAN_POINT('Ctrl Pts',(113.116580401765,20.620565418951,26.));
#95633=CARTESIAN_POINT('Ctrl Pts',(113.103577952414,20.5958722593316,31.));
#95634=CARTESIAN_POINT('Ctrl Pts',(113.103577952414,20.5958722593316,26.));
#95635=CARTESIAN_POINT('Ctrl Pts',(113.090439979387,20.5719986997143,31.));
#95636=CARTESIAN_POINT('Ctrl Pts',(113.090439979387,20.5719986997143,26.));
#95637=CARTESIAN_POINT('Ctrl Pts',(113.077156094945,20.5489328907344,31.));
#95638=CARTESIAN_POINT('Ctrl Pts',(113.077156094945,20.5489328907344,26.));
#95639=CARTESIAN_POINT('Ctrl Pts',(113.063720290664,20.5266668759651,31.));
#95640=CARTESIAN_POINT('Ctrl Pts',(113.063720290664,20.5266668759651,26.));
#95641=CARTESIAN_POINT('Ctrl Pts',(113.050144565478,20.5052095736397,31.));
#95642=CARTESIAN_POINT('Ctrl Pts',(113.050144565478,20.5052095736397,26.));
#95643=CARTESIAN_POINT('Ctrl Pts',(113.036471400248,20.4845986273869,31.));
#95644=CARTESIAN_POINT('Ctrl Pts',(113.036471400248,20.4845986273869,26.));
#95645=CARTESIAN_POINT('Ctrl Pts',(113.022792050042,20.4649175331864,31.));
#95646=CARTESIAN_POINT('Ctrl Pts',(113.022792050042,20.4649175331864,26.));
#95647=CARTESIAN_POINT('Ctrl Pts',(113.009241331072,20.4462905786477,31.));
#95648=CARTESIAN_POINT('Ctrl Pts',(113.009241331072,20.4462905786477,26.));
#95649=CARTESIAN_POINT('Ctrl Pts',(112.995973525845,20.4288599537543,31.));
#95650=CARTESIAN_POINT('Ctrl Pts',(112.995973525845,20.4288599537543,26.));
#95651=CARTESIAN_POINT('Ctrl Pts',(112.983143024276,20.4127670810703,31.));
#95652=CARTESIAN_POINT('Ctrl Pts',(112.983143024276,20.4127670810703,26.));
#95653=CARTESIAN_POINT('Ctrl Pts',(112.970884815319,20.3981338431457,31.));
#95654=CARTESIAN_POINT('Ctrl Pts',(112.970884815319,20.3981338431457,26.));
#95655=CARTESIAN_POINT('Ctrl Pts',(112.959290298087,20.3850388002292,31.));
#95656=CARTESIAN_POINT('Ctrl Pts',(112.959290298087,20.3850388002292,26.));
#95657=CARTESIAN_POINT('Ctrl Pts',(112.948409254356,20.3735200916464,31.));
#95658=CARTESIAN_POINT('Ctrl Pts',(112.948409254356,20.3735200916464,26.));
#95659=CARTESIAN_POINT('Ctrl Pts',(112.940292984329,20.3655764825671,31.));
#95660=CARTESIAN_POINT('Ctrl Pts',(112.940292984329,20.3655764825671,26.));
#95661=CARTESIAN_POINT('Ctrl Pts',(112.934538866432,20.3603331283963,31.));
#95662=CARTESIAN_POINT('Ctrl Pts',(112.934538866432,20.3603331283963,26.));
#95663=CARTESIAN_POINT('Ctrl Pts',(112.930850568392,20.3571544856518,31.));
#95664=CARTESIAN_POINT('Ctrl Pts',(112.930850568392,20.3571544856518,26.));
#95665=CARTESIAN_POINT('Ctrl Pts',(112.929043363902,20.3556443953479,31.));
#95666=CARTESIAN_POINT('Ctrl Pts',(112.929043363902,20.3556443953479,26.));
#95667=CARTESIAN_POINT('',(113.282106315114,21.0786000286317,31.));
#95668=CARTESIAN_POINT('Ctrl Pts',(112.929043363902,20.3556443953479,31.));
#95669=CARTESIAN_POINT('Ctrl Pts',(112.930850568392,20.3571544856518,31.));
#95670=CARTESIAN_POINT('Ctrl Pts',(112.934538866432,20.3603331283963,31.));
#95671=CARTESIAN_POINT('Ctrl Pts',(112.940292984329,20.3655764825671,31.));
#95672=CARTESIAN_POINT('Ctrl Pts',(112.948409254356,20.3735200916464,31.));
#95673=CARTESIAN_POINT('Ctrl Pts',(112.959290298087,20.3850388002292,31.));
#95674=CARTESIAN_POINT('Ctrl Pts',(112.970884815319,20.3981338431457,31.));
#95675=CARTESIAN_POINT('Ctrl Pts',(112.983143024276,20.4127670810703,31.));
#95676=CARTESIAN_POINT('Ctrl Pts',(112.995973525845,20.4288599537543,31.));
#95677=CARTESIAN_POINT('Ctrl Pts',(113.009241331072,20.4462905786477,31.));
#95678=CARTESIAN_POINT('Ctrl Pts',(113.022792050042,20.4649175331864,31.));
#95679=CARTESIAN_POINT('Ctrl Pts',(113.036471400248,20.4845986273869,31.));
#95680=CARTESIAN_POINT('Ctrl Pts',(113.050144565478,20.5052095736397,31.));
#95681=CARTESIAN_POINT('Ctrl Pts',(113.063720290664,20.5266668759651,31.));
#95682=CARTESIAN_POINT('Ctrl Pts',(113.077156094945,20.5489328907344,31.));
#95683=CARTESIAN_POINT('Ctrl Pts',(113.090439979387,20.5719986997143,31.));
#95684=CARTESIAN_POINT('Ctrl Pts',(113.103577952414,20.5958722593316,31.));
#95685=CARTESIAN_POINT('Ctrl Pts',(113.116580401765,20.620565418951,31.));
#95686=CARTESIAN_POINT('Ctrl Pts',(113.129446586011,20.6460787876893,31.));
#95687=CARTESIAN_POINT('Ctrl Pts',(113.14215932433,20.6723968769145,31.));
#95688=CARTESIAN_POINT('Ctrl Pts',(113.154691839545,20.6994954480571,31.));
#95689=CARTESIAN_POINT('Ctrl Pts',(113.167011461991,20.7273455467799,31.));
#95690=CARTESIAN_POINT('Ctrl Pts',(113.179084338231,20.755918372192,31.));
#95691=CARTESIAN_POINT('Ctrl Pts',(113.190880362291,20.7851903361014,31.));
#95692=CARTESIAN_POINT('Ctrl Pts',(113.20237586544,20.8151453544684,31.));
#95693=CARTESIAN_POINT('Ctrl Pts',(113.213552317998,20.8457724495694,31.));
#95694=CARTESIAN_POINT('Ctrl Pts',(113.224396097542,20.8770643375138,31.));
#95695=CARTESIAN_POINT('Ctrl Pts',(113.234897901322,20.9090156011505,31.));
#95696=CARTESIAN_POINT('Ctrl Pts',(113.245052489404,20.9416206763202,31.));
#95697=CARTESIAN_POINT('Ctrl Pts',(113.254858170225,20.9748725094354,31.));
#95698=CARTESIAN_POINT('Ctrl Pts',(113.264315515495,21.0087640299247,31.));
#95699=CARTESIAN_POINT('Ctrl Pts',(113.271604120853,21.0363840302376,31.));
#95700=CARTESIAN_POINT('Ctrl Pts',(113.276915439246,21.0573821334494,31.));
#95701=CARTESIAN_POINT('Ctrl Pts',(113.280387493883,21.0715064643109,31.));
#95702=CARTESIAN_POINT('Ctrl Pts',(113.282106315114,21.0786000286317,31.));
#95703=CARTESIAN_POINT('',(113.282106315114,21.0786000286317,26.));
#95704=CARTESIAN_POINT('Ctrl Pts',(113.282106315114,21.0786000286317,26.));
#95705=CARTESIAN_POINT('Ctrl Pts',(113.280387493883,21.0715064643109,26.));
#95706=CARTESIAN_POINT('Ctrl Pts',(113.276915439246,21.0573821334494,26.));
#95707=CARTESIAN_POINT('Ctrl Pts',(113.271604120853,21.0363840302376,26.));
#95708=CARTESIAN_POINT('Ctrl Pts',(113.264315515495,21.0087640299247,26.));
#95709=CARTESIAN_POINT('Ctrl Pts',(113.254858170225,20.9748725094354,26.));
#95710=CARTESIAN_POINT('Ctrl Pts',(113.245052489404,20.9416206763202,26.));
#95711=CARTESIAN_POINT('Ctrl Pts',(113.234897901322,20.9090156011505,26.));
#95712=CARTESIAN_POINT('Ctrl Pts',(113.224396097542,20.8770643375138,26.));
#95713=CARTESIAN_POINT('Ctrl Pts',(113.213552317998,20.8457724495694,26.));
#95714=CARTESIAN_POINT('Ctrl Pts',(113.20237586544,20.8151453544684,26.));
#95715=CARTESIAN_POINT('Ctrl Pts',(113.190880362291,20.7851903361014,26.));
#95716=CARTESIAN_POINT('Ctrl Pts',(113.179084338231,20.755918372192,26.));
#95717=CARTESIAN_POINT('Ctrl Pts',(113.167011461991,20.7273455467799,26.));
#95718=CARTESIAN_POINT('Ctrl Pts',(113.154691839545,20.6994954480571,26.));
#95719=CARTESIAN_POINT('Ctrl Pts',(113.14215932433,20.6723968769145,26.));
#95720=CARTESIAN_POINT('Ctrl Pts',(113.129446586011,20.6460787876893,26.));
#95721=CARTESIAN_POINT('Ctrl Pts',(113.116580401765,20.620565418951,26.));
#95722=CARTESIAN_POINT('Ctrl Pts',(113.103577952414,20.5958722593316,26.));
#95723=CARTESIAN_POINT('Ctrl Pts',(113.090439979387,20.5719986997143,26.));
#95724=CARTESIAN_POINT('Ctrl Pts',(113.077156094945,20.5489328907344,26.));
#95725=CARTESIAN_POINT('Ctrl Pts',(113.063720290664,20.5266668759651,26.));
#95726=CARTESIAN_POINT('Ctrl Pts',(113.050144565478,20.5052095736397,26.));
#95727=CARTESIAN_POINT('Ctrl Pts',(113.036471400248,20.4845986273869,26.));
#95728=CARTESIAN_POINT('Ctrl Pts',(113.022792050042,20.4649175331864,26.));
#95729=CARTESIAN_POINT('Ctrl Pts',(113.009241331072,20.4462905786477,26.));
#95730=CARTESIAN_POINT('Ctrl Pts',(112.995973525845,20.4288599537543,26.));
#95731=CARTESIAN_POINT('Ctrl Pts',(112.983143024276,20.4127670810703,26.));
#95732=CARTESIAN_POINT('Ctrl Pts',(112.970884815319,20.3981338431457,26.));
#95733=CARTESIAN_POINT('Ctrl Pts',(112.959290298087,20.3850388002292,26.));
#95734=CARTESIAN_POINT('Ctrl Pts',(112.948409254356,20.3735200916464,26.));
#95735=CARTESIAN_POINT('Ctrl Pts',(112.940292984329,20.3655764825671,26.));
#95736=CARTESIAN_POINT('Ctrl Pts',(112.934538866432,20.3603331283963,26.));
#95737=CARTESIAN_POINT('Ctrl Pts',(112.930850568392,20.3571544856518,26.));
#95738=CARTESIAN_POINT('Ctrl Pts',(112.929043363902,20.3556443953479,26.));
#95739=CARTESIAN_POINT('',(113.282106315114,21.0786000286317,31.));
#95740=CARTESIAN_POINT('Origin',(109.999999999998,17.9999999999978,31.));
#95741=CARTESIAN_POINT('',(113.078600028632,21.2821063151136,31.));
#95742=CARTESIAN_POINT('Origin',(109.999999999998,17.9999999999978,31.));
#95743=CARTESIAN_POINT('',(113.078600028632,21.2821063151136,26.));
#95744=CARTESIAN_POINT('Origin',(109.999999999998,17.9999999999978,26.));
#95745=CARTESIAN_POINT('',(113.078600028632,21.2821063151136,31.));
#95746=CARTESIAN_POINT('Ctrl Pts',(112.355644395348,20.9290433639019,31.));
#95747=CARTESIAN_POINT('Ctrl Pts',(112.355644395348,20.9290433639019,26.));
#95748=CARTESIAN_POINT('Ctrl Pts',(112.357154485648,20.9308505683967,31.));
#95749=CARTESIAN_POINT('Ctrl Pts',(112.357154485648,20.9308505683967,26.));
#95750=CARTESIAN_POINT('Ctrl Pts',(112.360333128385,20.9345388664441,31.));
#95751=CARTESIAN_POINT('Ctrl Pts',(112.360333128385,20.9345388664441,26.));
#95752=CARTESIAN_POINT('Ctrl Pts',(112.365576482549,20.9402929843488,31.));
#95753=CARTESIAN_POINT('Ctrl Pts',(112.365576482549,20.9402929843488,26.));
#95754=CARTESIAN_POINT('Ctrl Pts',(112.373520091625,20.9484092543796,31.));
#95755=CARTESIAN_POINT('Ctrl Pts',(112.373520091625,20.9484092543796,26.));
#95756=CARTESIAN_POINT('Ctrl Pts',(112.385038800212,20.9592902981059,31.));
#95757=CARTESIAN_POINT('Ctrl Pts',(112.385038800212,20.9592902981059,26.));
#95758=CARTESIAN_POINT('Ctrl Pts',(112.398133843138,20.9708848153277,31.));
#95759=CARTESIAN_POINT('Ctrl Pts',(112.398133843138,20.9708848153277,26.));
#95760=CARTESIAN_POINT('Ctrl Pts',(112.412767081074,20.9831430242715,31.));
#95761=CARTESIAN_POINT('Ctrl Pts',(112.412767081074,20.9831430242715,26.));
#95762=CARTESIAN_POINT('Ctrl Pts',(112.428859953768,20.9959735258305,31.));
#95763=CARTESIAN_POINT('Ctrl Pts',(112.428859953768,20.9959735258305,26.));
#95764=CARTESIAN_POINT('Ctrl Pts',(112.446290578665,21.0092413310541,31.));
#95765=CARTESIAN_POINT('Ctrl Pts',(112.446290578665,21.0092413310541,26.));
#95766=CARTESIAN_POINT('Ctrl Pts',(112.4649175332,21.0227920500277,31.));
#95767=CARTESIAN_POINT('Ctrl Pts',(112.4649175332,21.0227920500277,26.));
#95768=CARTESIAN_POINT('Ctrl Pts',(112.484598627392,21.0364714002426,31.));
#95769=CARTESIAN_POINT('Ctrl Pts',(112.484598627392,21.0364714002426,26.));
#95770=CARTESIAN_POINT('Ctrl Pts',(112.505209573635,21.0501445654825,31.));
#95771=CARTESIAN_POINT('Ctrl Pts',(112.505209573635,21.0501445654825,26.));
#95772=CARTESIAN_POINT('Ctrl Pts',(112.526666875952,21.0637202906774,31.));
#95773=CARTESIAN_POINT('Ctrl Pts',(112.526666875952,21.0637202906774,26.));
#95774=CARTESIAN_POINT('Ctrl Pts',(112.548932890716,21.0771560949637,31.));
#95775=CARTESIAN_POINT('Ctrl Pts',(112.548932890716,21.0771560949637,26.));
#95776=CARTESIAN_POINT('Ctrl Pts',(112.571998699698,21.0904399794041,31.));
#95777=CARTESIAN_POINT('Ctrl Pts',(112.571998699698,21.0904399794041,26.));
#95778=CARTESIAN_POINT('Ctrl Pts',(112.595872259324,21.1035779524222,31.));
#95779=CARTESIAN_POINT('Ctrl Pts',(112.595872259324,21.1035779524222,26.));
#95780=CARTESIAN_POINT('Ctrl Pts',(112.620565418957,21.1165804017582,31.));
#95781=CARTESIAN_POINT('Ctrl Pts',(112.620565418957,21.1165804017582,26.));
#95782=CARTESIAN_POINT('Ctrl Pts',(112.646078787711,21.1294465859895,31.));
#95783=CARTESIAN_POINT('Ctrl Pts',(112.646078787711,21.1294465859895,26.));
#95784=CARTESIAN_POINT('Ctrl Pts',(112.672396876946,21.1421593242979,31.));
#95785=CARTESIAN_POINT('Ctrl Pts',(112.672396876946,21.1421593242979,26.));
#95786=CARTESIAN_POINT('Ctrl Pts',(112.699495448089,21.1546918395131,31.));
#95787=CARTESIAN_POINT('Ctrl Pts',(112.699495448089,21.1546918395131,26.));
#95788=CARTESIAN_POINT('Ctrl Pts',(112.727345546797,21.1670114619741,31.));
#95789=CARTESIAN_POINT('Ctrl Pts',(112.727345546797,21.1670114619741,26.));
#95790=CARTESIAN_POINT('Ctrl Pts',(112.755918372182,21.1790843382401,31.));
#95791=CARTESIAN_POINT('Ctrl Pts',(112.755918372182,21.1790843382401,26.));
#95792=CARTESIAN_POINT('Ctrl Pts',(112.785190336059,21.1908803623338,31.));
#95793=CARTESIAN_POINT('Ctrl Pts',(112.785190336059,21.1908803623338,26.));
#95794=CARTESIAN_POINT('Ctrl Pts',(112.8151453544,21.2023758655074,31.));
#95795=CARTESIAN_POINT('Ctrl Pts',(112.8151453544,21.2023758655074,26.));
#95796=CARTESIAN_POINT('Ctrl Pts',(112.845772449496,21.2135523180713,31.));
#95797=CARTESIAN_POINT('Ctrl Pts',(112.845772449496,21.2135523180713,26.));
#95798=CARTESIAN_POINT('Ctrl Pts',(112.877064337466,21.2243960975892,31.));
#95799=CARTESIAN_POINT('Ctrl Pts',(112.877064337466,21.2243960975892,26.));
#95800=CARTESIAN_POINT('Ctrl Pts',(112.909015601161,21.2348979013117,31.));
#95801=CARTESIAN_POINT('Ctrl Pts',(112.909015601161,21.2348979013117,26.));
#95802=CARTESIAN_POINT('Ctrl Pts',(112.94162067641,21.2450524893146,31.));
#95803=CARTESIAN_POINT('Ctrl Pts',(112.94162067641,21.2450524893146,26.));
#95804=CARTESIAN_POINT('Ctrl Pts',(112.9748725096,21.2548581700607,31.));
#95805=CARTESIAN_POINT('Ctrl Pts',(112.9748725096,21.2548581700607,26.));
#95806=CARTESIAN_POINT('Ctrl Pts',(113.008764030125,21.2643155152947,31.));
#95807=CARTESIAN_POINT('Ctrl Pts',(113.008764030125,21.2643155152947,26.));
#95808=CARTESIAN_POINT('Ctrl Pts',(113.036384030409,21.2716041206815,31.));
#95809=CARTESIAN_POINT('Ctrl Pts',(113.036384030409,21.2716041206815,26.));
#95810=CARTESIAN_POINT('Ctrl Pts',(113.057382133554,21.2769154391419,31.));
#95811=CARTESIAN_POINT('Ctrl Pts',(113.057382133554,21.2769154391419,26.));
#95812=CARTESIAN_POINT('Ctrl Pts',(113.071506464349,21.2803874938447,31.));
#95813=CARTESIAN_POINT('Ctrl Pts',(113.071506464349,21.2803874938447,26.));
#95814=CARTESIAN_POINT('Ctrl Pts',(113.078600028632,21.2821063151136,31.));
#95815=CARTESIAN_POINT('Ctrl Pts',(113.078600028632,21.2821063151136,26.));
#95816=CARTESIAN_POINT('Ctrl Pts',(112.355644395348,20.9290433639019,31.));
#95817=CARTESIAN_POINT('Ctrl Pts',(112.357154485648,20.9308505683967,31.));
#95818=CARTESIAN_POINT('Ctrl Pts',(112.360333128385,20.9345388664441,31.));
#95819=CARTESIAN_POINT('Ctrl Pts',(112.365576482549,20.9402929843488,31.));
#95820=CARTESIAN_POINT('Ctrl Pts',(112.373520091625,20.9484092543796,31.));
#95821=CARTESIAN_POINT('Ctrl Pts',(112.385038800212,20.9592902981059,31.));
#95822=CARTESIAN_POINT('Ctrl Pts',(112.398133843138,20.9708848153277,31.));
#95823=CARTESIAN_POINT('Ctrl Pts',(112.412767081074,20.9831430242715,31.));
#95824=CARTESIAN_POINT('Ctrl Pts',(112.428859953768,20.9959735258305,31.));
#95825=CARTESIAN_POINT('Ctrl Pts',(112.446290578665,21.0092413310541,31.));
#95826=CARTESIAN_POINT('Ctrl Pts',(112.4649175332,21.0227920500277,31.));
#95827=CARTESIAN_POINT('Ctrl Pts',(112.484598627392,21.0364714002426,31.));
#95828=CARTESIAN_POINT('Ctrl Pts',(112.505209573635,21.0501445654825,31.));
#95829=CARTESIAN_POINT('Ctrl Pts',(112.526666875952,21.0637202906774,31.));
#95830=CARTESIAN_POINT('Ctrl Pts',(112.548932890716,21.0771560949637,31.));
#95831=CARTESIAN_POINT('Ctrl Pts',(112.571998699698,21.0904399794041,31.));
#95832=CARTESIAN_POINT('Ctrl Pts',(112.595872259324,21.1035779524222,31.));
#95833=CARTESIAN_POINT('Ctrl Pts',(112.620565418957,21.1165804017582,31.));
#95834=CARTESIAN_POINT('Ctrl Pts',(112.646078787711,21.1294465859895,31.));
#95835=CARTESIAN_POINT('Ctrl Pts',(112.672396876946,21.1421593242979,31.));
#95836=CARTESIAN_POINT('Ctrl Pts',(112.699495448089,21.1546918395131,31.));
#95837=CARTESIAN_POINT('Ctrl Pts',(112.727345546797,21.1670114619741,31.));
#95838=CARTESIAN_POINT('Ctrl Pts',(112.755918372182,21.1790843382401,31.));
#95839=CARTESIAN_POINT('Ctrl Pts',(112.785190336059,21.1908803623338,31.));
#95840=CARTESIAN_POINT('Ctrl Pts',(112.8151453544,21.2023758655074,31.));
#95841=CARTESIAN_POINT('Ctrl Pts',(112.845772449496,21.2135523180713,31.));
#95842=CARTESIAN_POINT('Ctrl Pts',(112.877064337466,21.2243960975892,31.));
#95843=CARTESIAN_POINT('Ctrl Pts',(112.909015601161,21.2348979013117,31.));
#95844=CARTESIAN_POINT('Ctrl Pts',(112.94162067641,21.2450524893146,31.));
#95845=CARTESIAN_POINT('Ctrl Pts',(112.9748725096,21.2548581700607,31.));
#95846=CARTESIAN_POINT('Ctrl Pts',(113.008764030125,21.2643155152947,31.));
#95847=CARTESIAN_POINT('Ctrl Pts',(113.036384030409,21.2716041206815,31.));
#95848=CARTESIAN_POINT('Ctrl Pts',(113.057382133554,21.2769154391419,31.));
#95849=CARTESIAN_POINT('Ctrl Pts',(113.071506464349,21.2803874938447,31.));
#95850=CARTESIAN_POINT('Ctrl Pts',(113.078600028632,21.2821063151136,31.));
#95851=CARTESIAN_POINT('Ctrl Pts',(112.355644395348,20.9290433639019,26.));
#95852=CARTESIAN_POINT('Ctrl Pts',(112.357154485648,20.9308505683967,26.));
#95853=CARTESIAN_POINT('Ctrl Pts',(112.360333128385,20.9345388664441,26.));
#95854=CARTESIAN_POINT('Ctrl Pts',(112.365576482549,20.9402929843488,26.));
#95855=CARTESIAN_POINT('Ctrl Pts',(112.373520091625,20.9484092543796,26.));
#95856=CARTESIAN_POINT('Ctrl Pts',(112.385038800212,20.9592902981059,26.));
#95857=CARTESIAN_POINT('Ctrl Pts',(112.398133843138,20.9708848153277,26.));
#95858=CARTESIAN_POINT('Ctrl Pts',(112.412767081074,20.9831430242715,26.));
#95859=CARTESIAN_POINT('Ctrl Pts',(112.428859953768,20.9959735258305,26.));
#95860=CARTESIAN_POINT('Ctrl Pts',(112.446290578665,21.0092413310541,26.));
#95861=CARTESIAN_POINT('Ctrl Pts',(112.4649175332,21.0227920500277,26.));
#95862=CARTESIAN_POINT('Ctrl Pts',(112.484598627392,21.0364714002426,26.));
#95863=CARTESIAN_POINT('Ctrl Pts',(112.505209573635,21.0501445654825,26.));
#95864=CARTESIAN_POINT('Ctrl Pts',(112.526666875952,21.0637202906774,26.));
#95865=CARTESIAN_POINT('Ctrl Pts',(112.548932890716,21.0771560949637,26.));
#95866=CARTESIAN_POINT('Ctrl Pts',(112.571998699698,21.0904399794041,26.));
#95867=CARTESIAN_POINT('Ctrl Pts',(112.595872259324,21.1035779524222,26.));
#95868=CARTESIAN_POINT('Ctrl Pts',(112.620565418957,21.1165804017582,26.));
#95869=CARTESIAN_POINT('Ctrl Pts',(112.646078787711,21.1294465859895,26.));
#95870=CARTESIAN_POINT('Ctrl Pts',(112.672396876946,21.1421593242979,26.));
#95871=CARTESIAN_POINT('Ctrl Pts',(112.699495448089,21.1546918395131,26.));
#95872=CARTESIAN_POINT('Ctrl Pts',(112.727345546797,21.1670114619741,26.));
#95873=CARTESIAN_POINT('Ctrl Pts',(112.755918372182,21.1790843382401,26.));
#95874=CARTESIAN_POINT('Ctrl Pts',(112.785190336059,21.1908803623338,26.));
#95875=CARTESIAN_POINT('Ctrl Pts',(112.8151453544,21.2023758655074,26.));
#95876=CARTESIAN_POINT('Ctrl Pts',(112.845772449496,21.2135523180713,26.));
#95877=CARTESIAN_POINT('Ctrl Pts',(112.877064337466,21.2243960975892,26.));
#95878=CARTESIAN_POINT('Ctrl Pts',(112.909015601161,21.2348979013117,26.));
#95879=CARTESIAN_POINT('Ctrl Pts',(112.94162067641,21.2450524893146,26.));
#95880=CARTESIAN_POINT('Ctrl Pts',(112.9748725096,21.2548581700607,26.));
#95881=CARTESIAN_POINT('Ctrl Pts',(113.008764030125,21.2643155152947,26.));
#95882=CARTESIAN_POINT('Ctrl Pts',(113.036384030409,21.2716041206815,26.));
#95883=CARTESIAN_POINT('Ctrl Pts',(113.057382133554,21.2769154391419,26.));
#95884=CARTESIAN_POINT('Ctrl Pts',(113.071506464349,21.2803874938447,26.));
#95885=CARTESIAN_POINT('Ctrl Pts',(113.078600028632,21.2821063151136,26.));
#95886=CARTESIAN_POINT('Origin',(112.724546968557,20.7245469685797,31.));
#95887=CARTESIAN_POINT('Origin',(112.828999637636,19.548349459992,31.));
#95888=CARTESIAN_POINT('',(113.297228010781,19.8046171311037,31.));
#95889=CARTESIAN_POINT('',(113.297228010781,19.8046171311037,31.));
#95890=CARTESIAN_POINT('',(113.297228010781,19.8046171311037,26.));
#95891=CARTESIAN_POINT('',(113.297228010781,19.8046171311037,31.));
#95892=CARTESIAN_POINT('',(113.297228010781,19.8046171311037,26.));
#95893=CARTESIAN_POINT('Origin',(113.60754929639,19.0554352746927,31.));
#95894=CARTESIAN_POINT('',(113.60754929639,19.0554352746927,26.));
#95895=CARTESIAN_POINT('',(113.095253230553,18.9055564249396,26.));
#95896=CARTESIAN_POINT('',(113.60754929639,19.0554352746927,31.));
#95897=CARTESIAN_POINT('',(113.60754929639,19.0554352746927,31.));
#95898=CARTESIAN_POINT('',(113.095253230553,18.9055564249396,31.));
#95899=CARTESIAN_POINT('Ctrl Pts',(114.210400073896,19.5882478451867,31.));
#95900=CARTESIAN_POINT('Ctrl Pts',(114.210400073896,19.5882478451867,26.));
#95901=CARTESIAN_POINT('Ctrl Pts',(114.206097500599,19.5823520107063,31.));
#95902=CARTESIAN_POINT('Ctrl Pts',(114.206097500599,19.5823520107063,26.));
#95903=CARTESIAN_POINT('Ctrl Pts',(114.19748459297,19.5706315282987,31.));
#95904=CARTESIAN_POINT('Ctrl Pts',(114.19748459297,19.5706315282987,26.));
#95905=CARTESIAN_POINT('Ctrl Pts',(114.184541948405,19.5532643640729,31.));
#95906=CARTESIAN_POINT('Ctrl Pts',(114.184541948405,19.5532643640729,26.));
#95907=CARTESIAN_POINT('Ctrl Pts',(114.167238438573,19.5305360396115,31.));
#95908=CARTESIAN_POINT('Ctrl Pts',(114.167238438573,19.5305360396115,26.));
#95909=CARTESIAN_POINT('Ctrl Pts',(114.145531267457,19.5028435268547,31.));
#95910=CARTESIAN_POINT('Ctrl Pts',(114.145531267457,19.5028435268547,26.));
#95911=CARTESIAN_POINT('Ctrl Pts',(114.123747074016,19.4758753104142,31.));
#95912=CARTESIAN_POINT('Ctrl Pts',(114.123747074016,19.4758753104142,26.));
#95913=CARTESIAN_POINT('Ctrl Pts',(114.101888035847,19.4496381414305,31.));
#95914=CARTESIAN_POINT('Ctrl Pts',(114.101888035847,19.4496381414305,26.));
#95915=CARTESIAN_POINT('Ctrl Pts',(114.079958415043,19.4241378892353,31.));
#95916=CARTESIAN_POINT('Ctrl Pts',(114.079958415043,19.4241378892353,26.));
#95917=CARTESIAN_POINT('Ctrl Pts',(114.057965181984,19.3993776892053,31.));
#95918=CARTESIAN_POINT('Ctrl Pts',(114.057965181984,19.3993776892053,26.));
#95919=CARTESIAN_POINT('Ctrl Pts',(114.035919004342,19.3753589861281,31.));
#95920=CARTESIAN_POINT('Ctrl Pts',(114.035919004342,19.3753589861281,26.));
#95921=CARTESIAN_POINT('Ctrl Pts',(114.013835255023,19.3520832963642,31.));
#95922=CARTESIAN_POINT('Ctrl Pts',(114.013835255023,19.3520832963642,26.));
#95923=CARTESIAN_POINT('Ctrl Pts',(113.991735254207,19.3295536710079,31.));
#95924=CARTESIAN_POINT('Ctrl Pts',(113.991735254207,19.3295536710079,26.));
#95925=CARTESIAN_POINT('Ctrl Pts',(113.96964702405,19.3077759121412,31.));
#95926=CARTESIAN_POINT('Ctrl Pts',(113.96964702405,19.3077759121412,26.));
#95927=CARTESIAN_POINT('Ctrl Pts',(113.947607405652,19.2867602913563,31.));
#95928=CARTESIAN_POINT('Ctrl Pts',(113.947607405652,19.2867602913563,26.));
#95929=CARTESIAN_POINT('Ctrl Pts',(113.925658697137,19.266520462056,31.));
#95930=CARTESIAN_POINT('Ctrl Pts',(113.925658697137,19.266520462056,26.));
#95931=CARTESIAN_POINT('Ctrl Pts',(113.903842161685,19.2470706724204,31.));
#95932=CARTESIAN_POINT('Ctrl Pts',(113.903842161685,19.2470706724204,26.));
#95933=CARTESIAN_POINT('Ctrl Pts',(113.882191813877,19.2284230687867,31.));
#95934=CARTESIAN_POINT('Ctrl Pts',(113.882191813877,19.2284230687867,26.));
#95935=CARTESIAN_POINT('Ctrl Pts',(113.860729453971,19.2105853859678,31.));
#95936=CARTESIAN_POINT('Ctrl Pts',(113.860729453971,19.2105853859678,26.));
#95937=CARTESIAN_POINT('Ctrl Pts',(113.839455533856,19.1935567774815,31.));
#95938=CARTESIAN_POINT('Ctrl Pts',(113.839455533856,19.1935567774815,26.));
#95939=CARTESIAN_POINT('Ctrl Pts',(113.818355921957,19.1773302711575,31.));
#95940=CARTESIAN_POINT('Ctrl Pts',(113.818355921957,19.1773302711575,26.));
#95941=CARTESIAN_POINT('Ctrl Pts',(113.797422022421,19.1619008155406,31.));
#95942=CARTESIAN_POINT('Ctrl Pts',(113.797422022421,19.1619008155406,26.));
#95943=CARTESIAN_POINT('Ctrl Pts',(113.77666833368,19.1472720582102,31.));
#95944=CARTESIAN_POINT('Ctrl Pts',(113.77666833368,19.1472720582102,26.));
#95945=CARTESIAN_POINT('Ctrl Pts',(113.756148508523,19.133462520623,31.));
#95946=CARTESIAN_POINT('Ctrl Pts',(113.756148508523,19.133462520623,26.));
#95947=CARTESIAN_POINT('Ctrl Pts',(113.735978808168,19.1205144212031,31.));
#95948=CARTESIAN_POINT('Ctrl Pts',(113.735978808168,19.1205144212031,26.));
#95949=CARTESIAN_POINT('Ctrl Pts',(113.716331349364,19.1084909947982,31.));
#95950=CARTESIAN_POINT('Ctrl Pts',(113.716331349364,19.1084909947982,26.));
#95951=CARTESIAN_POINT('Ctrl Pts',(113.697403084311,19.0974645664646,31.));
#95952=CARTESIAN_POINT('Ctrl Pts',(113.697403084311,19.0974645664646,26.));
#95953=CARTESIAN_POINT('Ctrl Pts',(113.679390770764,19.087506711152,31.));
#95954=CARTESIAN_POINT('Ctrl Pts',(113.679390770764,19.087506711152,26.));
#95955=CARTESIAN_POINT('Ctrl Pts',(113.662465764688,19.0786783756173,31.));
#95956=CARTESIAN_POINT('Ctrl Pts',(113.662465764688,19.0786783756173,26.));
#95957=CARTESIAN_POINT('Ctrl Pts',(113.646742571557,19.0710171631404,31.));
#95958=CARTESIAN_POINT('Ctrl Pts',(113.646742571557,19.0710171631404,26.));
#95959=CARTESIAN_POINT('Ctrl Pts',(113.632281779025,19.0645392592025,31.));
#95960=CARTESIAN_POINT('Ctrl Pts',(113.632281779025,19.0645392592025,26.));
#95961=CARTESIAN_POINT('Ctrl Pts',(113.621743435679,19.0603062834318,31.));
#95962=CARTESIAN_POINT('Ctrl Pts',(113.621743435679,19.0603062834318,26.));
#95963=CARTESIAN_POINT('Ctrl Pts',(113.614420779155,19.0576640614188,31.));
#95964=CARTESIAN_POINT('Ctrl Pts',(113.614420779155,19.0576640614188,26.));
#95965=CARTESIAN_POINT('Ctrl Pts',(113.609796822171,19.0561388289994,31.));
#95966=CARTESIAN_POINT('Ctrl Pts',(113.609796822171,19.0561388289994,26.));
#95967=CARTESIAN_POINT('Ctrl Pts',(113.60754929639,19.0554352746927,31.));
#95968=CARTESIAN_POINT('Ctrl Pts',(113.60754929639,19.0554352746927,26.));
#95969=CARTESIAN_POINT('',(114.210400073896,19.5882478451867,31.));
#95970=CARTESIAN_POINT('Ctrl Pts',(113.60754929639,19.0554352746927,31.));
#95971=CARTESIAN_POINT('Ctrl Pts',(113.609796822171,19.0561388289994,31.));
#95972=CARTESIAN_POINT('Ctrl Pts',(113.614420779155,19.0576640614188,31.));
#95973=CARTESIAN_POINT('Ctrl Pts',(113.621743435679,19.0603062834318,31.));
#95974=CARTESIAN_POINT('Ctrl Pts',(113.632281779025,19.0645392592025,31.));
#95975=CARTESIAN_POINT('Ctrl Pts',(113.646742571557,19.0710171631404,31.));
#95976=CARTESIAN_POINT('Ctrl Pts',(113.662465764688,19.0786783756173,31.));
#95977=CARTESIAN_POINT('Ctrl Pts',(113.679390770764,19.087506711152,31.));
#95978=CARTESIAN_POINT('Ctrl Pts',(113.697403084311,19.0974645664646,31.));
#95979=CARTESIAN_POINT('Ctrl Pts',(113.716331349364,19.1084909947982,31.));
#95980=CARTESIAN_POINT('Ctrl Pts',(113.735978808168,19.1205144212031,31.));
#95981=CARTESIAN_POINT('Ctrl Pts',(113.756148508523,19.133462520623,31.));
#95982=CARTESIAN_POINT('Ctrl Pts',(113.77666833368,19.1472720582102,31.));
#95983=CARTESIAN_POINT('Ctrl Pts',(113.797422022421,19.1619008155406,31.));
#95984=CARTESIAN_POINT('Ctrl Pts',(113.818355921957,19.1773302711575,31.));
#95985=CARTESIAN_POINT('Ctrl Pts',(113.839455533856,19.1935567774815,31.));
#95986=CARTESIAN_POINT('Ctrl Pts',(113.860729453971,19.2105853859678,31.));
#95987=CARTESIAN_POINT('Ctrl Pts',(113.882191813877,19.2284230687867,31.));
#95988=CARTESIAN_POINT('Ctrl Pts',(113.903842161685,19.2470706724204,31.));
#95989=CARTESIAN_POINT('Ctrl Pts',(113.925658697137,19.266520462056,31.));
#95990=CARTESIAN_POINT('Ctrl Pts',(113.947607405652,19.2867602913563,31.));
#95991=CARTESIAN_POINT('Ctrl Pts',(113.96964702405,19.3077759121412,31.));
#95992=CARTESIAN_POINT('Ctrl Pts',(113.991735254207,19.3295536710079,31.));
#95993=CARTESIAN_POINT('Ctrl Pts',(114.013835255023,19.3520832963642,31.));
#95994=CARTESIAN_POINT('Ctrl Pts',(114.035919004342,19.3753589861281,31.));
#95995=CARTESIAN_POINT('Ctrl Pts',(114.057965181984,19.3993776892053,31.));
#95996=CARTESIAN_POINT('Ctrl Pts',(114.079958415043,19.4241378892353,31.));
#95997=CARTESIAN_POINT('Ctrl Pts',(114.101888035847,19.4496381414305,31.));
#95998=CARTESIAN_POINT('Ctrl Pts',(114.123747074016,19.4758753104142,31.));
#95999=CARTESIAN_POINT('Ctrl Pts',(114.145531267457,19.5028435268547,31.));
#96000=CARTESIAN_POINT('Ctrl Pts',(114.167238438573,19.5305360396115,31.));
#96001=CARTESIAN_POINT('Ctrl Pts',(114.184541948405,19.5532643640729,31.));
#96002=CARTESIAN_POINT('Ctrl Pts',(114.19748459297,19.5706315282987,31.));
#96003=CARTESIAN_POINT('Ctrl Pts',(114.206097500599,19.5823520107063,31.));
#96004=CARTESIAN_POINT('Ctrl Pts',(114.210400073896,19.5882478451867,31.));
#96005=CARTESIAN_POINT('',(114.210400073896,19.5882478451867,26.));
#96006=CARTESIAN_POINT('Ctrl Pts',(114.210400073896,19.5882478451867,26.));
#96007=CARTESIAN_POINT('Ctrl Pts',(114.206097500599,19.5823520107063,26.));
#96008=CARTESIAN_POINT('Ctrl Pts',(114.19748459297,19.5706315282987,26.));
#96009=CARTESIAN_POINT('Ctrl Pts',(114.184541948405,19.5532643640729,26.));
#96010=CARTESIAN_POINT('Ctrl Pts',(114.167238438573,19.5305360396115,26.));
#96011=CARTESIAN_POINT('Ctrl Pts',(114.145531267457,19.5028435268547,26.));
#96012=CARTESIAN_POINT('Ctrl Pts',(114.123747074016,19.4758753104142,26.));
#96013=CARTESIAN_POINT('Ctrl Pts',(114.101888035847,19.4496381414305,26.));
#96014=CARTESIAN_POINT('Ctrl Pts',(114.079958415043,19.4241378892353,26.));
#96015=CARTESIAN_POINT('Ctrl Pts',(114.057965181984,19.3993776892053,26.));
#96016=CARTESIAN_POINT('Ctrl Pts',(114.035919004342,19.3753589861281,26.));
#96017=CARTESIAN_POINT('Ctrl Pts',(114.013835255023,19.3520832963642,26.));
#96018=CARTESIAN_POINT('Ctrl Pts',(113.991735254207,19.3295536710079,26.));
#96019=CARTESIAN_POINT('Ctrl Pts',(113.96964702405,19.3077759121412,26.));
#96020=CARTESIAN_POINT('Ctrl Pts',(113.947607405652,19.2867602913563,26.));
#96021=CARTESIAN_POINT('Ctrl Pts',(113.925658697137,19.266520462056,26.));
#96022=CARTESIAN_POINT('Ctrl Pts',(113.903842161685,19.2470706724204,26.));
#96023=CARTESIAN_POINT('Ctrl Pts',(113.882191813877,19.2284230687867,26.));
#96024=CARTESIAN_POINT('Ctrl Pts',(113.860729453971,19.2105853859678,26.));
#96025=CARTESIAN_POINT('Ctrl Pts',(113.839455533856,19.1935567774815,26.));
#96026=CARTESIAN_POINT('Ctrl Pts',(113.818355921957,19.1773302711575,26.));
#96027=CARTESIAN_POINT('Ctrl Pts',(113.797422022421,19.1619008155406,26.));
#96028=CARTESIAN_POINT('Ctrl Pts',(113.77666833368,19.1472720582102,26.));
#96029=CARTESIAN_POINT('Ctrl Pts',(113.756148508523,19.133462520623,26.));
#96030=CARTESIAN_POINT('Ctrl Pts',(113.735978808168,19.1205144212031,26.));
#96031=CARTESIAN_POINT('Ctrl Pts',(113.716331349364,19.1084909947982,26.));
#96032=CARTESIAN_POINT('Ctrl Pts',(113.697403084311,19.0974645664646,26.));
#96033=CARTESIAN_POINT('Ctrl Pts',(113.679390770764,19.087506711152,26.));
#96034=CARTESIAN_POINT('Ctrl Pts',(113.662465764688,19.0786783756173,26.));
#96035=CARTESIAN_POINT('Ctrl Pts',(113.646742571557,19.0710171631404,26.));
#96036=CARTESIAN_POINT('Ctrl Pts',(113.632281779025,19.0645392592025,26.));
#96037=CARTESIAN_POINT('Ctrl Pts',(113.621743435679,19.0603062834318,26.));
#96038=CARTESIAN_POINT('Ctrl Pts',(113.614420779155,19.0576640614188,26.));
#96039=CARTESIAN_POINT('Ctrl Pts',(113.609796822171,19.0561388289994,26.));
#96040=CARTESIAN_POINT('Ctrl Pts',(113.60754929639,19.0554352746927,26.));
#96041=CARTESIAN_POINT('',(114.210400073896,19.5882478451867,31.));
#96042=CARTESIAN_POINT('Origin',(109.999999999997,17.9999999999988,31.));
#96043=CARTESIAN_POINT('',(114.100263265296,19.8541416222235,31.));
#96044=CARTESIAN_POINT('Origin',(109.999999999997,17.9999999999988,31.));
#96045=CARTESIAN_POINT('',(114.100263265296,19.8541416222235,26.));
#96046=CARTESIAN_POINT('Origin',(109.999999999997,17.9999999999988,26.));
#96047=CARTESIAN_POINT('',(114.100263265296,19.8541416222235,31.));
#96048=CARTESIAN_POINT('Ctrl Pts',(113.297228010781,19.8046171311037,31.));
#96049=CARTESIAN_POINT('Ctrl Pts',(113.297228010781,19.8046171311037,26.));
#96050=CARTESIAN_POINT('Ctrl Pts',(113.29931473952,19.8057088838085,31.));
#96051=CARTESIAN_POINT('Ctrl Pts',(113.29931473952,19.8057088838085,26.));
#96052=CARTESIAN_POINT('Ctrl Pts',(113.303662873043,19.8079000129713,31.));
#96053=CARTESIAN_POINT('Ctrl Pts',(113.303662873043,19.8079000129713,26.));
#96054=CARTESIAN_POINT('Ctrl Pts',(113.310709106226,19.8112095799625,31.));
#96055=CARTESIAN_POINT('Ctrl Pts',(113.310709106226,19.8112095799625,26.));
#96056=CARTESIAN_POINT('Ctrl Pts',(113.321154006139,19.8156681481377,31.));
#96057=CARTESIAN_POINT('Ctrl Pts',(113.321154006139,19.8156681481377,26.));
#96058=CARTESIAN_POINT('Ctrl Pts',(113.335959900405,19.8213129027904,31.));
#96059=CARTESIAN_POINT('Ctrl Pts',(113.335959900405,19.8213129027904,26.));
#96060=CARTESIAN_POINT('Ctrl Pts',(113.352495172189,19.8270135839669,31.));
#96061=CARTESIAN_POINT('Ctrl Pts',(113.352495172189,19.8270135839669,26.));
#96062=CARTESIAN_POINT('Ctrl Pts',(113.370705534686,19.8327387945953,31.));
#96063=CARTESIAN_POINT('Ctrl Pts',(113.370705534686,19.8327387945953,26.));
#96064=CARTESIAN_POINT('Ctrl Pts',(113.390483430762,19.8384341566185,31.));
#96065=CARTESIAN_POINT('Ctrl Pts',(113.390483430762,19.8384341566185,26.));
#96066=CARTESIAN_POINT('Ctrl Pts',(113.411664597586,19.8440215989421,31.));
#96067=CARTESIAN_POINT('Ctrl Pts',(113.411664597586,19.8440215989421,26.));
#96068=CARTESIAN_POINT('Ctrl Pts',(113.434059295282,19.8494126039565,31.));
#96069=CARTESIAN_POINT('Ctrl Pts',(113.434059295282,19.8494126039565,26.));
#96070=CARTESIAN_POINT('Ctrl Pts',(113.457477116077,19.8545190469599,31.));
#96071=CARTESIAN_POINT('Ctrl Pts',(113.457477116077,19.8545190469599,26.));
#96072=CARTESIAN_POINT('Ctrl Pts',(113.481751641261,19.8592639368172,31.));
#96073=CARTESIAN_POINT('Ctrl Pts',(113.481751641261,19.8592639368172,26.));
#96074=CARTESIAN_POINT('Ctrl Pts',(113.506770808809,19.863594917364,31.));
#96075=CARTESIAN_POINT('Ctrl Pts',(113.506770808809,19.863594917364,26.));
#96076=CARTESIAN_POINT('Ctrl Pts',(113.532483583821,19.8674871469917,31.));
#96077=CARTESIAN_POINT('Ctrl Pts',(113.532483583821,19.8674871469917,26.));
#96078=CARTESIAN_POINT('Ctrl Pts',(113.558877135133,19.8709329529872,31.));
#96079=CARTESIAN_POINT('Ctrl Pts',(113.558877135133,19.8709329529872,26.));
#96080=CARTESIAN_POINT('Ctrl Pts',(113.585961112848,19.8739348416169,31.));
#96081=CARTESIAN_POINT('Ctrl Pts',(113.585961112848,19.8739348416169,26.));
#96082=CARTESIAN_POINT('Ctrl Pts',(113.613750439568,19.8764978753463,31.));
#96083=CARTESIAN_POINT('Ctrl Pts',(113.613750439568,19.8764978753463,26.));
#96084=CARTESIAN_POINT('Ctrl Pts',(113.642245394308,19.8786211360933,31.));
#96085=CARTESIAN_POINT('Ctrl Pts',(113.642245394308,19.8786211360933,26.));
#96086=CARTESIAN_POINT('Ctrl Pts',(113.671425092618,19.8802946780967,31.));
#96087=CARTESIAN_POINT('Ctrl Pts',(113.671425092618,19.8802946780967,26.));
#96088=CARTESIAN_POINT('Ctrl Pts',(113.701256893795,19.8815030381781,31.));
#96089=CARTESIAN_POINT('Ctrl Pts',(113.701256893795,19.8815030381781,26.));
#96090=CARTESIAN_POINT('Ctrl Pts',(113.73170154538,19.8822271138526,31.));
#96091=CARTESIAN_POINT('Ctrl Pts',(113.73170154538,19.8822271138526,26.));
#96092=CARTESIAN_POINT('Ctrl Pts',(113.762719483667,19.8824466502425,31.));
#96093=CARTESIAN_POINT('Ctrl Pts',(113.762719483667,19.8824466502425,26.));
#96094=CARTESIAN_POINT('Ctrl Pts',(113.794277394957,19.8821428598593,31.));
#96095=CARTESIAN_POINT('Ctrl Pts',(113.794277394957,19.8821428598593,26.));
#96096=CARTESIAN_POINT('Ctrl Pts',(113.82635136191,19.8813000307218,31.));
#96097=CARTESIAN_POINT('Ctrl Pts',(113.82635136191,19.8813000307218,26.));
#96098=CARTESIAN_POINT('Ctrl Pts',(113.858924151438,19.8799052446171,31.));
#96099=CARTESIAN_POINT('Ctrl Pts',(113.858924151438,19.8799052446171,26.));
#96100=CARTESIAN_POINT('Ctrl Pts',(113.891983821033,19.8779487034752,31.));
#96101=CARTESIAN_POINT('Ctrl Pts',(113.891983821033,19.8779487034752,26.));
#96102=CARTESIAN_POINT('Ctrl Pts',(113.925521805893,19.8754238857298,31.));
#96103=CARTESIAN_POINT('Ctrl Pts',(113.925521805893,19.8754238857298,26.));
#96104=CARTESIAN_POINT('Ctrl Pts',(113.959530960163,19.8723280796379,31.));
#96105=CARTESIAN_POINT('Ctrl Pts',(113.959530960163,19.8723280796379,26.));
#96106=CARTESIAN_POINT('Ctrl Pts',(113.99400411983,19.868662421724,31.));
#96107=CARTESIAN_POINT('Ctrl Pts',(113.99400411983,19.868662421724,26.));
#96108=CARTESIAN_POINT('Ctrl Pts',(114.028934971304,19.8644301460149,31.));
#96109=CARTESIAN_POINT('Ctrl Pts',(114.028934971304,19.8644301460149,26.));
#96110=CARTESIAN_POINT('Ctrl Pts',(114.057241752781,19.8605942228417,31.));
#96111=CARTESIAN_POINT('Ctrl Pts',(114.057241752781,19.8605942228417,26.));
#96112=CARTESIAN_POINT('Ctrl Pts',(114.078674024077,19.8574656150733,31.));
#96113=CARTESIAN_POINT('Ctrl Pts',(114.078674024077,19.8574656150733,26.));
#96114=CARTESIAN_POINT('Ctrl Pts',(114.09305190202,19.8552682279604,31.));
#96115=CARTESIAN_POINT('Ctrl Pts',(114.09305190202,19.8552682279604,26.));
#96116=CARTESIAN_POINT('Ctrl Pts',(114.100263265296,19.8541416222235,31.));
#96117=CARTESIAN_POINT('Ctrl Pts',(114.100263265296,19.8541416222235,26.));
#96118=CARTESIAN_POINT('Ctrl Pts',(113.297228010781,19.8046171311037,31.));
#96119=CARTESIAN_POINT('Ctrl Pts',(113.29931473952,19.8057088838085,31.));
#96120=CARTESIAN_POINT('Ctrl Pts',(113.303662873043,19.8079000129713,31.));
#96121=CARTESIAN_POINT('Ctrl Pts',(113.310709106226,19.8112095799625,31.));
#96122=CARTESIAN_POINT('Ctrl Pts',(113.321154006139,19.8156681481377,31.));
#96123=CARTESIAN_POINT('Ctrl Pts',(113.335959900405,19.8213129027904,31.));
#96124=CARTESIAN_POINT('Ctrl Pts',(113.352495172189,19.8270135839669,31.));
#96125=CARTESIAN_POINT('Ctrl Pts',(113.370705534686,19.8327387945953,31.));
#96126=CARTESIAN_POINT('Ctrl Pts',(113.390483430762,19.8384341566185,31.));
#96127=CARTESIAN_POINT('Ctrl Pts',(113.411664597586,19.8440215989421,31.));
#96128=CARTESIAN_POINT('Ctrl Pts',(113.434059295282,19.8494126039565,31.));
#96129=CARTESIAN_POINT('Ctrl Pts',(113.457477116077,19.8545190469599,31.));
#96130=CARTESIAN_POINT('Ctrl Pts',(113.481751641261,19.8592639368172,31.));
#96131=CARTESIAN_POINT('Ctrl Pts',(113.506770808809,19.863594917364,31.));
#96132=CARTESIAN_POINT('Ctrl Pts',(113.532483583821,19.8674871469917,31.));
#96133=CARTESIAN_POINT('Ctrl Pts',(113.558877135133,19.8709329529872,31.));
#96134=CARTESIAN_POINT('Ctrl Pts',(113.585961112848,19.8739348416169,31.));
#96135=CARTESIAN_POINT('Ctrl Pts',(113.613750439568,19.8764978753463,31.));
#96136=CARTESIAN_POINT('Ctrl Pts',(113.642245394308,19.8786211360933,31.));
#96137=CARTESIAN_POINT('Ctrl Pts',(113.671425092618,19.8802946780967,31.));
#96138=CARTESIAN_POINT('Ctrl Pts',(113.701256893795,19.8815030381781,31.));
#96139=CARTESIAN_POINT('Ctrl Pts',(113.73170154538,19.8822271138526,31.));
#96140=CARTESIAN_POINT('Ctrl Pts',(113.762719483667,19.8824466502425,31.));
#96141=CARTESIAN_POINT('Ctrl Pts',(113.794277394957,19.8821428598593,31.));
#96142=CARTESIAN_POINT('Ctrl Pts',(113.82635136191,19.8813000307218,31.));
#96143=CARTESIAN_POINT('Ctrl Pts',(113.858924151438,19.8799052446171,31.));
#96144=CARTESIAN_POINT('Ctrl Pts',(113.891983821033,19.8779487034752,31.));
#96145=CARTESIAN_POINT('Ctrl Pts',(113.925521805893,19.8754238857298,31.));
#96146=CARTESIAN_POINT('Ctrl Pts',(113.959530960163,19.8723280796379,31.));
#96147=CARTESIAN_POINT('Ctrl Pts',(113.99400411983,19.868662421724,31.));
#96148=CARTESIAN_POINT('Ctrl Pts',(114.028934971304,19.8644301460149,31.));
#96149=CARTESIAN_POINT('Ctrl Pts',(114.057241752781,19.8605942228417,31.));
#96150=CARTESIAN_POINT('Ctrl Pts',(114.078674024077,19.8574656150733,31.));
#96151=CARTESIAN_POINT('Ctrl Pts',(114.09305190202,19.8552682279604,31.));
#96152=CARTESIAN_POINT('Ctrl Pts',(114.100263265296,19.8541416222235,31.));
#96153=CARTESIAN_POINT('Ctrl Pts',(113.297228010781,19.8046171311037,26.));
#96154=CARTESIAN_POINT('Ctrl Pts',(113.29931473952,19.8057088838085,26.));
#96155=CARTESIAN_POINT('Ctrl Pts',(113.303662873043,19.8079000129713,26.));
#96156=CARTESIAN_POINT('Ctrl Pts',(113.310709106226,19.8112095799625,26.));
#96157=CARTESIAN_POINT('Ctrl Pts',(113.321154006139,19.8156681481377,26.));
#96158=CARTESIAN_POINT('Ctrl Pts',(113.335959900405,19.8213129027904,26.));
#96159=CARTESIAN_POINT('Ctrl Pts',(113.352495172189,19.8270135839669,26.));
#96160=CARTESIAN_POINT('Ctrl Pts',(113.370705534686,19.8327387945953,26.));
#96161=CARTESIAN_POINT('Ctrl Pts',(113.390483430762,19.8384341566185,26.));
#96162=CARTESIAN_POINT('Ctrl Pts',(113.411664597586,19.8440215989421,26.));
#96163=CARTESIAN_POINT('Ctrl Pts',(113.434059295282,19.8494126039565,26.));
#96164=CARTESIAN_POINT('Ctrl Pts',(113.457477116077,19.8545190469599,26.));
#96165=CARTESIAN_POINT('Ctrl Pts',(113.481751641261,19.8592639368172,26.));
#96166=CARTESIAN_POINT('Ctrl Pts',(113.506770808809,19.863594917364,26.));
#96167=CARTESIAN_POINT('Ctrl Pts',(113.532483583821,19.8674871469917,26.));
#96168=CARTESIAN_POINT('Ctrl Pts',(113.558877135133,19.8709329529872,26.));
#96169=CARTESIAN_POINT('Ctrl Pts',(113.585961112848,19.8739348416169,26.));
#96170=CARTESIAN_POINT('Ctrl Pts',(113.613750439568,19.8764978753463,26.));
#96171=CARTESIAN_POINT('Ctrl Pts',(113.642245394308,19.8786211360933,26.));
#96172=CARTESIAN_POINT('Ctrl Pts',(113.671425092618,19.8802946780967,26.));
#96173=CARTESIAN_POINT('Ctrl Pts',(113.701256893795,19.8815030381781,26.));
#96174=CARTESIAN_POINT('Ctrl Pts',(113.73170154538,19.8822271138526,26.));
#96175=CARTESIAN_POINT('Ctrl Pts',(113.762719483667,19.8824466502425,26.));
#96176=CARTESIAN_POINT('Ctrl Pts',(113.794277394957,19.8821428598593,26.));
#96177=CARTESIAN_POINT('Ctrl Pts',(113.82635136191,19.8813000307218,26.));
#96178=CARTESIAN_POINT('Ctrl Pts',(113.858924151438,19.8799052446171,26.));
#96179=CARTESIAN_POINT('Ctrl Pts',(113.891983821033,19.8779487034752,26.));
#96180=CARTESIAN_POINT('Ctrl Pts',(113.925521805893,19.8754238857298,26.));
#96181=CARTESIAN_POINT('Ctrl Pts',(113.959530960163,19.8723280796379,26.));
#96182=CARTESIAN_POINT('Ctrl Pts',(113.99400411983,19.868662421724,26.));
#96183=CARTESIAN_POINT('Ctrl Pts',(114.028934971304,19.8644301460149,26.));
#96184=CARTESIAN_POINT('Ctrl Pts',(114.057241752781,19.8605942228417,26.));
#96185=CARTESIAN_POINT('Ctrl Pts',(114.078674024077,19.8574656150733,26.));
#96186=CARTESIAN_POINT('Ctrl Pts',(114.09305190202,19.8552682279604,26.));
#96187=CARTESIAN_POINT('Ctrl Pts',(114.100263265296,19.8541416222235,26.));
#96188=CARTESIAN_POINT('Origin',(113.559792165192,19.4745141940691,31.));
#96189=CARTESIAN_POINT('Origin',(113.206182548544,18.3478770837715,31.));
#96190=CARTESIAN_POINT('',(113.736838551019,18.4054542989899,31.));
#96191=CARTESIAN_POINT('',(113.736838551019,18.4054542989899,31.));
#96192=CARTESIAN_POINT('',(113.736838551019,18.4054542989899,26.));
#96193=CARTESIAN_POINT('',(113.736838551019,18.4054542989899,31.));
#96194=CARTESIAN_POINT('',(113.736838551019,18.4054542989899,26.));
#96195=CARTESIAN_POINT('Origin',(113.736838551019,17.5945457010101,31.));
#96196=CARTESIAN_POINT('',(113.736838551019,17.5945457010101,26.));
#96197=CARTESIAN_POINT('',(113.206182548544,17.6521229162285,26.));
#96198=CARTESIAN_POINT('',(113.736838551019,17.5945457010101,31.));
#96199=CARTESIAN_POINT('',(113.736838551019,17.5945457010101,31.));
#96200=CARTESIAN_POINT('',(113.206182548544,17.6521229162285,31.));
#96201=CARTESIAN_POINT('Ctrl Pts',(114.497698588799,17.8560993248145,31.));
#96202=CARTESIAN_POINT('Ctrl Pts',(114.497698588799,17.8560993248145,26.));
#96203=CARTESIAN_POINT('Ctrl Pts',(114.491467291217,17.8522988075283,31.));
#96204=CARTESIAN_POINT('Ctrl Pts',(114.491467291217,17.8522988075283,26.));
#96205=CARTESIAN_POINT('Ctrl Pts',(114.479024767707,17.8447665107748,31.));
#96206=CARTESIAN_POINT('Ctrl Pts',(114.479024767707,17.8447665107748,26.));
#96207=CARTESIAN_POINT('Ctrl Pts',(114.46042119728,17.8336742788547,31.));
#96208=CARTESIAN_POINT('Ctrl Pts',(114.46042119728,17.8336742788547,26.));
#96209=CARTESIAN_POINT('Ctrl Pts',(114.435737085489,17.8192978116112,31.));
#96210=CARTESIAN_POINT('Ctrl Pts',(114.435737085489,17.8192978116112,26.));
#96211=CARTESIAN_POINT('Ctrl Pts',(114.405084808554,17.8020202406208,31.));
#96212=CARTESIAN_POINT('Ctrl Pts',(114.405084808554,17.8020202406208,26.));
#96213=CARTESIAN_POINT('Ctrl Pts',(114.374638548468,17.7854413073407,31.));
#96214=CARTESIAN_POINT('Ctrl Pts',(114.374638548468,17.7854413073407,26.));
#96215=CARTESIAN_POINT('Ctrl Pts',(114.344402900622,17.7695664156801,31.));
#96216=CARTESIAN_POINT('Ctrl Pts',(114.344402900622,17.7695664156801,26.));
#96217=CARTESIAN_POINT('Ctrl Pts',(114.314384048769,17.7543993571629,31.));
#96218=CARTESIAN_POINT('Ctrl Pts',(114.314384048769,17.7543993571629,26.));
#96219=CARTESIAN_POINT('Ctrl Pts',(114.284589632559,17.73994036105,31.));
#96220=CARTESIAN_POINT('Ctrl Pts',(114.284589632559,17.73994036105,26.));
#96221=CARTESIAN_POINT('Ctrl Pts',(114.255030060531,17.72618667981,31.));
#96222=CARTESIAN_POINT('Ctrl Pts',(114.255030060531,17.72618667981,26.));
#96223=CARTESIAN_POINT('Ctrl Pts',(114.225720115684,17.7131338314213,31.));
#96224=CARTESIAN_POINT('Ctrl Pts',(114.225720115684,17.7131338314213,26.));
#96225=CARTESIAN_POINT('Ctrl Pts',(114.1966806629,17.7007764758468,31.));
#96226=CARTESIAN_POINT('Ctrl Pts',(114.1966806629,17.7007764758468,26.));
#96227=CARTESIAN_POINT('Ctrl Pts',(114.167939811637,17.6891092498973,31.));
#96228=CARTESIAN_POINT('Ctrl Pts',(114.167939811637,17.6891092498973,26.));
#96229=CARTESIAN_POINT('Ctrl Pts',(114.139535529399,17.6781275448076,31.));
#96230=CARTESIAN_POINT('Ctrl Pts',(114.139535529399,17.6781275448076,26.));
#96231=CARTESIAN_POINT('Ctrl Pts',(114.11151211949,17.667827787886,31.));
#96232=CARTESIAN_POINT('Ctrl Pts',(114.11151211949,17.667827787886,26.));
#96233=CARTESIAN_POINT('Ctrl Pts',(114.083913156659,17.6582073519993,31.));
#96234=CARTESIAN_POINT('Ctrl Pts',(114.083913156659,17.6582073519993,26.));
#96235=CARTESIAN_POINT('Ctrl Pts',(114.056774714484,17.6492644420825,31.));
#96236=CARTESIAN_POINT('Ctrl Pts',(114.056774714484,17.6492644420825,26.));
#96237=CARTESIAN_POINT('Ctrl Pts',(114.030119893761,17.6409978615743,31.));
#96238=CARTESIAN_POINT('Ctrl Pts',(114.030119893761,17.6409978615743,26.));
#96239=CARTESIAN_POINT('Ctrl Pts',(114.003948788046,17.6334066554963,31.));
#96240=CARTESIAN_POINT('Ctrl Pts',(114.003948788046,17.6334066554963,26.));
#96241=CARTESIAN_POINT('Ctrl Pts',(113.978245673333,17.6264897903224,31.));
#96242=CARTESIAN_POINT('Ctrl Pts',(113.978245673333,17.6264897903224,26.));
#96243=CARTESIAN_POINT('Ctrl Pts',(113.953000674982,17.6202458886071,31.));
#96244=CARTESIAN_POINT('Ctrl Pts',(113.953000674982,17.6202458886071,26.));
#96245=CARTESIAN_POINT('Ctrl Pts',(113.928228583663,17.6146727719654,31.));
#96246=CARTESIAN_POINT('Ctrl Pts',(113.928228583663,17.6146727719654,26.));
#96247=CARTESIAN_POINT('Ctrl Pts',(113.903986055947,17.6097670199576,31.));
#96248=CARTESIAN_POINT('Ctrl Pts',(113.903986055947,17.6097670199576,26.));
#96249=CARTESIAN_POINT('Ctrl Pts',(113.880396659483,17.6055231460801,31.));
#96250=CARTESIAN_POINT('Ctrl Pts',(113.880396659483,17.6055231460801,26.));
#96251=CARTESIAN_POINT('Ctrl Pts',(113.857643608343,17.6019337054866,31.));
#96252=CARTESIAN_POINT('Ctrl Pts',(113.857643608343,17.6019337054866,26.));
#96253=CARTESIAN_POINT('Ctrl Pts',(113.835936540232,17.5989901474718,31.));
#96254=CARTESIAN_POINT('Ctrl Pts',(113.835936540232,17.5989901474718,26.));
#96255=CARTESIAN_POINT('Ctrl Pts',(113.815484626163,17.5966833027337,31.));
#96256=CARTESIAN_POINT('Ctrl Pts',(113.815484626163,17.5966833027337,26.));
#96257=CARTESIAN_POINT('Ctrl Pts',(113.796469501718,17.5950039036449,31.));
#96258=CARTESIAN_POINT('Ctrl Pts',(113.796469501718,17.5950039036449,26.));
#96259=CARTESIAN_POINT('Ctrl Pts',(113.779011346312,17.5939428717583,31.));
#96260=CARTESIAN_POINT('Ctrl Pts',(113.779011346312,17.5939428717583,26.));
#96261=CARTESIAN_POINT('Ctrl Pts',(113.763172329554,17.5934919746174,31.));
#96262=CARTESIAN_POINT('Ctrl Pts',(113.763172329554,17.5934919746174,26.));
#96263=CARTESIAN_POINT('Ctrl Pts',(113.751816280133,17.5936140643445,31.));
#96264=CARTESIAN_POINT('Ctrl Pts',(113.751816280133,17.5936140643445,26.));
#96265=CARTESIAN_POINT('Ctrl Pts',(113.744039893058,17.5939752288389,31.));
#96266=CARTESIAN_POINT('Ctrl Pts',(113.744039893058,17.5939752288389,26.));
#96267=CARTESIAN_POINT('Ctrl Pts',(113.739184232663,17.5943356095541,31.));
#96268=CARTESIAN_POINT('Ctrl Pts',(113.739184232663,17.5943356095541,26.));
#96269=CARTESIAN_POINT('Ctrl Pts',(113.736838551019,17.5945457010101,31.));
#96270=CARTESIAN_POINT('Ctrl Pts',(113.736838551019,17.5945457010101,26.));
#96271=CARTESIAN_POINT('',(114.497698588799,17.8560993248145,31.));
#96272=CARTESIAN_POINT('Ctrl Pts',(113.736838551019,17.5945457010101,31.));
#96273=CARTESIAN_POINT('Ctrl Pts',(113.739184232663,17.5943356095541,31.));
#96274=CARTESIAN_POINT('Ctrl Pts',(113.744039893058,17.5939752288389,31.));
#96275=CARTESIAN_POINT('Ctrl Pts',(113.751816280133,17.5936140643445,31.));
#96276=CARTESIAN_POINT('Ctrl Pts',(113.763172329554,17.5934919746174,31.));
#96277=CARTESIAN_POINT('Ctrl Pts',(113.779011346312,17.5939428717583,31.));
#96278=CARTESIAN_POINT('Ctrl Pts',(113.796469501718,17.5950039036449,31.));
#96279=CARTESIAN_POINT('Ctrl Pts',(113.815484626163,17.5966833027337,31.));
#96280=CARTESIAN_POINT('Ctrl Pts',(113.835936540232,17.5989901474718,31.));
#96281=CARTESIAN_POINT('Ctrl Pts',(113.857643608343,17.6019337054866,31.));
#96282=CARTESIAN_POINT('Ctrl Pts',(113.880396659483,17.6055231460801,31.));
#96283=CARTESIAN_POINT('Ctrl Pts',(113.903986055947,17.6097670199576,31.));
#96284=CARTESIAN_POINT('Ctrl Pts',(113.928228583663,17.6146727719654,31.));
#96285=CARTESIAN_POINT('Ctrl Pts',(113.953000674982,17.6202458886071,31.));
#96286=CARTESIAN_POINT('Ctrl Pts',(113.978245673333,17.6264897903224,31.));
#96287=CARTESIAN_POINT('Ctrl Pts',(114.003948788046,17.6334066554963,31.));
#96288=CARTESIAN_POINT('Ctrl Pts',(114.030119893761,17.6409978615743,31.));
#96289=CARTESIAN_POINT('Ctrl Pts',(114.056774714484,17.6492644420825,31.));
#96290=CARTESIAN_POINT('Ctrl Pts',(114.083913156659,17.6582073519993,31.));
#96291=CARTESIAN_POINT('Ctrl Pts',(114.11151211949,17.667827787886,31.));
#96292=CARTESIAN_POINT('Ctrl Pts',(114.139535529399,17.6781275448076,31.));
#96293=CARTESIAN_POINT('Ctrl Pts',(114.167939811637,17.6891092498973,31.));
#96294=CARTESIAN_POINT('Ctrl Pts',(114.1966806629,17.7007764758468,31.));
#96295=CARTESIAN_POINT('Ctrl Pts',(114.225720115684,17.7131338314213,31.));
#96296=CARTESIAN_POINT('Ctrl Pts',(114.255030060531,17.72618667981,31.));
#96297=CARTESIAN_POINT('Ctrl Pts',(114.284589632559,17.73994036105,31.));
#96298=CARTESIAN_POINT('Ctrl Pts',(114.314384048769,17.7543993571629,31.));
#96299=CARTESIAN_POINT('Ctrl Pts',(114.344402900622,17.7695664156801,31.));
#96300=CARTESIAN_POINT('Ctrl Pts',(114.374638548468,17.7854413073407,31.));
#96301=CARTESIAN_POINT('Ctrl Pts',(114.405084808554,17.8020202406208,31.));
#96302=CARTESIAN_POINT('Ctrl Pts',(114.435737085489,17.8192978116112,31.));
#96303=CARTESIAN_POINT('Ctrl Pts',(114.46042119728,17.8336742788547,31.));
#96304=CARTESIAN_POINT('Ctrl Pts',(114.479024767707,17.8447665107748,31.));
#96305=CARTESIAN_POINT('Ctrl Pts',(114.491467291217,17.8522988075283,31.));
#96306=CARTESIAN_POINT('Ctrl Pts',(114.497698588799,17.8560993248145,31.));
#96307=CARTESIAN_POINT('',(114.497698588799,17.8560993248145,26.));
#96308=CARTESIAN_POINT('Ctrl Pts',(114.497698588799,17.8560993248145,26.));
#96309=CARTESIAN_POINT('Ctrl Pts',(114.491467291217,17.8522988075283,26.));
#96310=CARTESIAN_POINT('Ctrl Pts',(114.479024767707,17.8447665107748,26.));
#96311=CARTESIAN_POINT('Ctrl Pts',(114.46042119728,17.8336742788547,26.));
#96312=CARTESIAN_POINT('Ctrl Pts',(114.435737085489,17.8192978116112,26.));
#96313=CARTESIAN_POINT('Ctrl Pts',(114.405084808554,17.8020202406208,26.));
#96314=CARTESIAN_POINT('Ctrl Pts',(114.374638548468,17.7854413073407,26.));
#96315=CARTESIAN_POINT('Ctrl Pts',(114.344402900622,17.7695664156801,26.));
#96316=CARTESIAN_POINT('Ctrl Pts',(114.314384048769,17.7543993571629,26.));
#96317=CARTESIAN_POINT('Ctrl Pts',(114.284589632559,17.73994036105,26.));
#96318=CARTESIAN_POINT('Ctrl Pts',(114.255030060531,17.72618667981,26.));
#96319=CARTESIAN_POINT('Ctrl Pts',(114.225720115684,17.7131338314213,26.));
#96320=CARTESIAN_POINT('Ctrl Pts',(114.1966806629,17.7007764758468,26.));
#96321=CARTESIAN_POINT('Ctrl Pts',(114.167939811637,17.6891092498973,26.));
#96322=CARTESIAN_POINT('Ctrl Pts',(114.139535529399,17.6781275448076,26.));
#96323=CARTESIAN_POINT('Ctrl Pts',(114.11151211949,17.667827787886,26.));
#96324=CARTESIAN_POINT('Ctrl Pts',(114.083913156659,17.6582073519993,26.));
#96325=CARTESIAN_POINT('Ctrl Pts',(114.056774714484,17.6492644420825,26.));
#96326=CARTESIAN_POINT('Ctrl Pts',(114.030119893761,17.6409978615743,26.));
#96327=CARTESIAN_POINT('Ctrl Pts',(114.003948788046,17.6334066554963,26.));
#96328=CARTESIAN_POINT('Ctrl Pts',(113.978245673333,17.6264897903224,26.));
#96329=CARTESIAN_POINT('Ctrl Pts',(113.953000674982,17.6202458886071,26.));
#96330=CARTESIAN_POINT('Ctrl Pts',(113.928228583663,17.6146727719654,26.));
#96331=CARTESIAN_POINT('Ctrl Pts',(113.903986055947,17.6097670199576,26.));
#96332=CARTESIAN_POINT('Ctrl Pts',(113.880396659483,17.6055231460801,26.));
#96333=CARTESIAN_POINT('Ctrl Pts',(113.857643608343,17.6019337054866,26.));
#96334=CARTESIAN_POINT('Ctrl Pts',(113.835936540232,17.5989901474718,26.));
#96335=CARTESIAN_POINT('Ctrl Pts',(113.815484626163,17.5966833027337,26.));
#96336=CARTESIAN_POINT('Ctrl Pts',(113.796469501718,17.5950039036449,26.));
#96337=CARTESIAN_POINT('Ctrl Pts',(113.779011346312,17.5939428717583,26.));
#96338=CARTESIAN_POINT('Ctrl Pts',(113.763172329554,17.5934919746174,26.));
#96339=CARTESIAN_POINT('Ctrl Pts',(113.751816280133,17.5936140643445,26.));
#96340=CARTESIAN_POINT('Ctrl Pts',(113.744039893058,17.5939752288389,26.));
#96341=CARTESIAN_POINT('Ctrl Pts',(113.739184232663,17.5943356095541,26.));
#96342=CARTESIAN_POINT('Ctrl Pts',(113.736838551019,17.5945457010101,26.));
#96343=CARTESIAN_POINT('',(114.497698588799,17.8560993248145,31.));
#96344=CARTESIAN_POINT('Origin',(109.999999999997,18.,31.));
#96345=CARTESIAN_POINT('',(114.497698588799,18.1439006751855,31.));
#96346=CARTESIAN_POINT('Origin',(109.999999999997,18.,31.));
#96347=CARTESIAN_POINT('',(114.497698588799,18.1439006751855,26.));
#96348=CARTESIAN_POINT('Origin',(109.999999999997,18.,26.));
#96349=CARTESIAN_POINT('',(114.497698588799,18.1439006751855,31.));
#96350=CARTESIAN_POINT('Ctrl Pts',(113.736838551019,18.4054542989899,31.));
#96351=CARTESIAN_POINT('Ctrl Pts',(113.736838551019,18.4054542989899,26.));
#96352=CARTESIAN_POINT('Ctrl Pts',(113.739184232663,18.4056643904521,31.));
#96353=CARTESIAN_POINT('Ctrl Pts',(113.739184232663,18.4056643904521,26.));
#96354=CARTESIAN_POINT('Ctrl Pts',(113.744039893058,18.406024771178,31.));
#96355=CARTESIAN_POINT('Ctrl Pts',(113.744039893058,18.406024771178,26.));
#96356=CARTESIAN_POINT('Ctrl Pts',(113.751816280134,18.4063859356827,31.));
#96357=CARTESIAN_POINT('Ctrl Pts',(113.751816280134,18.4063859356827,26.));
#96358=CARTESIAN_POINT('Ctrl Pts',(113.763172329555,18.4065080254146,31.));
#96359=CARTESIAN_POINT('Ctrl Pts',(113.763172329555,18.4065080254146,26.));
#96360=CARTESIAN_POINT('Ctrl Pts',(113.779011346313,18.4060571282676,31.));
#96361=CARTESIAN_POINT('Ctrl Pts',(113.779011346313,18.4060571282676,26.));
#96362=CARTESIAN_POINT('Ctrl Pts',(113.796469501718,18.4049960963666,31.));
#96363=CARTESIAN_POINT('Ctrl Pts',(113.796469501718,18.4049960963666,26.));
#96364=CARTESIAN_POINT('Ctrl Pts',(113.815484626163,18.4033166972605,31.));
#96365=CARTESIAN_POINT('Ctrl Pts',(113.815484626163,18.4033166972605,26.));
#96366=CARTESIAN_POINT('Ctrl Pts',(113.835936540232,18.4010098525085,31.));
#96367=CARTESIAN_POINT('Ctrl Pts',(113.835936540232,18.4010098525085,26.));
#96368=CARTESIAN_POINT('Ctrl Pts',(113.857643608342,18.3980662944885,31.));
#96369=CARTESIAN_POINT('Ctrl Pts',(113.857643608342,18.3980662944885,26.));
#96370=CARTESIAN_POINT('Ctrl Pts',(113.880396659483,18.3944768538998,31.));
#96371=CARTESIAN_POINT('Ctrl Pts',(113.880396659483,18.3944768538998,26.));
#96372=CARTESIAN_POINT('Ctrl Pts',(113.903986055946,18.3902329800346,31.));
#96373=CARTESIAN_POINT('Ctrl Pts',(113.903986055946,18.3902329800346,26.));
#96374=CARTESIAN_POINT('Ctrl Pts',(113.928228583663,18.3853272280411,31.));
#96375=CARTESIAN_POINT('Ctrl Pts',(113.928228583663,18.3853272280411,26.));
#96376=CARTESIAN_POINT('Ctrl Pts',(113.953000674982,18.3797541114119,31.));
#96377=CARTESIAN_POINT('Ctrl Pts',(113.953000674982,18.3797541114119,26.));
#96378=CARTESIAN_POINT('Ctrl Pts',(113.978245673333,18.3735102097034,31.));
#96379=CARTESIAN_POINT('Ctrl Pts',(113.978245673333,18.3735102097034,26.));
#96380=CARTESIAN_POINT('Ctrl Pts',(114.003948788046,18.3665933445275,31.));
#96381=CARTESIAN_POINT('Ctrl Pts',(114.003948788046,18.3665933445275,26.));
#96382=CARTESIAN_POINT('Ctrl Pts',(114.030119893761,18.359002138437,31.));
#96383=CARTESIAN_POINT('Ctrl Pts',(114.030119893761,18.359002138437,26.));
#96384=CARTESIAN_POINT('Ctrl Pts',(114.056774714484,18.3507355579086,31.));
#96385=CARTESIAN_POINT('Ctrl Pts',(114.056774714484,18.3507355579086,26.));
#96386=CARTESIAN_POINT('Ctrl Pts',(114.083913156659,18.3417926479699,31.));
#96387=CARTESIAN_POINT('Ctrl Pts',(114.083913156659,18.3417926479699,26.));
#96388=CARTESIAN_POINT('Ctrl Pts',(114.11151211949,18.332172212069,31.));
#96389=CARTESIAN_POINT('Ctrl Pts',(114.11151211949,18.332172212069,26.));
#96390=CARTESIAN_POINT('Ctrl Pts',(114.139535529399,18.3218724551479,31.));
#96391=CARTESIAN_POINT('Ctrl Pts',(114.139535529399,18.3218724551479,26.));
#96392=CARTESIAN_POINT('Ctrl Pts',(114.167939811637,18.3108907500782,31.));
#96393=CARTESIAN_POINT('Ctrl Pts',(114.167939811637,18.3108907500782,26.));
#96394=CARTESIAN_POINT('Ctrl Pts',(114.1966806629,18.2992235241669,31.));
#96395=CARTESIAN_POINT('Ctrl Pts',(114.1966806629,18.2992235241669,26.));
#96396=CARTESIAN_POINT('Ctrl Pts',(114.225720115684,18.2868661686388,31.));
#96397=CARTESIAN_POINT('Ctrl Pts',(114.225720115684,18.2868661686388,26.));
#96398=CARTESIAN_POINT('Ctrl Pts',(114.255030060531,18.2738133202861,31.));
#96399=CARTESIAN_POINT('Ctrl Pts',(114.255030060531,18.2738133202861,26.));
#96400=CARTESIAN_POINT('Ctrl Pts',(114.284589632559,18.2600596390535,31.));
#96401=CARTESIAN_POINT('Ctrl Pts',(114.284589632559,18.2600596390535,26.));
#96402=CARTESIAN_POINT('Ctrl Pts',(114.314384048769,18.2456006429046,31.));
#96403=CARTESIAN_POINT('Ctrl Pts',(114.314384048769,18.2456006429046,26.));
#96404=CARTESIAN_POINT('Ctrl Pts',(114.344402900622,18.2304335843055,31.));
#96405=CARTESIAN_POINT('Ctrl Pts',(114.344402900622,18.2304335843055,26.));
#96406=CARTESIAN_POINT('Ctrl Pts',(114.374638548469,18.2145586925326,31.));
#96407=CARTESIAN_POINT('Ctrl Pts',(114.374638548469,18.2145586925326,26.));
#96408=CARTESIAN_POINT('Ctrl Pts',(114.405084808554,18.1979797591469,31.));
#96409=CARTESIAN_POINT('Ctrl Pts',(114.405084808554,18.1979797591469,26.));
#96410=CARTESIAN_POINT('Ctrl Pts',(114.435737085489,18.1807021881057,31.));
#96411=CARTESIAN_POINT('Ctrl Pts',(114.435737085489,18.1807021881057,26.));
#96412=CARTESIAN_POINT('Ctrl Pts',(114.460421197281,18.1663257209028,31.));
#96413=CARTESIAN_POINT('Ctrl Pts',(114.460421197281,18.1663257209028,26.));
#96414=CARTESIAN_POINT('Ctrl Pts',(114.479024767707,18.1552334890775,31.));
#96415=CARTESIAN_POINT('Ctrl Pts',(114.479024767707,18.1552334890775,26.));
#96416=CARTESIAN_POINT('Ctrl Pts',(114.491467291217,18.1477011924174,31.));
#96417=CARTESIAN_POINT('Ctrl Pts',(114.491467291217,18.1477011924174,26.));
#96418=CARTESIAN_POINT('Ctrl Pts',(114.497698588799,18.1439006751855,31.));
#96419=CARTESIAN_POINT('Ctrl Pts',(114.497698588799,18.1439006751855,26.));
#96420=CARTESIAN_POINT('Ctrl Pts',(113.736838551019,18.4054542989899,31.));
#96421=CARTESIAN_POINT('Ctrl Pts',(113.739184232663,18.4056643904521,31.));
#96422=CARTESIAN_POINT('Ctrl Pts',(113.744039893058,18.406024771178,31.));
#96423=CARTESIAN_POINT('Ctrl Pts',(113.751816280134,18.4063859356827,31.));
#96424=CARTESIAN_POINT('Ctrl Pts',(113.763172329555,18.4065080254146,31.));
#96425=CARTESIAN_POINT('Ctrl Pts',(113.779011346313,18.4060571282676,31.));
#96426=CARTESIAN_POINT('Ctrl Pts',(113.796469501718,18.4049960963666,31.));
#96427=CARTESIAN_POINT('Ctrl Pts',(113.815484626163,18.4033166972605,31.));
#96428=CARTESIAN_POINT('Ctrl Pts',(113.835936540232,18.4010098525085,31.));
#96429=CARTESIAN_POINT('Ctrl Pts',(113.857643608342,18.3980662944885,31.));
#96430=CARTESIAN_POINT('Ctrl Pts',(113.880396659483,18.3944768538998,31.));
#96431=CARTESIAN_POINT('Ctrl Pts',(113.903986055946,18.3902329800346,31.));
#96432=CARTESIAN_POINT('Ctrl Pts',(113.928228583663,18.3853272280411,31.));
#96433=CARTESIAN_POINT('Ctrl Pts',(113.953000674982,18.3797541114119,31.));
#96434=CARTESIAN_POINT('Ctrl Pts',(113.978245673333,18.3735102097034,31.));
#96435=CARTESIAN_POINT('Ctrl Pts',(114.003948788046,18.3665933445275,31.));
#96436=CARTESIAN_POINT('Ctrl Pts',(114.030119893761,18.359002138437,31.));
#96437=CARTESIAN_POINT('Ctrl Pts',(114.056774714484,18.3507355579086,31.));
#96438=CARTESIAN_POINT('Ctrl Pts',(114.083913156659,18.3417926479699,31.));
#96439=CARTESIAN_POINT('Ctrl Pts',(114.11151211949,18.332172212069,31.));
#96440=CARTESIAN_POINT('Ctrl Pts',(114.139535529399,18.3218724551479,31.));
#96441=CARTESIAN_POINT('Ctrl Pts',(114.167939811637,18.3108907500782,31.));
#96442=CARTESIAN_POINT('Ctrl Pts',(114.1966806629,18.2992235241669,31.));
#96443=CARTESIAN_POINT('Ctrl Pts',(114.225720115684,18.2868661686388,31.));
#96444=CARTESIAN_POINT('Ctrl Pts',(114.255030060531,18.2738133202861,31.));
#96445=CARTESIAN_POINT('Ctrl Pts',(114.284589632559,18.2600596390535,31.));
#96446=CARTESIAN_POINT('Ctrl Pts',(114.314384048769,18.2456006429046,31.));
#96447=CARTESIAN_POINT('Ctrl Pts',(114.344402900622,18.2304335843055,31.));
#96448=CARTESIAN_POINT('Ctrl Pts',(114.374638548469,18.2145586925326,31.));
#96449=CARTESIAN_POINT('Ctrl Pts',(114.405084808554,18.1979797591469,31.));
#96450=CARTESIAN_POINT('Ctrl Pts',(114.435737085489,18.1807021881057,31.));
#96451=CARTESIAN_POINT('Ctrl Pts',(114.460421197281,18.1663257209028,31.));
#96452=CARTESIAN_POINT('Ctrl Pts',(114.479024767707,18.1552334890775,31.));
#96453=CARTESIAN_POINT('Ctrl Pts',(114.491467291217,18.1477011924174,31.));
#96454=CARTESIAN_POINT('Ctrl Pts',(114.497698588799,18.1439006751855,31.));
#96455=CARTESIAN_POINT('Ctrl Pts',(113.736838551019,18.4054542989899,26.));
#96456=CARTESIAN_POINT('Ctrl Pts',(113.739184232663,18.4056643904521,26.));
#96457=CARTESIAN_POINT('Ctrl Pts',(113.744039893058,18.406024771178,26.));
#96458=CARTESIAN_POINT('Ctrl Pts',(113.751816280134,18.4063859356827,26.));
#96459=CARTESIAN_POINT('Ctrl Pts',(113.763172329555,18.4065080254146,26.));
#96460=CARTESIAN_POINT('Ctrl Pts',(113.779011346313,18.4060571282676,26.));
#96461=CARTESIAN_POINT('Ctrl Pts',(113.796469501718,18.4049960963666,26.));
#96462=CARTESIAN_POINT('Ctrl Pts',(113.815484626163,18.4033166972605,26.));
#96463=CARTESIAN_POINT('Ctrl Pts',(113.835936540232,18.4010098525085,26.));
#96464=CARTESIAN_POINT('Ctrl Pts',(113.857643608342,18.3980662944885,26.));
#96465=CARTESIAN_POINT('Ctrl Pts',(113.880396659483,18.3944768538998,26.));
#96466=CARTESIAN_POINT('Ctrl Pts',(113.903986055946,18.3902329800346,26.));
#96467=CARTESIAN_POINT('Ctrl Pts',(113.928228583663,18.3853272280411,26.));
#96468=CARTESIAN_POINT('Ctrl Pts',(113.953000674982,18.3797541114119,26.));
#96469=CARTESIAN_POINT('Ctrl Pts',(113.978245673333,18.3735102097034,26.));
#96470=CARTESIAN_POINT('Ctrl Pts',(114.003948788046,18.3665933445275,26.));
#96471=CARTESIAN_POINT('Ctrl Pts',(114.030119893761,18.359002138437,26.));
#96472=CARTESIAN_POINT('Ctrl Pts',(114.056774714484,18.3507355579086,26.));
#96473=CARTESIAN_POINT('Ctrl Pts',(114.083913156659,18.3417926479699,26.));
#96474=CARTESIAN_POINT('Ctrl Pts',(114.11151211949,18.332172212069,26.));
#96475=CARTESIAN_POINT('Ctrl Pts',(114.139535529399,18.3218724551479,26.));
#96476=CARTESIAN_POINT('Ctrl Pts',(114.167939811637,18.3108907500782,26.));
#96477=CARTESIAN_POINT('Ctrl Pts',(114.1966806629,18.2992235241669,26.));
#96478=CARTESIAN_POINT('Ctrl Pts',(114.225720115684,18.2868661686388,26.));
#96479=CARTESIAN_POINT('Ctrl Pts',(114.255030060531,18.2738133202861,26.));
#96480=CARTESIAN_POINT('Ctrl Pts',(114.284589632559,18.2600596390535,26.));
#96481=CARTESIAN_POINT('Ctrl Pts',(114.314384048769,18.2456006429046,26.));
#96482=CARTESIAN_POINT('Ctrl Pts',(114.344402900622,18.2304335843055,26.));
#96483=CARTESIAN_POINT('Ctrl Pts',(114.374638548469,18.2145586925326,26.));
#96484=CARTESIAN_POINT('Ctrl Pts',(114.405084808554,18.1979797591469,26.));
#96485=CARTESIAN_POINT('Ctrl Pts',(114.435737085489,18.1807021881057,26.));
#96486=CARTESIAN_POINT('Ctrl Pts',(114.460421197281,18.1663257209028,26.));
#96487=CARTESIAN_POINT('Ctrl Pts',(114.479024767707,18.1552334890775,26.));
#96488=CARTESIAN_POINT('Ctrl Pts',(114.491467291217,18.1477011924174,26.));
#96489=CARTESIAN_POINT('Ctrl Pts',(114.497698588799,18.1439006751855,26.));
#96490=CARTESIAN_POINT('Origin',(113.853091274272,18.000000000016,31.));
#96491=CARTESIAN_POINT('Origin',(113.095253230553,17.0944435750604,31.));
#96492=CARTESIAN_POINT('',(113.60754929639,16.9445647253073,31.));
#96493=CARTESIAN_POINT('',(113.60754929639,16.9445647253073,31.));
#96494=CARTESIAN_POINT('',(113.60754929639,16.9445647253073,26.));
#96495=CARTESIAN_POINT('',(113.60754929639,16.9445647253073,31.));
#96496=CARTESIAN_POINT('',(113.60754929639,16.9445647253073,26.));
#96497=CARTESIAN_POINT('Origin',(113.297228010781,16.1953828688964,31.));
#96498=CARTESIAN_POINT('',(113.297228010781,16.1953828688964,26.));
#96499=CARTESIAN_POINT('',(112.828999637636,16.451650540008,26.));
#96500=CARTESIAN_POINT('',(113.297228010781,16.1953828688964,31.));
#96501=CARTESIAN_POINT('',(113.297228010781,16.1953828688964,31.));
#96502=CARTESIAN_POINT('',(112.828999637636,16.451650540008,31.));
#96503=CARTESIAN_POINT('Ctrl Pts',(114.100263265296,16.1458583777765,31.));
#96504=CARTESIAN_POINT('Ctrl Pts',(114.100263265296,16.1458583777765,26.));
#96505=CARTESIAN_POINT('Ctrl Pts',(114.093051902,16.1447317719895,31.));
#96506=CARTESIAN_POINT('Ctrl Pts',(114.093051902,16.1447317719895,26.));
#96507=CARTESIAN_POINT('Ctrl Pts',(114.078674024021,16.1425343847903,31.));
#96508=CARTESIAN_POINT('Ctrl Pts',(114.078674024021,16.1425343847903,26.));
#96509=CARTESIAN_POINT('Ctrl Pts',(114.057241752688,16.1394057769344,31.));
#96510=CARTESIAN_POINT('Ctrl Pts',(114.057241752688,16.1394057769344,26.));
#96511=CARTESIAN_POINT('Ctrl Pts',(114.028934971196,16.1355698537236,31.));
#96512=CARTESIAN_POINT('Ctrl Pts',(114.028934971196,16.1355698537236,26.));
#96513=CARTESIAN_POINT('Ctrl Pts',(113.994004119741,16.1313375780615,31.));
#96514=CARTESIAN_POINT('Ctrl Pts',(113.994004119741,16.1313375780615,26.));
#96515=CARTESIAN_POINT('Ctrl Pts',(113.959530960114,16.1276719202451,31.));
#96516=CARTESIAN_POINT('Ctrl Pts',(113.959530960114,16.1276719202451,26.));
#96517=CARTESIAN_POINT('Ctrl Pts',(113.925521805887,16.1245761142569,31.));
#96518=CARTESIAN_POINT('Ctrl Pts',(113.925521805887,16.1245761142569,26.));
#96519=CARTESIAN_POINT('Ctrl Pts',(113.891983821059,16.1220512965871,31.));
#96520=CARTESIAN_POINT('Ctrl Pts',(113.891983821059,16.1220512965871,26.));
#96521=CARTESIAN_POINT('Ctrl Pts',(113.858924151478,16.1200947554784,31.));
#96522=CARTESIAN_POINT('Ctrl Pts',(113.858924151478,16.1200947554784,26.));
#96523=CARTESIAN_POINT('Ctrl Pts',(113.826351361947,16.118699969367,31.));
#96524=CARTESIAN_POINT('Ctrl Pts',(113.826351361947,16.118699969367,26.));
#96525=CARTESIAN_POINT('Ctrl Pts',(113.79427739498,16.1178571401962,31.));
#96526=CARTESIAN_POINT('Ctrl Pts',(113.79427739498,16.1178571401962,26.));
#96527=CARTESIAN_POINT('Ctrl Pts',(113.762719483672,16.1175533497701,31.));
#96528=CARTESIAN_POINT('Ctrl Pts',(113.762719483672,16.1175533497701,26.));
#96529=CARTESIAN_POINT('Ctrl Pts',(113.73170154537,16.1177728861249,31.));
#96530=CARTESIAN_POINT('Ctrl Pts',(113.73170154537,16.1177728861249,26.));
#96531=CARTESIAN_POINT('Ctrl Pts',(113.701256893778,16.1184969617808,31.));
#96532=CARTESIAN_POINT('Ctrl Pts',(113.701256893778,16.1184969617808,26.));
#96533=CARTESIAN_POINT('Ctrl Pts',(113.671425092601,16.1197053218617,31.));
#96534=CARTESIAN_POINT('Ctrl Pts',(113.671425092601,16.1197053218617,26.));
#96535=CARTESIAN_POINT('Ctrl Pts',(113.642245394296,16.1213788638783,31.));
#96536=CARTESIAN_POINT('Ctrl Pts',(113.642245394296,16.1213788638783,26.));
#96537=CARTESIAN_POINT('Ctrl Pts',(113.613750439565,16.1235021246454,31.));
#96538=CARTESIAN_POINT('Ctrl Pts',(113.613750439565,16.1235021246454,26.));
#96539=CARTESIAN_POINT('Ctrl Pts',(113.585961112853,16.1260651583935,31.));
#96540=CARTESIAN_POINT('Ctrl Pts',(113.585961112853,16.1260651583935,26.));
#96541=CARTESIAN_POINT('Ctrl Pts',(113.558877135142,16.1290670470348,31.));
#96542=CARTESIAN_POINT('Ctrl Pts',(113.558877135142,16.1290670470348,26.));
#96543=CARTESIAN_POINT('Ctrl Pts',(113.532483583831,16.1325128530322,31.));
#96544=CARTESIAN_POINT('Ctrl Pts',(113.532483583831,16.1325128530322,26.));
#96545=CARTESIAN_POINT('Ctrl Pts',(113.506770808816,16.1364050826537,31.));
#96546=CARTESIAN_POINT('Ctrl Pts',(113.506770808816,16.1364050826537,26.));
#96547=CARTESIAN_POINT('Ctrl Pts',(113.481751641264,16.1407360631888,31.));
#96548=CARTESIAN_POINT('Ctrl Pts',(113.481751641264,16.1407360631888,26.));
#96549=CARTESIAN_POINT('Ctrl Pts',(113.457477116074,16.1454809530329,31.));
#96550=CARTESIAN_POINT('Ctrl Pts',(113.457477116074,16.1454809530329,26.));
#96551=CARTESIAN_POINT('Ctrl Pts',(113.434059295275,16.1505873960249,31.));
#96552=CARTESIAN_POINT('Ctrl Pts',(113.434059295275,16.1505873960249,26.));
#96553=CARTESIAN_POINT('Ctrl Pts',(113.411664597577,16.1559784010347,31.));
#96554=CARTESIAN_POINT('Ctrl Pts',(113.411664597577,16.1559784010347,26.));
#96555=CARTESIAN_POINT('Ctrl Pts',(113.390483430755,16.1615658433631,31.));
#96556=CARTESIAN_POINT('Ctrl Pts',(113.390483430755,16.1615658433631,26.));
#96557=CARTESIAN_POINT('Ctrl Pts',(113.370705534684,16.1672612053993,31.));
#96558=CARTESIAN_POINT('Ctrl Pts',(113.370705534684,16.1672612053993,26.));
#96559=CARTESIAN_POINT('Ctrl Pts',(113.352495172193,16.1729864160438,31.));
#96560=CARTESIAN_POINT('Ctrl Pts',(113.352495172193,16.1729864160438,26.));
#96561=CARTESIAN_POINT('Ctrl Pts',(113.335959900414,16.178687097234,31.));
#96562=CARTESIAN_POINT('Ctrl Pts',(113.335959900414,16.178687097234,26.));
#96563=CARTESIAN_POINT('Ctrl Pts',(113.32115400615,16.1843318518923,31.));
#96564=CARTESIAN_POINT('Ctrl Pts',(113.32115400615,16.1843318518923,26.));
#96565=CARTESIAN_POINT('Ctrl Pts',(113.310709106236,16.188790420063,31.));
#96566=CARTESIAN_POINT('Ctrl Pts',(113.310709106236,16.188790420063,26.));
#96567=CARTESIAN_POINT('Ctrl Pts',(113.303662873049,16.1920999870445,31.));
#96568=CARTESIAN_POINT('Ctrl Pts',(113.303662873049,16.1920999870445,26.));
#96569=CARTESIAN_POINT('Ctrl Pts',(113.299314739522,16.1942911161974,31.));
#96570=CARTESIAN_POINT('Ctrl Pts',(113.299314739522,16.1942911161974,26.));
#96571=CARTESIAN_POINT('Ctrl Pts',(113.297228010781,16.1953828688964,31.));
#96572=CARTESIAN_POINT('Ctrl Pts',(113.297228010781,16.1953828688964,26.));
#96573=CARTESIAN_POINT('',(114.100263265296,16.1458583777765,31.));
#96574=CARTESIAN_POINT('Ctrl Pts',(113.297228010781,16.1953828688964,31.));
#96575=CARTESIAN_POINT('Ctrl Pts',(113.299314739522,16.1942911161974,31.));
#96576=CARTESIAN_POINT('Ctrl Pts',(113.303662873049,16.1920999870445,31.));
#96577=CARTESIAN_POINT('Ctrl Pts',(113.310709106236,16.188790420063,31.));
#96578=CARTESIAN_POINT('Ctrl Pts',(113.32115400615,16.1843318518923,31.));
#96579=CARTESIAN_POINT('Ctrl Pts',(113.335959900414,16.178687097234,31.));
#96580=CARTESIAN_POINT('Ctrl Pts',(113.352495172193,16.1729864160438,31.));
#96581=CARTESIAN_POINT('Ctrl Pts',(113.370705534684,16.1672612053993,31.));
#96582=CARTESIAN_POINT('Ctrl Pts',(113.390483430755,16.1615658433631,31.));
#96583=CARTESIAN_POINT('Ctrl Pts',(113.411664597577,16.1559784010347,31.));
#96584=CARTESIAN_POINT('Ctrl Pts',(113.434059295275,16.1505873960249,31.));
#96585=CARTESIAN_POINT('Ctrl Pts',(113.457477116074,16.1454809530329,31.));
#96586=CARTESIAN_POINT('Ctrl Pts',(113.481751641264,16.1407360631888,31.));
#96587=CARTESIAN_POINT('Ctrl Pts',(113.506770808816,16.1364050826537,31.));
#96588=CARTESIAN_POINT('Ctrl Pts',(113.532483583831,16.1325128530322,31.));
#96589=CARTESIAN_POINT('Ctrl Pts',(113.558877135142,16.1290670470348,31.));
#96590=CARTESIAN_POINT('Ctrl Pts',(113.585961112853,16.1260651583935,31.));
#96591=CARTESIAN_POINT('Ctrl Pts',(113.613750439565,16.1235021246454,31.));
#96592=CARTESIAN_POINT('Ctrl Pts',(113.642245394296,16.1213788638783,31.));
#96593=CARTESIAN_POINT('Ctrl Pts',(113.671425092601,16.1197053218617,31.));
#96594=CARTESIAN_POINT('Ctrl Pts',(113.701256893778,16.1184969617808,31.));
#96595=CARTESIAN_POINT('Ctrl Pts',(113.73170154537,16.1177728861249,31.));
#96596=CARTESIAN_POINT('Ctrl Pts',(113.762719483672,16.1175533497701,31.));
#96597=CARTESIAN_POINT('Ctrl Pts',(113.79427739498,16.1178571401962,31.));
#96598=CARTESIAN_POINT('Ctrl Pts',(113.826351361947,16.118699969367,31.));
#96599=CARTESIAN_POINT('Ctrl Pts',(113.858924151478,16.1200947554784,31.));
#96600=CARTESIAN_POINT('Ctrl Pts',(113.891983821059,16.1220512965871,31.));
#96601=CARTESIAN_POINT('Ctrl Pts',(113.925521805887,16.1245761142569,31.));
#96602=CARTESIAN_POINT('Ctrl Pts',(113.959530960114,16.1276719202451,31.));
#96603=CARTESIAN_POINT('Ctrl Pts',(113.994004119741,16.1313375780615,31.));
#96604=CARTESIAN_POINT('Ctrl Pts',(114.028934971196,16.1355698537236,31.));
#96605=CARTESIAN_POINT('Ctrl Pts',(114.057241752688,16.1394057769344,31.));
#96606=CARTESIAN_POINT('Ctrl Pts',(114.078674024021,16.1425343847903,31.));
#96607=CARTESIAN_POINT('Ctrl Pts',(114.093051902,16.1447317719895,31.));
#96608=CARTESIAN_POINT('Ctrl Pts',(114.100263265296,16.1458583777765,31.));
#96609=CARTESIAN_POINT('',(114.100263265296,16.1458583777765,26.));
#96610=CARTESIAN_POINT('Ctrl Pts',(114.100263265296,16.1458583777765,26.));
#96611=CARTESIAN_POINT('Ctrl Pts',(114.093051902,16.1447317719895,26.));
#96612=CARTESIAN_POINT('Ctrl Pts',(114.078674024021,16.1425343847903,26.));
#96613=CARTESIAN_POINT('Ctrl Pts',(114.057241752688,16.1394057769344,26.));
#96614=CARTESIAN_POINT('Ctrl Pts',(114.028934971196,16.1355698537236,26.));
#96615=CARTESIAN_POINT('Ctrl Pts',(113.994004119741,16.1313375780615,26.));
#96616=CARTESIAN_POINT('Ctrl Pts',(113.959530960114,16.1276719202451,26.));
#96617=CARTESIAN_POINT('Ctrl Pts',(113.925521805887,16.1245761142569,26.));
#96618=CARTESIAN_POINT('Ctrl Pts',(113.891983821059,16.1220512965871,26.));
#96619=CARTESIAN_POINT('Ctrl Pts',(113.858924151478,16.1200947554784,26.));
#96620=CARTESIAN_POINT('Ctrl Pts',(113.826351361947,16.118699969367,26.));
#96621=CARTESIAN_POINT('Ctrl Pts',(113.79427739498,16.1178571401962,26.));
#96622=CARTESIAN_POINT('Ctrl Pts',(113.762719483672,16.1175533497701,26.));
#96623=CARTESIAN_POINT('Ctrl Pts',(113.73170154537,16.1177728861249,26.));
#96624=CARTESIAN_POINT('Ctrl Pts',(113.701256893778,16.1184969617808,26.));
#96625=CARTESIAN_POINT('Ctrl Pts',(113.671425092601,16.1197053218617,26.));
#96626=CARTESIAN_POINT('Ctrl Pts',(113.642245394296,16.1213788638783,26.));
#96627=CARTESIAN_POINT('Ctrl Pts',(113.613750439565,16.1235021246454,26.));
#96628=CARTESIAN_POINT('Ctrl Pts',(113.585961112853,16.1260651583935,26.));
#96629=CARTESIAN_POINT('Ctrl Pts',(113.558877135142,16.1290670470348,26.));
#96630=CARTESIAN_POINT('Ctrl Pts',(113.532483583831,16.1325128530322,26.));
#96631=CARTESIAN_POINT('Ctrl Pts',(113.506770808816,16.1364050826537,26.));
#96632=CARTESIAN_POINT('Ctrl Pts',(113.481751641264,16.1407360631888,26.));
#96633=CARTESIAN_POINT('Ctrl Pts',(113.457477116074,16.1454809530329,26.));
#96634=CARTESIAN_POINT('Ctrl Pts',(113.434059295275,16.1505873960249,26.));
#96635=CARTESIAN_POINT('Ctrl Pts',(113.411664597577,16.1559784010347,26.));
#96636=CARTESIAN_POINT('Ctrl Pts',(113.390483430755,16.1615658433631,26.));
#96637=CARTESIAN_POINT('Ctrl Pts',(113.370705534684,16.1672612053993,26.));
#96638=CARTESIAN_POINT('Ctrl Pts',(113.352495172193,16.1729864160438,26.));
#96639=CARTESIAN_POINT('Ctrl Pts',(113.335959900414,16.178687097234,26.));
#96640=CARTESIAN_POINT('Ctrl Pts',(113.32115400615,16.1843318518923,26.));
#96641=CARTESIAN_POINT('Ctrl Pts',(113.310709106236,16.188790420063,26.));
#96642=CARTESIAN_POINT('Ctrl Pts',(113.303662873049,16.1920999870445,26.));
#96643=CARTESIAN_POINT('Ctrl Pts',(113.299314739522,16.1942911161974,26.));
#96644=CARTESIAN_POINT('Ctrl Pts',(113.297228010781,16.1953828688964,26.));
#96645=CARTESIAN_POINT('',(114.100263265296,16.1458583777765,31.));
#96646=CARTESIAN_POINT('Origin',(109.999999999997,18.0000000000012,31.));
#96647=CARTESIAN_POINT('',(114.210400073896,16.4117521548133,31.));
#96648=CARTESIAN_POINT('Origin',(109.999999999997,18.0000000000012,31.));
#96649=CARTESIAN_POINT('',(114.210400073896,16.4117521548133,26.));
#96650=CARTESIAN_POINT('Origin',(109.999999999997,18.0000000000012,26.));
#96651=CARTESIAN_POINT('',(114.210400073896,16.4117521548133,31.));
#96652=CARTESIAN_POINT('Ctrl Pts',(113.60754929639,16.9445647253073,31.));
#96653=CARTESIAN_POINT('Ctrl Pts',(113.60754929639,16.9445647253073,26.));
#96654=CARTESIAN_POINT('Ctrl Pts',(113.609796822173,16.9438611710063,31.));
#96655=CARTESIAN_POINT('Ctrl Pts',(113.609796822173,16.9438611710063,26.));
#96656=CARTESIAN_POINT('Ctrl Pts',(113.614420779162,16.9423359385965,31.));
#96657=CARTESIAN_POINT('Ctrl Pts',(113.614420779162,16.9423359385965,26.));
#96658=CARTESIAN_POINT('Ctrl Pts',(113.62174343569,16.9396937165929,31.));
#96659=CARTESIAN_POINT('Ctrl Pts',(113.62174343569,16.9396937165929,26.));
#96660=CARTESIAN_POINT('Ctrl Pts',(113.632281779039,16.9354607408266,31.));
#96661=CARTESIAN_POINT('Ctrl Pts',(113.632281779039,16.9354607408266,26.));
#96662=CARTESIAN_POINT('Ctrl Pts',(113.646742571568,16.9289828368832,31.));
#96663=CARTESIAN_POINT('Ctrl Pts',(113.646742571568,16.9289828368832,26.));
#96664=CARTESIAN_POINT('Ctrl Pts',(113.662465764693,16.9213216243932,31.));
#96665=CARTESIAN_POINT('Ctrl Pts',(113.662465764693,16.9213216243932,26.));
#96666=CARTESIAN_POINT('Ctrl Pts',(113.679390770761,16.9124932888427,31.));
#96667=CARTESIAN_POINT('Ctrl Pts',(113.679390770761,16.9124932888427,26.));
#96668=CARTESIAN_POINT('Ctrl Pts',(113.697403084302,16.9025354335174,31.));
#96669=CARTESIAN_POINT('Ctrl Pts',(113.697403084302,16.9025354335174,26.));
#96670=CARTESIAN_POINT('Ctrl Pts',(113.716331349354,16.891509005179,31.));
#96671=CARTESIAN_POINT('Ctrl Pts',(113.716331349354,16.891509005179,26.));
#96672=CARTESIAN_POINT('Ctrl Pts',(113.73597880816,16.8794855787786,31.));
#96673=CARTESIAN_POINT('Ctrl Pts',(113.73597880816,16.8794855787786,26.));
#96674=CARTESIAN_POINT('Ctrl Pts',(113.75614850852,16.8665374793698,31.));
#96675=CARTESIAN_POINT('Ctrl Pts',(113.75614850852,16.8665374793698,26.));
#96676=CARTESIAN_POINT('Ctrl Pts',(113.776668333682,16.8527279417957,31.));
#96677=CARTESIAN_POINT('Ctrl Pts',(113.776668333682,16.8527279417957,26.));
#96678=CARTESIAN_POINT('Ctrl Pts',(113.797422022429,16.8380991844769,31.));
#96679=CARTESIAN_POINT('Ctrl Pts',(113.797422022429,16.8380991844769,26.));
#96680=CARTESIAN_POINT('Ctrl Pts',(113.818355921967,16.8226697288662,31.));
#96681=CARTESIAN_POINT('Ctrl Pts',(113.818355921967,16.8226697288662,26.));
#96682=CARTESIAN_POINT('Ctrl Pts',(113.839455533865,16.8064432225404,31.));
#96683=CARTESIAN_POINT('Ctrl Pts',(113.839455533865,16.8064432225404,26.));
#96684=CARTESIAN_POINT('Ctrl Pts',(113.860729453975,16.7894146140426,31.));
#96685=CARTESIAN_POINT('Ctrl Pts',(113.860729453975,16.7894146140426,26.));
#96686=CARTESIAN_POINT('Ctrl Pts',(113.882191813874,16.7715769312051,31.));
#96687=CARTESIAN_POINT('Ctrl Pts',(113.882191813874,16.7715769312051,26.));
#96688=CARTESIAN_POINT('Ctrl Pts',(113.903842161673,16.7529293275511,31.));
#96689=CARTESIAN_POINT('Ctrl Pts',(113.903842161673,16.7529293275511,26.));
#96690=CARTESIAN_POINT('Ctrl Pts',(113.92565869712,16.7334795379024,31.));
#96691=CARTESIAN_POINT('Ctrl Pts',(113.92565869712,16.7334795379024,26.));
#96692=CARTESIAN_POINT('Ctrl Pts',(113.947607405635,16.7132397086026,31.));
#96693=CARTESIAN_POINT('Ctrl Pts',(113.947607405635,16.7132397086026,26.));
#96694=CARTESIAN_POINT('Ctrl Pts',(113.969647024041,16.6922240878361,31.));
#96695=CARTESIAN_POINT('Ctrl Pts',(113.969647024041,16.6922240878361,26.));
#96696=CARTESIAN_POINT('Ctrl Pts',(113.991735254212,16.6704463290048,31.));
#96697=CARTESIAN_POINT('Ctrl Pts',(113.991735254212,16.6704463290048,26.));
#96698=CARTESIAN_POINT('Ctrl Pts',(114.013835255045,16.6479167036913,31.));
#96699=CARTESIAN_POINT('Ctrl Pts',(114.013835255045,16.6479167036913,26.));
#96700=CARTESIAN_POINT('Ctrl Pts',(114.035919004379,16.6246410139608,31.));
#96701=CARTESIAN_POINT('Ctrl Pts',(114.035919004379,16.6246410139608,26.));
#96702=CARTESIAN_POINT('Ctrl Pts',(114.057965182023,16.6006223108904,31.));
#96703=CARTESIAN_POINT('Ctrl Pts',(114.057965182023,16.6006223108904,26.));
#96704=CARTESIAN_POINT('Ctrl Pts',(114.079958415069,16.5758621108271,31.));
#96705=CARTESIAN_POINT('Ctrl Pts',(114.079958415069,16.5758621108271,26.));
#96706=CARTESIAN_POINT('Ctrl Pts',(114.101888035841,16.5503618585562,31.));
#96707=CARTESIAN_POINT('Ctrl Pts',(114.101888035841,16.5503618585562,26.));
#96708=CARTESIAN_POINT('Ctrl Pts',(114.123747073967,16.5241246894687,31.));
#96709=CARTESIAN_POINT('Ctrl Pts',(114.123747073967,16.5241246894687,26.));
#96710=CARTESIAN_POINT('Ctrl Pts',(114.145531267368,16.4971564729307,31.));
#96711=CARTESIAN_POINT('Ctrl Pts',(114.145531267368,16.4971564729307,26.));
#96712=CARTESIAN_POINT('Ctrl Pts',(114.167238438465,16.4694639601268,31.));
#96713=CARTESIAN_POINT('Ctrl Pts',(114.167238438465,16.4694639601268,26.));
#96714=CARTESIAN_POINT('Ctrl Pts',(114.184541948313,16.446735635703,31.));
#96715=CARTESIAN_POINT('Ctrl Pts',(114.184541948313,16.446735635703,26.));
#96716=CARTESIAN_POINT('Ctrl Pts',(114.197484592914,16.4293684715648,31.));
#96717=CARTESIAN_POINT('Ctrl Pts',(114.197484592914,16.4293684715648,26.));
#96718=CARTESIAN_POINT('Ctrl Pts',(114.206097500578,16.4176479892436,31.));
#96719=CARTESIAN_POINT('Ctrl Pts',(114.206097500578,16.4176479892436,26.));
#96720=CARTESIAN_POINT('Ctrl Pts',(114.210400073896,16.4117521548133,31.));
#96721=CARTESIAN_POINT('Ctrl Pts',(114.210400073896,16.4117521548133,26.));
#96722=CARTESIAN_POINT('Ctrl Pts',(113.60754929639,16.9445647253073,31.));
#96723=CARTESIAN_POINT('Ctrl Pts',(113.609796822173,16.9438611710063,31.));
#96724=CARTESIAN_POINT('Ctrl Pts',(113.614420779162,16.9423359385965,31.));
#96725=CARTESIAN_POINT('Ctrl Pts',(113.62174343569,16.9396937165929,31.));
#96726=CARTESIAN_POINT('Ctrl Pts',(113.632281779039,16.9354607408266,31.));
#96727=CARTESIAN_POINT('Ctrl Pts',(113.646742571568,16.9289828368832,31.));
#96728=CARTESIAN_POINT('Ctrl Pts',(113.662465764693,16.9213216243932,31.));
#96729=CARTESIAN_POINT('Ctrl Pts',(113.679390770761,16.9124932888427,31.));
#96730=CARTESIAN_POINT('Ctrl Pts',(113.697403084302,16.9025354335174,31.));
#96731=CARTESIAN_POINT('Ctrl Pts',(113.716331349354,16.891509005179,31.));
#96732=CARTESIAN_POINT('Ctrl Pts',(113.73597880816,16.8794855787786,31.));
#96733=CARTESIAN_POINT('Ctrl Pts',(113.75614850852,16.8665374793698,31.));
#96734=CARTESIAN_POINT('Ctrl Pts',(113.776668333682,16.8527279417957,31.));
#96735=CARTESIAN_POINT('Ctrl Pts',(113.797422022429,16.8380991844769,31.));
#96736=CARTESIAN_POINT('Ctrl Pts',(113.818355921967,16.8226697288662,31.));
#96737=CARTESIAN_POINT('Ctrl Pts',(113.839455533865,16.8064432225404,31.));
#96738=CARTESIAN_POINT('Ctrl Pts',(113.860729453975,16.7894146140426,31.));
#96739=CARTESIAN_POINT('Ctrl Pts',(113.882191813874,16.7715769312051,31.));
#96740=CARTESIAN_POINT('Ctrl Pts',(113.903842161673,16.7529293275511,31.));
#96741=CARTESIAN_POINT('Ctrl Pts',(113.92565869712,16.7334795379024,31.));
#96742=CARTESIAN_POINT('Ctrl Pts',(113.947607405635,16.7132397086026,31.));
#96743=CARTESIAN_POINT('Ctrl Pts',(113.969647024041,16.6922240878361,31.));
#96744=CARTESIAN_POINT('Ctrl Pts',(113.991735254212,16.6704463290048,31.));
#96745=CARTESIAN_POINT('Ctrl Pts',(114.013835255045,16.6479167036913,31.));
#96746=CARTESIAN_POINT('Ctrl Pts',(114.035919004379,16.6246410139608,31.));
#96747=CARTESIAN_POINT('Ctrl Pts',(114.057965182023,16.6006223108904,31.));
#96748=CARTESIAN_POINT('Ctrl Pts',(114.079958415069,16.5758621108271,31.));
#96749=CARTESIAN_POINT('Ctrl Pts',(114.101888035841,16.5503618585562,31.));
#96750=CARTESIAN_POINT('Ctrl Pts',(114.123747073967,16.5241246894687,31.));
#96751=CARTESIAN_POINT('Ctrl Pts',(114.145531267368,16.4971564729307,31.));
#96752=CARTESIAN_POINT('Ctrl Pts',(114.167238438465,16.4694639601268,31.));
#96753=CARTESIAN_POINT('Ctrl Pts',(114.184541948313,16.446735635703,31.));
#96754=CARTESIAN_POINT('Ctrl Pts',(114.197484592914,16.4293684715648,31.));
#96755=CARTESIAN_POINT('Ctrl Pts',(114.206097500578,16.4176479892436,31.));
#96756=CARTESIAN_POINT('Ctrl Pts',(114.210400073896,16.4117521548133,31.));
#96757=CARTESIAN_POINT('Ctrl Pts',(113.60754929639,16.9445647253073,26.));
#96758=CARTESIAN_POINT('Ctrl Pts',(113.609796822173,16.9438611710063,26.));
#96759=CARTESIAN_POINT('Ctrl Pts',(113.614420779162,16.9423359385965,26.));
#96760=CARTESIAN_POINT('Ctrl Pts',(113.62174343569,16.9396937165929,26.));
#96761=CARTESIAN_POINT('Ctrl Pts',(113.632281779039,16.9354607408266,26.));
#96762=CARTESIAN_POINT('Ctrl Pts',(113.646742571568,16.9289828368832,26.));
#96763=CARTESIAN_POINT('Ctrl Pts',(113.662465764693,16.9213216243932,26.));
#96764=CARTESIAN_POINT('Ctrl Pts',(113.679390770761,16.9124932888427,26.));
#96765=CARTESIAN_POINT('Ctrl Pts',(113.697403084302,16.9025354335174,26.));
#96766=CARTESIAN_POINT('Ctrl Pts',(113.716331349354,16.891509005179,26.));
#96767=CARTESIAN_POINT('Ctrl Pts',(113.73597880816,16.8794855787786,26.));
#96768=CARTESIAN_POINT('Ctrl Pts',(113.75614850852,16.8665374793698,26.));
#96769=CARTESIAN_POINT('Ctrl Pts',(113.776668333682,16.8527279417957,26.));
#96770=CARTESIAN_POINT('Ctrl Pts',(113.797422022429,16.8380991844769,26.));
#96771=CARTESIAN_POINT('Ctrl Pts',(113.818355921967,16.8226697288662,26.));
#96772=CARTESIAN_POINT('Ctrl Pts',(113.839455533865,16.8064432225404,26.));
#96773=CARTESIAN_POINT('Ctrl Pts',(113.860729453975,16.7894146140426,26.));
#96774=CARTESIAN_POINT('Ctrl Pts',(113.882191813874,16.7715769312051,26.));
#96775=CARTESIAN_POINT('Ctrl Pts',(113.903842161673,16.7529293275511,26.));
#96776=CARTESIAN_POINT('Ctrl Pts',(113.92565869712,16.7334795379024,26.));
#96777=CARTESIAN_POINT('Ctrl Pts',(113.947607405635,16.7132397086026,26.));
#96778=CARTESIAN_POINT('Ctrl Pts',(113.969647024041,16.6922240878361,26.));
#96779=CARTESIAN_POINT('Ctrl Pts',(113.991735254212,16.6704463290048,26.));
#96780=CARTESIAN_POINT('Ctrl Pts',(114.013835255045,16.6479167036913,26.));
#96781=CARTESIAN_POINT('Ctrl Pts',(114.035919004379,16.6246410139608,26.));
#96782=CARTESIAN_POINT('Ctrl Pts',(114.057965182023,16.6006223108904,26.));
#96783=CARTESIAN_POINT('Ctrl Pts',(114.079958415069,16.5758621108271,26.));
#96784=CARTESIAN_POINT('Ctrl Pts',(114.101888035841,16.5503618585562,26.));
#96785=CARTESIAN_POINT('Ctrl Pts',(114.123747073967,16.5241246894687,26.));
#96786=CARTESIAN_POINT('Ctrl Pts',(114.145531267368,16.4971564729307,26.));
#96787=CARTESIAN_POINT('Ctrl Pts',(114.167238438465,16.4694639601268,26.));
#96788=CARTESIAN_POINT('Ctrl Pts',(114.184541948313,16.446735635703,26.));
#96789=CARTESIAN_POINT('Ctrl Pts',(114.197484592914,16.4293684715648,26.));
#96790=CARTESIAN_POINT('Ctrl Pts',(114.206097500578,16.4176479892436,26.));
#96791=CARTESIAN_POINT('Ctrl Pts',(114.210400073896,16.4117521548133,26.));
#96792=CARTESIAN_POINT('Origin',(113.559792165204,16.5254858059605,31.));
#96793=CARTESIAN_POINT('Origin',(112.513099666751,15.978872823157,31.));
#96794=CARTESIAN_POINT('',(112.929043363902,15.6443556046521,31.));
#96795=CARTESIAN_POINT('',(112.929043363902,15.6443556046521,31.));
#96796=CARTESIAN_POINT('',(112.929043363902,15.6443556046521,26.));
#96797=CARTESIAN_POINT('',(112.929043363902,15.6443556046521,31.));
#96798=CARTESIAN_POINT('',(112.929043363902,15.6443556046521,26.));
#96799=CARTESIAN_POINT('Origin',(112.355644395348,15.0709566360981,31.));
#96800=CARTESIAN_POINT('',(112.355644395348,15.0709566360981,26.));
#96801=CARTESIAN_POINT('',(112.021127176843,15.4869003332485,26.));
#96802=CARTESIAN_POINT('',(112.355644395348,15.0709566360981,31.));
#96803=CARTESIAN_POINT('',(112.355644395348,15.0709566360981,31.));
#96804=CARTESIAN_POINT('',(112.021127176843,15.4869003332485,31.));
#96805=CARTESIAN_POINT('Ctrl Pts',(113.078600028632,14.7178936848864,31.));
#96806=CARTESIAN_POINT('Ctrl Pts',(113.078600028632,14.7178936848864,26.));
#96807=CARTESIAN_POINT('Ctrl Pts',(113.071506464311,14.719612506117,31.));
#96808=CARTESIAN_POINT('Ctrl Pts',(113.071506464311,14.719612506117,26.));
#96809=CARTESIAN_POINT('Ctrl Pts',(113.057382133449,14.7230845607538,31.));
#96810=CARTESIAN_POINT('Ctrl Pts',(113.057382133449,14.7230845607538,26.));
#96811=CARTESIAN_POINT('Ctrl Pts',(113.036384030238,14.7283958791472,31.));
#96812=CARTESIAN_POINT('Ctrl Pts',(113.036384030238,14.7283958791472,26.));
#96813=CARTESIAN_POINT('Ctrl Pts',(113.008764029925,14.7356844845053,31.));
#96814=CARTESIAN_POINT('Ctrl Pts',(113.008764029925,14.7356844845053,26.));
#96815=CARTESIAN_POINT('Ctrl Pts',(112.974872509435,14.7451418297753,31.));
#96816=CARTESIAN_POINT('Ctrl Pts',(112.974872509435,14.7451418297753,26.));
#96817=CARTESIAN_POINT('Ctrl Pts',(112.94162067632,14.7549475105959,31.));
#96818=CARTESIAN_POINT('Ctrl Pts',(112.94162067632,14.7549475105959,26.));
#96819=CARTESIAN_POINT('Ctrl Pts',(112.90901560115,14.7651020986781,31.));
#96820=CARTESIAN_POINT('Ctrl Pts',(112.90901560115,14.7651020986781,26.));
#96821=CARTESIAN_POINT('Ctrl Pts',(112.877064337514,14.7756039024585,31.));
#96822=CARTESIAN_POINT('Ctrl Pts',(112.877064337514,14.7756039024585,26.));
#96823=CARTESIAN_POINT('Ctrl Pts',(112.845772449569,14.7864476820017,31.));
#96824=CARTESIAN_POINT('Ctrl Pts',(112.845772449569,14.7864476820017,26.));
#96825=CARTESIAN_POINT('Ctrl Pts',(112.815145354468,14.7976241345605,31.));
#96826=CARTESIAN_POINT('Ctrl Pts',(112.815145354468,14.7976241345605,26.));
#96827=CARTESIAN_POINT('Ctrl Pts',(112.785190336101,14.8091196377086,31.));
#96828=CARTESIAN_POINT('Ctrl Pts',(112.785190336101,14.8091196377086,26.));
#96829=CARTESIAN_POINT('Ctrl Pts',(112.755918372192,14.8209156617695,31.));
#96830=CARTESIAN_POINT('Ctrl Pts',(112.755918372192,14.8209156617695,26.));
#96831=CARTESIAN_POINT('Ctrl Pts',(112.72734554678,14.8329885380086,31.));
#96832=CARTESIAN_POINT('Ctrl Pts',(112.72734554678,14.8329885380086,26.));
#96833=CARTESIAN_POINT('Ctrl Pts',(112.699495448057,14.8453081604554,31.));
#96834=CARTESIAN_POINT('Ctrl Pts',(112.699495448057,14.8453081604554,26.));
#96835=CARTESIAN_POINT('Ctrl Pts',(112.672396876915,14.8578406756703,31.));
#96836=CARTESIAN_POINT('Ctrl Pts',(112.672396876915,14.8578406756703,26.));
#96837=CARTESIAN_POINT('Ctrl Pts',(112.646078787689,14.8705534139887,31.));
#96838=CARTESIAN_POINT('Ctrl Pts',(112.646078787689,14.8705534139887,26.));
#96839=CARTESIAN_POINT('Ctrl Pts',(112.620565418951,14.8834195982355,31.));
#96840=CARTESIAN_POINT('Ctrl Pts',(112.620565418951,14.8834195982355,26.));
#96841=CARTESIAN_POINT('Ctrl Pts',(112.595872259332,14.8964220475858,31.));
#96842=CARTESIAN_POINT('Ctrl Pts',(112.595872259332,14.8964220475858,26.));
#96843=CARTESIAN_POINT('Ctrl Pts',(112.571998699714,14.9095600206129,31.));
#96844=CARTESIAN_POINT('Ctrl Pts',(112.571998699714,14.9095600206129,26.));
#96845=CARTESIAN_POINT('Ctrl Pts',(112.548932890734,14.9228439050547,31.));
#96846=CARTESIAN_POINT('Ctrl Pts',(112.548932890734,14.9228439050547,26.));
#96847=CARTESIAN_POINT('Ctrl Pts',(112.526666875965,14.9362797093362,31.));
#96848=CARTESIAN_POINT('Ctrl Pts',(112.526666875965,14.9362797093362,26.));
#96849=CARTESIAN_POINT('Ctrl Pts',(112.50520957364,14.9498554345222,31.));
#96850=CARTESIAN_POINT('Ctrl Pts',(112.50520957364,14.9498554345222,26.));
#96851=CARTESIAN_POINT('Ctrl Pts',(112.484598627387,14.9635285997518,31.));
#96852=CARTESIAN_POINT('Ctrl Pts',(112.484598627387,14.9635285997518,26.));
#96853=CARTESIAN_POINT('Ctrl Pts',(112.464917533186,14.9772079499578,31.));
#96854=CARTESIAN_POINT('Ctrl Pts',(112.464917533186,14.9772079499578,26.));
#96855=CARTESIAN_POINT('Ctrl Pts',(112.446290578648,14.9907586689278,31.));
#96856=CARTESIAN_POINT('Ctrl Pts',(112.446290578648,14.9907586689278,26.));
#96857=CARTESIAN_POINT('Ctrl Pts',(112.428859953754,15.0040264741551,31.));
#96858=CARTESIAN_POINT('Ctrl Pts',(112.428859953754,15.0040264741551,26.));
#96859=CARTESIAN_POINT('Ctrl Pts',(112.41276708107,15.0168569757243,31.));
#96860=CARTESIAN_POINT('Ctrl Pts',(112.41276708107,15.0168569757243,26.));
#96861=CARTESIAN_POINT('Ctrl Pts',(112.398133843146,15.0291151846807,31.));
#96862=CARTESIAN_POINT('Ctrl Pts',(112.398133843146,15.0291151846807,26.));
#96863=CARTESIAN_POINT('Ctrl Pts',(112.385038800229,15.0407097019132,31.));
#96864=CARTESIAN_POINT('Ctrl Pts',(112.385038800229,15.0407097019132,26.));
#96865=CARTESIAN_POINT('Ctrl Pts',(112.373520091646,15.0515907456439,31.));
#96866=CARTESIAN_POINT('Ctrl Pts',(112.373520091646,15.0515907456439,26.));
#96867=CARTESIAN_POINT('Ctrl Pts',(112.365576482567,15.0597070156712,31.));
#96868=CARTESIAN_POINT('Ctrl Pts',(112.365576482567,15.0597070156712,26.));
#96869=CARTESIAN_POINT('Ctrl Pts',(112.360333128396,15.0654611335682,31.));
#96870=CARTESIAN_POINT('Ctrl Pts',(112.360333128396,15.0654611335682,26.));
#96871=CARTESIAN_POINT('Ctrl Pts',(112.357154485652,15.0691494316078,31.));
#96872=CARTESIAN_POINT('Ctrl Pts',(112.357154485652,15.0691494316078,26.));
#96873=CARTESIAN_POINT('Ctrl Pts',(112.355644395348,15.0709566360981,31.));
#96874=CARTESIAN_POINT('Ctrl Pts',(112.355644395348,15.0709566360981,26.));
#96875=CARTESIAN_POINT('',(113.078600028632,14.7178936848864,31.));
#96876=CARTESIAN_POINT('Ctrl Pts',(112.355644395348,15.0709566360981,31.));
#96877=CARTESIAN_POINT('Ctrl Pts',(112.357154485652,15.0691494316078,31.));
#96878=CARTESIAN_POINT('Ctrl Pts',(112.360333128396,15.0654611335682,31.));
#96879=CARTESIAN_POINT('Ctrl Pts',(112.365576482567,15.0597070156712,31.));
#96880=CARTESIAN_POINT('Ctrl Pts',(112.373520091646,15.0515907456439,31.));
#96881=CARTESIAN_POINT('Ctrl Pts',(112.385038800229,15.0407097019132,31.));
#96882=CARTESIAN_POINT('Ctrl Pts',(112.398133843146,15.0291151846807,31.));
#96883=CARTESIAN_POINT('Ctrl Pts',(112.41276708107,15.0168569757243,31.));
#96884=CARTESIAN_POINT('Ctrl Pts',(112.428859953754,15.0040264741551,31.));
#96885=CARTESIAN_POINT('Ctrl Pts',(112.446290578648,14.9907586689278,31.));
#96886=CARTESIAN_POINT('Ctrl Pts',(112.464917533186,14.9772079499578,31.));
#96887=CARTESIAN_POINT('Ctrl Pts',(112.484598627387,14.9635285997518,31.));
#96888=CARTESIAN_POINT('Ctrl Pts',(112.50520957364,14.9498554345222,31.));
#96889=CARTESIAN_POINT('Ctrl Pts',(112.526666875965,14.9362797093362,31.));
#96890=CARTESIAN_POINT('Ctrl Pts',(112.548932890734,14.9228439050547,31.));
#96891=CARTESIAN_POINT('Ctrl Pts',(112.571998699714,14.9095600206129,31.));
#96892=CARTESIAN_POINT('Ctrl Pts',(112.595872259332,14.8964220475858,31.));
#96893=CARTESIAN_POINT('Ctrl Pts',(112.620565418951,14.8834195982355,31.));
#96894=CARTESIAN_POINT('Ctrl Pts',(112.646078787689,14.8705534139887,31.));
#96895=CARTESIAN_POINT('Ctrl Pts',(112.672396876915,14.8578406756703,31.));
#96896=CARTESIAN_POINT('Ctrl Pts',(112.699495448057,14.8453081604554,31.));
#96897=CARTESIAN_POINT('Ctrl Pts',(112.72734554678,14.8329885380086,31.));
#96898=CARTESIAN_POINT('Ctrl Pts',(112.755918372192,14.8209156617695,31.));
#96899=CARTESIAN_POINT('Ctrl Pts',(112.785190336101,14.8091196377086,31.));
#96900=CARTESIAN_POINT('Ctrl Pts',(112.815145354468,14.7976241345605,31.));
#96901=CARTESIAN_POINT('Ctrl Pts',(112.845772449569,14.7864476820017,31.));
#96902=CARTESIAN_POINT('Ctrl Pts',(112.877064337514,14.7756039024585,31.));
#96903=CARTESIAN_POINT('Ctrl Pts',(112.90901560115,14.7651020986781,31.));
#96904=CARTESIAN_POINT('Ctrl Pts',(112.94162067632,14.7549475105959,31.));
#96905=CARTESIAN_POINT('Ctrl Pts',(112.974872509435,14.7451418297753,31.));
#96906=CARTESIAN_POINT('Ctrl Pts',(113.008764029925,14.7356844845053,31.));
#96907=CARTESIAN_POINT('Ctrl Pts',(113.036384030238,14.7283958791472,31.));
#96908=CARTESIAN_POINT('Ctrl Pts',(113.057382133449,14.7230845607538,31.));
#96909=CARTESIAN_POINT('Ctrl Pts',(113.071506464311,14.719612506117,31.));
#96910=CARTESIAN_POINT('Ctrl Pts',(113.078600028632,14.7178936848864,31.));
#96911=CARTESIAN_POINT('',(113.078600028632,14.7178936848864,26.));
#96912=CARTESIAN_POINT('Ctrl Pts',(113.078600028632,14.7178936848864,26.));
#96913=CARTESIAN_POINT('Ctrl Pts',(113.071506464311,14.719612506117,26.));
#96914=CARTESIAN_POINT('Ctrl Pts',(113.057382133449,14.7230845607538,26.));
#96915=CARTESIAN_POINT('Ctrl Pts',(113.036384030238,14.7283958791472,26.));
#96916=CARTESIAN_POINT('Ctrl Pts',(113.008764029925,14.7356844845053,26.));
#96917=CARTESIAN_POINT('Ctrl Pts',(112.974872509435,14.7451418297753,26.));
#96918=CARTESIAN_POINT('Ctrl Pts',(112.94162067632,14.7549475105959,26.));
#96919=CARTESIAN_POINT('Ctrl Pts',(112.90901560115,14.7651020986781,26.));
#96920=CARTESIAN_POINT('Ctrl Pts',(112.877064337514,14.7756039024585,26.));
#96921=CARTESIAN_POINT('Ctrl Pts',(112.845772449569,14.7864476820017,26.));
#96922=CARTESIAN_POINT('Ctrl Pts',(112.815145354468,14.7976241345605,26.));
#96923=CARTESIAN_POINT('Ctrl Pts',(112.785190336101,14.8091196377086,26.));
#96924=CARTESIAN_POINT('Ctrl Pts',(112.755918372192,14.8209156617695,26.));
#96925=CARTESIAN_POINT('Ctrl Pts',(112.72734554678,14.8329885380086,26.));
#96926=CARTESIAN_POINT('Ctrl Pts',(112.699495448057,14.8453081604554,26.));
#96927=CARTESIAN_POINT('Ctrl Pts',(112.672396876915,14.8578406756703,26.));
#96928=CARTESIAN_POINT('Ctrl Pts',(112.646078787689,14.8705534139887,26.));
#96929=CARTESIAN_POINT('Ctrl Pts',(112.620565418951,14.8834195982355,26.));
#96930=CARTESIAN_POINT('Ctrl Pts',(112.595872259332,14.8964220475858,26.));
#96931=CARTESIAN_POINT('Ctrl Pts',(112.571998699714,14.9095600206129,26.));
#96932=CARTESIAN_POINT('Ctrl Pts',(112.548932890734,14.9228439050547,26.));
#96933=CARTESIAN_POINT('Ctrl Pts',(112.526666875965,14.9362797093362,26.));
#96934=CARTESIAN_POINT('Ctrl Pts',(112.50520957364,14.9498554345222,26.));
#96935=CARTESIAN_POINT('Ctrl Pts',(112.484598627387,14.9635285997518,26.));
#96936=CARTESIAN_POINT('Ctrl Pts',(112.464917533186,14.9772079499578,26.));
#96937=CARTESIAN_POINT('Ctrl Pts',(112.446290578648,14.9907586689278,26.));
#96938=CARTESIAN_POINT('Ctrl Pts',(112.428859953754,15.0040264741551,26.));
#96939=CARTESIAN_POINT('Ctrl Pts',(112.41276708107,15.0168569757243,26.));
#96940=CARTESIAN_POINT('Ctrl Pts',(112.398133843146,15.0291151846807,26.));
#96941=CARTESIAN_POINT('Ctrl Pts',(112.385038800229,15.0407097019132,26.));
#96942=CARTESIAN_POINT('Ctrl Pts',(112.373520091646,15.0515907456439,26.));
#96943=CARTESIAN_POINT('Ctrl Pts',(112.365576482567,15.0597070156712,26.));
#96944=CARTESIAN_POINT('Ctrl Pts',(112.360333128396,15.0654611335682,26.));
#96945=CARTESIAN_POINT('Ctrl Pts',(112.357154485652,15.0691494316078,26.));
#96946=CARTESIAN_POINT('Ctrl Pts',(112.355644395348,15.0709566360981,26.));
#96947=CARTESIAN_POINT('',(113.078600028632,14.7178936848864,31.));
#96948=CARTESIAN_POINT('Origin',(109.999999999998,18.0000000000022,31.));
#96949=CARTESIAN_POINT('',(113.282106315114,14.9213999713683,31.));
#96950=CARTESIAN_POINT('Origin',(109.999999999998,18.0000000000022,31.));
#96951=CARTESIAN_POINT('',(113.282106315114,14.9213999713683,26.));
#96952=CARTESIAN_POINT('Origin',(109.999999999998,18.0000000000022,26.));
#96953=CARTESIAN_POINT('',(113.282106315114,14.9213999713683,31.));
#96954=CARTESIAN_POINT('Ctrl Pts',(112.929043363902,15.6443556046521,31.));
#96955=CARTESIAN_POINT('Ctrl Pts',(112.929043363902,15.6443556046521,26.));
#96956=CARTESIAN_POINT('Ctrl Pts',(112.930850568397,15.6428455143525,31.));
#96957=CARTESIAN_POINT('Ctrl Pts',(112.930850568397,15.6428455143525,26.));
#96958=CARTESIAN_POINT('Ctrl Pts',(112.934538866444,15.6396668716152,31.));
#96959=CARTESIAN_POINT('Ctrl Pts',(112.934538866444,15.6396668716152,26.));
#96960=CARTESIAN_POINT('Ctrl Pts',(112.940292984349,15.6344235174514,31.));
#96961=CARTESIAN_POINT('Ctrl Pts',(112.940292984349,15.6344235174514,26.));
#96962=CARTESIAN_POINT('Ctrl Pts',(112.94840925438,15.6264799083753,31.));
#96963=CARTESIAN_POINT('Ctrl Pts',(112.94840925438,15.6264799083753,26.));
#96964=CARTESIAN_POINT('Ctrl Pts',(112.959290298106,15.6149611997885,31.));
#96965=CARTESIAN_POINT('Ctrl Pts',(112.959290298106,15.6149611997885,26.));
#96966=CARTESIAN_POINT('Ctrl Pts',(112.970884815328,15.6018661568621,31.));
#96967=CARTESIAN_POINT('Ctrl Pts',(112.970884815328,15.6018661568621,26.));
#96968=CARTESIAN_POINT('Ctrl Pts',(112.983143024272,15.5872329189258,31.));
#96969=CARTESIAN_POINT('Ctrl Pts',(112.983143024272,15.5872329189258,26.));
#96970=CARTESIAN_POINT('Ctrl Pts',(112.99597352583,15.5711400462322,31.));
#96971=CARTESIAN_POINT('Ctrl Pts',(112.99597352583,15.5711400462322,26.));
#96972=CARTESIAN_POINT('Ctrl Pts',(113.009241331054,15.5537094213352,31.));
#96973=CARTESIAN_POINT('Ctrl Pts',(113.009241331054,15.5537094213352,26.));
#96974=CARTESIAN_POINT('Ctrl Pts',(113.022792050028,15.5350824667997,31.));
#96975=CARTESIAN_POINT('Ctrl Pts',(113.022792050028,15.5350824667997,26.));
#96976=CARTESIAN_POINT('Ctrl Pts',(113.036471400243,15.5154013726076,31.));
#96977=CARTESIAN_POINT('Ctrl Pts',(113.036471400243,15.5154013726076,26.));
#96978=CARTESIAN_POINT('Ctrl Pts',(113.050144565483,15.4947904263648,31.));
#96979=CARTESIAN_POINT('Ctrl Pts',(113.050144565483,15.4947904263648,26.));
#96980=CARTESIAN_POINT('Ctrl Pts',(113.063720290677,15.4733331240482,31.));
#96981=CARTESIAN_POINT('Ctrl Pts',(113.063720290677,15.4733331240482,26.));
#96982=CARTESIAN_POINT('Ctrl Pts',(113.077156094964,15.4510671092837,31.));
#96983=CARTESIAN_POINT('Ctrl Pts',(113.077156094964,15.4510671092837,26.));
#96984=CARTESIAN_POINT('Ctrl Pts',(113.090439979404,15.4280013003025,31.));
#96985=CARTESIAN_POINT('Ctrl Pts',(113.090439979404,15.4280013003025,26.));
#96986=CARTESIAN_POINT('Ctrl Pts',(113.103577952422,15.4041277406764,31.));
#96987=CARTESIAN_POINT('Ctrl Pts',(113.103577952422,15.4041277406764,26.));
#96988=CARTESIAN_POINT('Ctrl Pts',(113.116580401758,15.3794345810427,31.));
#96989=CARTESIAN_POINT('Ctrl Pts',(113.116580401758,15.3794345810427,26.));
#96990=CARTESIAN_POINT('Ctrl Pts',(113.12944658599,15.3539212122889,31.));
#96991=CARTESIAN_POINT('Ctrl Pts',(113.12944658599,15.3539212122889,26.));
#96992=CARTESIAN_POINT('Ctrl Pts',(113.142159324298,15.3276031230536,31.));
#96993=CARTESIAN_POINT('Ctrl Pts',(113.142159324298,15.3276031230536,26.));
#96994=CARTESIAN_POINT('Ctrl Pts',(113.154691839513,15.3005045519114,31.));
#96995=CARTESIAN_POINT('Ctrl Pts',(113.154691839513,15.3005045519114,26.));
#96996=CARTESIAN_POINT('Ctrl Pts',(113.167011461974,15.2726544532028,31.));
#96997=CARTESIAN_POINT('Ctrl Pts',(113.167011461974,15.2726544532028,26.));
#96998=CARTESIAN_POINT('Ctrl Pts',(113.17908433824,15.2440816278177,31.));
#96999=CARTESIAN_POINT('Ctrl Pts',(113.17908433824,15.2440816278177,26.));
#97000=CARTESIAN_POINT('Ctrl Pts',(113.190880362334,15.2148096639412,31.));
#97001=CARTESIAN_POINT('Ctrl Pts',(113.190880362334,15.2148096639412,26.));
#97002=CARTESIAN_POINT('Ctrl Pts',(113.202375865507,15.1848546455997,31.));
#97003=CARTESIAN_POINT('Ctrl Pts',(113.202375865507,15.1848546455997,26.));
#97004=CARTESIAN_POINT('Ctrl Pts',(113.213552318071,15.1542275505039,31.));
#97005=CARTESIAN_POINT('Ctrl Pts',(113.213552318071,15.1542275505039,26.));
#97006=CARTESIAN_POINT('Ctrl Pts',(113.224396097589,15.1229356625341,31.));
#97007=CARTESIAN_POINT('Ctrl Pts',(113.224396097589,15.1229356625341,26.));
#97008=CARTESIAN_POINT('Ctrl Pts',(113.234897901312,15.0909843988393,31.));
#97009=CARTESIAN_POINT('Ctrl Pts',(113.234897901312,15.0909843988393,26.));
#97010=CARTESIAN_POINT('Ctrl Pts',(113.245052489315,15.0583793235901,31.));
#97011=CARTESIAN_POINT('Ctrl Pts',(113.245052489315,15.0583793235901,26.));
#97012=CARTESIAN_POINT('Ctrl Pts',(113.254858170061,15.0251274904002,31.));
#97013=CARTESIAN_POINT('Ctrl Pts',(113.254858170061,15.0251274904002,26.));
#97014=CARTESIAN_POINT('Ctrl Pts',(113.264315515295,14.9912359698749,31.));
#97015=CARTESIAN_POINT('Ctrl Pts',(113.264315515295,14.9912359698749,26.));
#97016=CARTESIAN_POINT('Ctrl Pts',(113.271604120682,14.9636159695907,31.));
#97017=CARTESIAN_POINT('Ctrl Pts',(113.271604120682,14.9636159695907,26.));
#97018=CARTESIAN_POINT('Ctrl Pts',(113.276915439142,14.942617866446,31.));
#97019=CARTESIAN_POINT('Ctrl Pts',(113.276915439142,14.942617866446,26.));
#97020=CARTESIAN_POINT('Ctrl Pts',(113.280387493845,14.9284935356507,31.));
#97021=CARTESIAN_POINT('Ctrl Pts',(113.280387493845,14.9284935356507,26.));
#97022=CARTESIAN_POINT('Ctrl Pts',(113.282106315114,14.9213999713683,31.));
#97023=CARTESIAN_POINT('Ctrl Pts',(113.282106315114,14.9213999713683,26.));
#97024=CARTESIAN_POINT('Ctrl Pts',(112.929043363902,15.6443556046521,31.));
#97025=CARTESIAN_POINT('Ctrl Pts',(112.930850568397,15.6428455143525,31.));
#97026=CARTESIAN_POINT('Ctrl Pts',(112.934538866444,15.6396668716152,31.));
#97027=CARTESIAN_POINT('Ctrl Pts',(112.940292984349,15.6344235174514,31.));
#97028=CARTESIAN_POINT('Ctrl Pts',(112.94840925438,15.6264799083753,31.));
#97029=CARTESIAN_POINT('Ctrl Pts',(112.959290298106,15.6149611997885,31.));
#97030=CARTESIAN_POINT('Ctrl Pts',(112.970884815328,15.6018661568621,31.));
#97031=CARTESIAN_POINT('Ctrl Pts',(112.983143024272,15.5872329189258,31.));
#97032=CARTESIAN_POINT('Ctrl Pts',(112.99597352583,15.5711400462322,31.));
#97033=CARTESIAN_POINT('Ctrl Pts',(113.009241331054,15.5537094213352,31.));
#97034=CARTESIAN_POINT('Ctrl Pts',(113.022792050028,15.5350824667997,31.));
#97035=CARTESIAN_POINT('Ctrl Pts',(113.036471400243,15.5154013726076,31.));
#97036=CARTESIAN_POINT('Ctrl Pts',(113.050144565483,15.4947904263648,31.));
#97037=CARTESIAN_POINT('Ctrl Pts',(113.063720290677,15.4733331240482,31.));
#97038=CARTESIAN_POINT('Ctrl Pts',(113.077156094964,15.4510671092837,31.));
#97039=CARTESIAN_POINT('Ctrl Pts',(113.090439979404,15.4280013003025,31.));
#97040=CARTESIAN_POINT('Ctrl Pts',(113.103577952422,15.4041277406764,31.));
#97041=CARTESIAN_POINT('Ctrl Pts',(113.116580401758,15.3794345810427,31.));
#97042=CARTESIAN_POINT('Ctrl Pts',(113.12944658599,15.3539212122889,31.));
#97043=CARTESIAN_POINT('Ctrl Pts',(113.142159324298,15.3276031230536,31.));
#97044=CARTESIAN_POINT('Ctrl Pts',(113.154691839513,15.3005045519114,31.));
#97045=CARTESIAN_POINT('Ctrl Pts',(113.167011461974,15.2726544532028,31.));
#97046=CARTESIAN_POINT('Ctrl Pts',(113.17908433824,15.2440816278177,31.));
#97047=CARTESIAN_POINT('Ctrl Pts',(113.190880362334,15.2148096639412,31.));
#97048=CARTESIAN_POINT('Ctrl Pts',(113.202375865507,15.1848546455997,31.));
#97049=CARTESIAN_POINT('Ctrl Pts',(113.213552318071,15.1542275505039,31.));
#97050=CARTESIAN_POINT('Ctrl Pts',(113.224396097589,15.1229356625341,31.));
#97051=CARTESIAN_POINT('Ctrl Pts',(113.234897901312,15.0909843988393,31.));
#97052=CARTESIAN_POINT('Ctrl Pts',(113.245052489315,15.0583793235901,31.));
#97053=CARTESIAN_POINT('Ctrl Pts',(113.254858170061,15.0251274904002,31.));
#97054=CARTESIAN_POINT('Ctrl Pts',(113.264315515295,14.9912359698749,31.));
#97055=CARTESIAN_POINT('Ctrl Pts',(113.271604120682,14.9636159695907,31.));
#97056=CARTESIAN_POINT('Ctrl Pts',(113.276915439142,14.942617866446,31.));
#97057=CARTESIAN_POINT('Ctrl Pts',(113.280387493845,14.9284935356507,31.));
#97058=CARTESIAN_POINT('Ctrl Pts',(113.282106315114,14.9213999713683,31.));
#97059=CARTESIAN_POINT('Ctrl Pts',(112.929043363902,15.6443556046521,26.));
#97060=CARTESIAN_POINT('Ctrl Pts',(112.930850568397,15.6428455143525,26.));
#97061=CARTESIAN_POINT('Ctrl Pts',(112.934538866444,15.6396668716152,26.));
#97062=CARTESIAN_POINT('Ctrl Pts',(112.940292984349,15.6344235174514,26.));
#97063=CARTESIAN_POINT('Ctrl Pts',(112.94840925438,15.6264799083753,26.));
#97064=CARTESIAN_POINT('Ctrl Pts',(112.959290298106,15.6149611997885,26.));
#97065=CARTESIAN_POINT('Ctrl Pts',(112.970884815328,15.6018661568621,26.));
#97066=CARTESIAN_POINT('Ctrl Pts',(112.983143024272,15.5872329189258,26.));
#97067=CARTESIAN_POINT('Ctrl Pts',(112.99597352583,15.5711400462322,26.));
#97068=CARTESIAN_POINT('Ctrl Pts',(113.009241331054,15.5537094213352,26.));
#97069=CARTESIAN_POINT('Ctrl Pts',(113.022792050028,15.5350824667997,26.));
#97070=CARTESIAN_POINT('Ctrl Pts',(113.036471400243,15.5154013726076,26.));
#97071=CARTESIAN_POINT('Ctrl Pts',(113.050144565483,15.4947904263648,26.));
#97072=CARTESIAN_POINT('Ctrl Pts',(113.063720290677,15.4733331240482,26.));
#97073=CARTESIAN_POINT('Ctrl Pts',(113.077156094964,15.4510671092837,26.));
#97074=CARTESIAN_POINT('Ctrl Pts',(113.090439979404,15.4280013003025,26.));
#97075=CARTESIAN_POINT('Ctrl Pts',(113.103577952422,15.4041277406764,26.));
#97076=CARTESIAN_POINT('Ctrl Pts',(113.116580401758,15.3794345810427,26.));
#97077=CARTESIAN_POINT('Ctrl Pts',(113.12944658599,15.3539212122889,26.));
#97078=CARTESIAN_POINT('Ctrl Pts',(113.142159324298,15.3276031230536,26.));
#97079=CARTESIAN_POINT('Ctrl Pts',(113.154691839513,15.3005045519114,26.));
#97080=CARTESIAN_POINT('Ctrl Pts',(113.167011461974,15.2726544532028,26.));
#97081=CARTESIAN_POINT('Ctrl Pts',(113.17908433824,15.2440816278177,26.));
#97082=CARTESIAN_POINT('Ctrl Pts',(113.190880362334,15.2148096639412,26.));
#97083=CARTESIAN_POINT('Ctrl Pts',(113.202375865507,15.1848546455997,26.));
#97084=CARTESIAN_POINT('Ctrl Pts',(113.213552318071,15.1542275505039,26.));
#97085=CARTESIAN_POINT('Ctrl Pts',(113.224396097589,15.1229356625341,26.));
#97086=CARTESIAN_POINT('Ctrl Pts',(113.234897901312,15.0909843988393,26.));
#97087=CARTESIAN_POINT('Ctrl Pts',(113.245052489315,15.0583793235901,26.));
#97088=CARTESIAN_POINT('Ctrl Pts',(113.254858170061,15.0251274904002,26.));
#97089=CARTESIAN_POINT('Ctrl Pts',(113.264315515295,14.9912359698749,26.));
#97090=CARTESIAN_POINT('Ctrl Pts',(113.271604120682,14.9636159695907,26.));
#97091=CARTESIAN_POINT('Ctrl Pts',(113.276915439142,14.942617866446,26.));
#97092=CARTESIAN_POINT('Ctrl Pts',(113.280387493845,14.9284935356507,26.));
#97093=CARTESIAN_POINT('Ctrl Pts',(113.282106315114,14.9213999713683,26.));
#97094=CARTESIAN_POINT('Origin',(112.72454696858,15.2754530314429,31.));
#97095=CARTESIAN_POINT('Origin',(111.548349459992,15.1710003623644,31.));
#97096=CARTESIAN_POINT('',(111.804617131104,14.702771989219,31.));
#97097=CARTESIAN_POINT('',(111.804617131104,14.702771989219,31.));
#97098=CARTESIAN_POINT('',(111.804617131104,14.702771989219,26.));
#97099=CARTESIAN_POINT('',(111.804617131104,14.702771989219,31.));
#97100=CARTESIAN_POINT('',(111.804617131104,14.702771989219,26.));
#97101=CARTESIAN_POINT('Origin',(111.055435274693,14.3924507036097,31.));
#97102=CARTESIAN_POINT('',(111.055435274693,14.3924507036097,26.));
#97103=CARTESIAN_POINT('',(110.90555642494,14.9047467694467,26.));
#97104=CARTESIAN_POINT('',(111.055435274693,14.3924507036097,31.));
#97105=CARTESIAN_POINT('',(111.055435274693,14.3924507036097,31.));
#97106=CARTESIAN_POINT('',(110.90555642494,14.9047467694467,31.));
#97107=CARTESIAN_POINT('Ctrl Pts',(111.588247845187,13.7895999261044,31.));
#97108=CARTESIAN_POINT('Ctrl Pts',(111.588247845187,13.7895999261044,26.));
#97109=CARTESIAN_POINT('Ctrl Pts',(111.582352010706,13.7939024994014,31.));
#97110=CARTESIAN_POINT('Ctrl Pts',(111.582352010706,13.7939024994014,26.));
#97111=CARTESIAN_POINT('Ctrl Pts',(111.570631528299,13.80251540703,31.));
#97112=CARTESIAN_POINT('Ctrl Pts',(111.570631528299,13.80251540703,26.));
#97113=CARTESIAN_POINT('Ctrl Pts',(111.553264364073,13.8154580515946,31.));
#97114=CARTESIAN_POINT('Ctrl Pts',(111.553264364073,13.8154580515946,26.));
#97115=CARTESIAN_POINT('Ctrl Pts',(111.530536039611,13.8327615614272,31.));
#97116=CARTESIAN_POINT('Ctrl Pts',(111.530536039611,13.8327615614272,26.));
#97117=CARTESIAN_POINT('Ctrl Pts',(111.502843526855,13.8544687325429,31.));
#97118=CARTESIAN_POINT('Ctrl Pts',(111.502843526855,13.8544687325429,26.));
#97119=CARTESIAN_POINT('Ctrl Pts',(111.475875310414,13.8762529259845,31.));
#97120=CARTESIAN_POINT('Ctrl Pts',(111.475875310414,13.8762529259845,26.));
#97121=CARTESIAN_POINT('Ctrl Pts',(111.44963814143,13.8981119641531,31.));
#97122=CARTESIAN_POINT('Ctrl Pts',(111.44963814143,13.8981119641531,26.));
#97123=CARTESIAN_POINT('Ctrl Pts',(111.424137889235,13.9200415849572,31.));
#97124=CARTESIAN_POINT('Ctrl Pts',(111.424137889235,13.9200415849572,26.));
#97125=CARTESIAN_POINT('Ctrl Pts',(111.399377689205,13.9420348180159,31.));
#97126=CARTESIAN_POINT('Ctrl Pts',(111.399377689205,13.9420348180159,26.));
#97127=CARTESIAN_POINT('Ctrl Pts',(111.375358986128,13.9640809956577,31.));
#97128=CARTESIAN_POINT('Ctrl Pts',(111.375358986128,13.9640809956577,26.));
#97129=CARTESIAN_POINT('Ctrl Pts',(111.352083296364,13.9861647449775,31.));
#97130=CARTESIAN_POINT('Ctrl Pts',(111.352083296364,13.9861647449775,26.));
#97131=CARTESIAN_POINT('Ctrl Pts',(111.329553671008,14.0082647457932,31.));
#97132=CARTESIAN_POINT('Ctrl Pts',(111.329553671008,14.0082647457932,26.));
#97133=CARTESIAN_POINT('Ctrl Pts',(111.307775912141,14.0303529759501,31.));
#97134=CARTESIAN_POINT('Ctrl Pts',(111.307775912141,14.0303529759501,26.));
#97135=CARTESIAN_POINT('Ctrl Pts',(111.286760291356,14.052392594348,31.));
#97136=CARTESIAN_POINT('Ctrl Pts',(111.286760291356,14.052392594348,26.));
#97137=CARTESIAN_POINT('Ctrl Pts',(111.266520462056,14.0743413028629,31.));
#97138=CARTESIAN_POINT('Ctrl Pts',(111.266520462056,14.0743413028629,26.));
#97139=CARTESIAN_POINT('Ctrl Pts',(111.24707067242,14.0961578383154,31.));
#97140=CARTESIAN_POINT('Ctrl Pts',(111.24707067242,14.0961578383154,26.));
#97141=CARTESIAN_POINT('Ctrl Pts',(111.228423068787,14.1178081861225,31.));
#97142=CARTESIAN_POINT('Ctrl Pts',(111.228423068787,14.1178081861225,26.));
#97143=CARTESIAN_POINT('Ctrl Pts',(111.210585385968,14.1392705460289,31.));
#97144=CARTESIAN_POINT('Ctrl Pts',(111.210585385968,14.1392705460289,26.));
#97145=CARTESIAN_POINT('Ctrl Pts',(111.193556777481,14.1605444661444,31.));
#97146=CARTESIAN_POINT('Ctrl Pts',(111.193556777481,14.1605444661444,26.));
#97147=CARTESIAN_POINT('Ctrl Pts',(111.177330271158,14.1816440780432,31.));
#97148=CARTESIAN_POINT('Ctrl Pts',(111.177330271158,14.1816440780432,26.));
#97149=CARTESIAN_POINT('Ctrl Pts',(111.161900815541,14.2025779775787,31.));
#97150=CARTESIAN_POINT('Ctrl Pts',(111.161900815541,14.2025779775787,26.));
#97151=CARTESIAN_POINT('Ctrl Pts',(111.14727205821,14.2233316663202,31.));
#97152=CARTESIAN_POINT('Ctrl Pts',(111.14727205821,14.2233316663202,26.));
#97153=CARTESIAN_POINT('Ctrl Pts',(111.133462520623,14.2438514914768,31.));
#97154=CARTESIAN_POINT('Ctrl Pts',(111.133462520623,14.2438514914768,26.));
#97155=CARTESIAN_POINT('Ctrl Pts',(111.120514421203,14.2640211918315,31.));
#97156=CARTESIAN_POINT('Ctrl Pts',(111.120514421203,14.2640211918315,26.));
#97157=CARTESIAN_POINT('Ctrl Pts',(111.108490994798,14.2836686506361,31.));
#97158=CARTESIAN_POINT('Ctrl Pts',(111.108490994798,14.2836686506361,26.));
#97159=CARTESIAN_POINT('Ctrl Pts',(111.097464566465,14.3025969156895,31.));
#97160=CARTESIAN_POINT('Ctrl Pts',(111.097464566465,14.3025969156895,26.));
#97161=CARTESIAN_POINT('Ctrl Pts',(111.087506711152,14.3206092292363,31.));
#97162=CARTESIAN_POINT('Ctrl Pts',(111.087506711152,14.3206092292363,26.));
#97163=CARTESIAN_POINT('Ctrl Pts',(111.078678375617,14.3375342353121,31.));
#97164=CARTESIAN_POINT('Ctrl Pts',(111.078678375617,14.3375342353121,26.));
#97165=CARTESIAN_POINT('Ctrl Pts',(111.07101716314,14.3532574284428,31.));
#97166=CARTESIAN_POINT('Ctrl Pts',(111.07101716314,14.3532574284428,26.));
#97167=CARTESIAN_POINT('Ctrl Pts',(111.064539259202,14.3677182209748,31.));
#97168=CARTESIAN_POINT('Ctrl Pts',(111.064539259202,14.3677182209748,26.));
#97169=CARTESIAN_POINT('Ctrl Pts',(111.060306283432,14.3782565643212,31.));
#97170=CARTESIAN_POINT('Ctrl Pts',(111.060306283432,14.3782565643212,26.));
#97171=CARTESIAN_POINT('Ctrl Pts',(111.057664061419,14.3855792208451,31.));
#97172=CARTESIAN_POINT('Ctrl Pts',(111.057664061419,14.3855792208451,26.));
#97173=CARTESIAN_POINT('Ctrl Pts',(111.056138828999,14.3902031778294,31.));
#97174=CARTESIAN_POINT('Ctrl Pts',(111.056138828999,14.3902031778294,26.));
#97175=CARTESIAN_POINT('Ctrl Pts',(111.055435274693,14.3924507036097,31.));
#97176=CARTESIAN_POINT('Ctrl Pts',(111.055435274693,14.3924507036097,26.));
#97177=CARTESIAN_POINT('',(111.588247845187,13.7895999261044,31.));
#97178=CARTESIAN_POINT('Ctrl Pts',(111.055435274693,14.3924507036097,31.));
#97179=CARTESIAN_POINT('Ctrl Pts',(111.056138828999,14.3902031778294,31.));
#97180=CARTESIAN_POINT('Ctrl Pts',(111.057664061419,14.3855792208451,31.));
#97181=CARTESIAN_POINT('Ctrl Pts',(111.060306283432,14.3782565643212,31.));
#97182=CARTESIAN_POINT('Ctrl Pts',(111.064539259202,14.3677182209748,31.));
#97183=CARTESIAN_POINT('Ctrl Pts',(111.07101716314,14.3532574284428,31.));
#97184=CARTESIAN_POINT('Ctrl Pts',(111.078678375617,14.3375342353121,31.));
#97185=CARTESIAN_POINT('Ctrl Pts',(111.087506711152,14.3206092292363,31.));
#97186=CARTESIAN_POINT('Ctrl Pts',(111.097464566465,14.3025969156895,31.));
#97187=CARTESIAN_POINT('Ctrl Pts',(111.108490994798,14.2836686506361,31.));
#97188=CARTESIAN_POINT('Ctrl Pts',(111.120514421203,14.2640211918315,31.));
#97189=CARTESIAN_POINT('Ctrl Pts',(111.133462520623,14.2438514914768,31.));
#97190=CARTESIAN_POINT('Ctrl Pts',(111.14727205821,14.2233316663202,31.));
#97191=CARTESIAN_POINT('Ctrl Pts',(111.161900815541,14.2025779775787,31.));
#97192=CARTESIAN_POINT('Ctrl Pts',(111.177330271158,14.1816440780432,31.));
#97193=CARTESIAN_POINT('Ctrl Pts',(111.193556777481,14.1605444661444,31.));
#97194=CARTESIAN_POINT('Ctrl Pts',(111.210585385968,14.1392705460289,31.));
#97195=CARTESIAN_POINT('Ctrl Pts',(111.228423068787,14.1178081861225,31.));
#97196=CARTESIAN_POINT('Ctrl Pts',(111.24707067242,14.0961578383154,31.));
#97197=CARTESIAN_POINT('Ctrl Pts',(111.266520462056,14.0743413028629,31.));
#97198=CARTESIAN_POINT('Ctrl Pts',(111.286760291356,14.052392594348,31.));
#97199=CARTESIAN_POINT('Ctrl Pts',(111.307775912141,14.0303529759501,31.));
#97200=CARTESIAN_POINT('Ctrl Pts',(111.329553671008,14.0082647457932,31.));
#97201=CARTESIAN_POINT('Ctrl Pts',(111.352083296364,13.9861647449775,31.));
#97202=CARTESIAN_POINT('Ctrl Pts',(111.375358986128,13.9640809956577,31.));
#97203=CARTESIAN_POINT('Ctrl Pts',(111.399377689205,13.9420348180159,31.));
#97204=CARTESIAN_POINT('Ctrl Pts',(111.424137889235,13.9200415849572,31.));
#97205=CARTESIAN_POINT('Ctrl Pts',(111.44963814143,13.8981119641531,31.));
#97206=CARTESIAN_POINT('Ctrl Pts',(111.475875310414,13.8762529259845,31.));
#97207=CARTESIAN_POINT('Ctrl Pts',(111.502843526855,13.8544687325429,31.));
#97208=CARTESIAN_POINT('Ctrl Pts',(111.530536039611,13.8327615614272,31.));
#97209=CARTESIAN_POINT('Ctrl Pts',(111.553264364073,13.8154580515946,31.));
#97210=CARTESIAN_POINT('Ctrl Pts',(111.570631528299,13.80251540703,31.));
#97211=CARTESIAN_POINT('Ctrl Pts',(111.582352010706,13.7939024994014,31.));
#97212=CARTESIAN_POINT('Ctrl Pts',(111.588247845187,13.7895999261044,31.));
#97213=CARTESIAN_POINT('',(111.588247845187,13.7895999261044,26.));
#97214=CARTESIAN_POINT('Ctrl Pts',(111.588247845187,13.7895999261044,26.));
#97215=CARTESIAN_POINT('Ctrl Pts',(111.582352010706,13.7939024994014,26.));
#97216=CARTESIAN_POINT('Ctrl Pts',(111.570631528299,13.80251540703,26.));
#97217=CARTESIAN_POINT('Ctrl Pts',(111.553264364073,13.8154580515946,26.));
#97218=CARTESIAN_POINT('Ctrl Pts',(111.530536039611,13.8327615614272,26.));
#97219=CARTESIAN_POINT('Ctrl Pts',(111.502843526855,13.8544687325429,26.));
#97220=CARTESIAN_POINT('Ctrl Pts',(111.475875310414,13.8762529259845,26.));
#97221=CARTESIAN_POINT('Ctrl Pts',(111.44963814143,13.8981119641531,26.));
#97222=CARTESIAN_POINT('Ctrl Pts',(111.424137889235,13.9200415849572,26.));
#97223=CARTESIAN_POINT('Ctrl Pts',(111.399377689205,13.9420348180159,26.));
#97224=CARTESIAN_POINT('Ctrl Pts',(111.375358986128,13.9640809956577,26.));
#97225=CARTESIAN_POINT('Ctrl Pts',(111.352083296364,13.9861647449775,26.));
#97226=CARTESIAN_POINT('Ctrl Pts',(111.329553671008,14.0082647457932,26.));
#97227=CARTESIAN_POINT('Ctrl Pts',(111.307775912141,14.0303529759501,26.));
#97228=CARTESIAN_POINT('Ctrl Pts',(111.286760291356,14.052392594348,26.));
#97229=CARTESIAN_POINT('Ctrl Pts',(111.266520462056,14.0743413028629,26.));
#97230=CARTESIAN_POINT('Ctrl Pts',(111.24707067242,14.0961578383154,26.));
#97231=CARTESIAN_POINT('Ctrl Pts',(111.228423068787,14.1178081861225,26.));
#97232=CARTESIAN_POINT('Ctrl Pts',(111.210585385968,14.1392705460289,26.));
#97233=CARTESIAN_POINT('Ctrl Pts',(111.193556777481,14.1605444661444,26.));
#97234=CARTESIAN_POINT('Ctrl Pts',(111.177330271158,14.1816440780432,26.));
#97235=CARTESIAN_POINT('Ctrl Pts',(111.161900815541,14.2025779775787,26.));
#97236=CARTESIAN_POINT('Ctrl Pts',(111.14727205821,14.2233316663202,26.));
#97237=CARTESIAN_POINT('Ctrl Pts',(111.133462520623,14.2438514914768,26.));
#97238=CARTESIAN_POINT('Ctrl Pts',(111.120514421203,14.2640211918315,26.));
#97239=CARTESIAN_POINT('Ctrl Pts',(111.108490994798,14.2836686506361,26.));
#97240=CARTESIAN_POINT('Ctrl Pts',(111.097464566465,14.3025969156895,26.));
#97241=CARTESIAN_POINT('Ctrl Pts',(111.087506711152,14.3206092292363,26.));
#97242=CARTESIAN_POINT('Ctrl Pts',(111.078678375617,14.3375342353121,26.));
#97243=CARTESIAN_POINT('Ctrl Pts',(111.07101716314,14.3532574284428,26.));
#97244=CARTESIAN_POINT('Ctrl Pts',(111.064539259202,14.3677182209748,26.));
#97245=CARTESIAN_POINT('Ctrl Pts',(111.060306283432,14.3782565643212,26.));
#97246=CARTESIAN_POINT('Ctrl Pts',(111.057664061419,14.3855792208451,26.));
#97247=CARTESIAN_POINT('Ctrl Pts',(111.056138828999,14.3902031778294,26.));
#97248=CARTESIAN_POINT('Ctrl Pts',(111.055435274693,14.3924507036097,26.));
#97249=CARTESIAN_POINT('',(111.588247845187,13.7895999261044,31.));
#97250=CARTESIAN_POINT('Origin',(109.999999999999,18.0000000000028,31.));
#97251=CARTESIAN_POINT('',(111.854141622223,13.8997367347037,31.));
#97252=CARTESIAN_POINT('Origin',(109.999999999999,18.0000000000028,31.));
#97253=CARTESIAN_POINT('',(111.854141622223,13.8997367347037,26.));
#97254=CARTESIAN_POINT('Origin',(109.999999999999,18.0000000000028,26.));
#97255=CARTESIAN_POINT('',(111.854141622223,13.8997367347037,31.));
#97256=CARTESIAN_POINT('Ctrl Pts',(111.804617131104,14.702771989219,31.));
#97257=CARTESIAN_POINT('Ctrl Pts',(111.804617131104,14.702771989219,26.));
#97258=CARTESIAN_POINT('Ctrl Pts',(111.805708883808,14.7006852604798,31.));
#97259=CARTESIAN_POINT('Ctrl Pts',(111.805708883808,14.7006852604798,26.));
#97260=CARTESIAN_POINT('Ctrl Pts',(111.807900012971,14.6963371269573,31.));
#97261=CARTESIAN_POINT('Ctrl Pts',(111.807900012971,14.6963371269573,26.));
#97262=CARTESIAN_POINT('Ctrl Pts',(111.811209579963,14.6892908937737,31.));
#97263=CARTESIAN_POINT('Ctrl Pts',(111.811209579963,14.6892908937737,26.));
#97264=CARTESIAN_POINT('Ctrl Pts',(111.815668148138,14.6788459938606,31.));
#97265=CARTESIAN_POINT('Ctrl Pts',(111.815668148138,14.6788459938606,26.));
#97266=CARTESIAN_POINT('Ctrl Pts',(111.82131290279,14.6640400995954,31.));
#97267=CARTESIAN_POINT('Ctrl Pts',(111.82131290279,14.6640400995954,26.));
#97268=CARTESIAN_POINT('Ctrl Pts',(111.827013583967,14.6475048278114,31.));
#97269=CARTESIAN_POINT('Ctrl Pts',(111.827013583967,14.6475048278114,26.));
#97270=CARTESIAN_POINT('Ctrl Pts',(111.832738794595,14.6292944653143,31.));
#97271=CARTESIAN_POINT('Ctrl Pts',(111.832738794595,14.6292944653143,26.));
#97272=CARTESIAN_POINT('Ctrl Pts',(111.838434156619,14.6095165692379,31.));
#97273=CARTESIAN_POINT('Ctrl Pts',(111.838434156619,14.6095165692379,26.));
#97274=CARTESIAN_POINT('Ctrl Pts',(111.844021598942,14.5883354024137,31.));
#97275=CARTESIAN_POINT('Ctrl Pts',(111.844021598942,14.5883354024137,26.));
#97276=CARTESIAN_POINT('Ctrl Pts',(111.849412603956,14.5659407047175,31.));
#97277=CARTESIAN_POINT('Ctrl Pts',(111.849412603956,14.5659407047175,26.));
#97278=CARTESIAN_POINT('Ctrl Pts',(111.85451904696,14.5425228839233,31.));
#97279=CARTESIAN_POINT('Ctrl Pts',(111.85451904696,14.5425228839233,26.));
#97280=CARTESIAN_POINT('Ctrl Pts',(111.859263936817,14.5182483587386,31.));
#97281=CARTESIAN_POINT('Ctrl Pts',(111.859263936817,14.5182483587386,26.));
#97282=CARTESIAN_POINT('Ctrl Pts',(111.863594917364,14.4932291911909,31.));
#97283=CARTESIAN_POINT('Ctrl Pts',(111.863594917364,14.4932291911909,26.));
#97284=CARTESIAN_POINT('Ctrl Pts',(111.867487146992,14.4675164161785,31.));
#97285=CARTESIAN_POINT('Ctrl Pts',(111.867487146992,14.4675164161785,26.));
#97286=CARTESIAN_POINT('Ctrl Pts',(111.870932952987,14.4411228648671,31.));
#97287=CARTESIAN_POINT('Ctrl Pts',(111.870932952987,14.4411228648671,26.));
#97288=CARTESIAN_POINT('Ctrl Pts',(111.873934841617,14.4140388871515,31.));
#97289=CARTESIAN_POINT('Ctrl Pts',(111.873934841617,14.4140388871515,26.));
#97290=CARTESIAN_POINT('Ctrl Pts',(111.876497875346,14.3862495604319,31.));
#97291=CARTESIAN_POINT('Ctrl Pts',(111.876497875346,14.3862495604319,26.));
#97292=CARTESIAN_POINT('Ctrl Pts',(111.878621136093,14.3577546056918,31.));
#97293=CARTESIAN_POINT('Ctrl Pts',(111.878621136093,14.3577546056918,26.));
#97294=CARTESIAN_POINT('Ctrl Pts',(111.880294678097,14.3285749073818,31.));
#97295=CARTESIAN_POINT('Ctrl Pts',(111.880294678097,14.3285749073818,26.));
#97296=CARTESIAN_POINT('Ctrl Pts',(111.881503038178,14.2987431062045,31.));
#97297=CARTESIAN_POINT('Ctrl Pts',(111.881503038178,14.2987431062045,26.));
#97298=CARTESIAN_POINT('Ctrl Pts',(111.882227113853,14.2682984546204,31.));
#97299=CARTESIAN_POINT('Ctrl Pts',(111.882227113853,14.2682984546204,26.));
#97300=CARTESIAN_POINT('Ctrl Pts',(111.882446650243,14.2372805163331,31.));
#97301=CARTESIAN_POINT('Ctrl Pts',(111.882446650243,14.2372805163331,26.));
#97302=CARTESIAN_POINT('Ctrl Pts',(111.882142859859,14.2057226050428,31.));
#97303=CARTESIAN_POINT('Ctrl Pts',(111.882142859859,14.2057226050428,26.));
#97304=CARTESIAN_POINT('Ctrl Pts',(111.881300030722,14.1736486380898,31.));
#97305=CARTESIAN_POINT('Ctrl Pts',(111.881300030722,14.1736486380898,26.));
#97306=CARTESIAN_POINT('Ctrl Pts',(111.879905244617,14.1410758485617,31.));
#97307=CARTESIAN_POINT('Ctrl Pts',(111.879905244617,14.1410758485617,26.));
#97308=CARTESIAN_POINT('Ctrl Pts',(111.877948703475,14.1080161789671,31.));
#97309=CARTESIAN_POINT('Ctrl Pts',(111.877948703475,14.1080161789671,26.));
#97310=CARTESIAN_POINT('Ctrl Pts',(111.87542388573,14.074478194107,31.));
#97311=CARTESIAN_POINT('Ctrl Pts',(111.87542388573,14.074478194107,26.));
#97312=CARTESIAN_POINT('Ctrl Pts',(111.872328079638,14.0404690398371,31.));
#97313=CARTESIAN_POINT('Ctrl Pts',(111.872328079638,14.0404690398371,26.));
#97314=CARTESIAN_POINT('Ctrl Pts',(111.868662421724,14.0059958801699,31.));
#97315=CARTESIAN_POINT('Ctrl Pts',(111.868662421724,14.0059958801699,26.));
#97316=CARTESIAN_POINT('Ctrl Pts',(111.864430146015,13.9710650286956,31.));
#97317=CARTESIAN_POINT('Ctrl Pts',(111.864430146015,13.9710650286956,26.));
#97318=CARTESIAN_POINT('Ctrl Pts',(111.860594222842,13.9427582472186,31.));
#97319=CARTESIAN_POINT('Ctrl Pts',(111.860594222842,13.9427582472186,26.));
#97320=CARTESIAN_POINT('Ctrl Pts',(111.857465615073,13.9213259759228,31.));
#97321=CARTESIAN_POINT('Ctrl Pts',(111.857465615073,13.9213259759228,26.));
#97322=CARTESIAN_POINT('Ctrl Pts',(111.85526822796,13.9069480979796,31.));
#97323=CARTESIAN_POINT('Ctrl Pts',(111.85526822796,13.9069480979796,26.));
#97324=CARTESIAN_POINT('Ctrl Pts',(111.854141622223,13.8997367347037,31.));
#97325=CARTESIAN_POINT('Ctrl Pts',(111.854141622223,13.8997367347037,26.));
#97326=CARTESIAN_POINT('Ctrl Pts',(111.804617131104,14.702771989219,31.));
#97327=CARTESIAN_POINT('Ctrl Pts',(111.805708883808,14.7006852604798,31.));
#97328=CARTESIAN_POINT('Ctrl Pts',(111.807900012971,14.6963371269573,31.));
#97329=CARTESIAN_POINT('Ctrl Pts',(111.811209579963,14.6892908937737,31.));
#97330=CARTESIAN_POINT('Ctrl Pts',(111.815668148138,14.6788459938606,31.));
#97331=CARTESIAN_POINT('Ctrl Pts',(111.82131290279,14.6640400995954,31.));
#97332=CARTESIAN_POINT('Ctrl Pts',(111.827013583967,14.6475048278114,31.));
#97333=CARTESIAN_POINT('Ctrl Pts',(111.832738794595,14.6292944653143,31.));
#97334=CARTESIAN_POINT('Ctrl Pts',(111.838434156619,14.6095165692379,31.));
#97335=CARTESIAN_POINT('Ctrl Pts',(111.844021598942,14.5883354024137,31.));
#97336=CARTESIAN_POINT('Ctrl Pts',(111.849412603956,14.5659407047175,31.));
#97337=CARTESIAN_POINT('Ctrl Pts',(111.85451904696,14.5425228839233,31.));
#97338=CARTESIAN_POINT('Ctrl Pts',(111.859263936817,14.5182483587386,31.));
#97339=CARTESIAN_POINT('Ctrl Pts',(111.863594917364,14.4932291911909,31.));
#97340=CARTESIAN_POINT('Ctrl Pts',(111.867487146992,14.4675164161785,31.));
#97341=CARTESIAN_POINT('Ctrl Pts',(111.870932952987,14.4411228648671,31.));
#97342=CARTESIAN_POINT('Ctrl Pts',(111.873934841617,14.4140388871515,31.));
#97343=CARTESIAN_POINT('Ctrl Pts',(111.876497875346,14.3862495604319,31.));
#97344=CARTESIAN_POINT('Ctrl Pts',(111.878621136093,14.3577546056918,31.));
#97345=CARTESIAN_POINT('Ctrl Pts',(111.880294678097,14.3285749073818,31.));
#97346=CARTESIAN_POINT('Ctrl Pts',(111.881503038178,14.2987431062045,31.));
#97347=CARTESIAN_POINT('Ctrl Pts',(111.882227113853,14.2682984546204,31.));
#97348=CARTESIAN_POINT('Ctrl Pts',(111.882446650243,14.2372805163331,31.));
#97349=CARTESIAN_POINT('Ctrl Pts',(111.882142859859,14.2057226050428,31.));
#97350=CARTESIAN_POINT('Ctrl Pts',(111.881300030722,14.1736486380898,31.));
#97351=CARTESIAN_POINT('Ctrl Pts',(111.879905244617,14.1410758485617,31.));
#97352=CARTESIAN_POINT('Ctrl Pts',(111.877948703475,14.1080161789671,31.));
#97353=CARTESIAN_POINT('Ctrl Pts',(111.87542388573,14.074478194107,31.));
#97354=CARTESIAN_POINT('Ctrl Pts',(111.872328079638,14.0404690398371,31.));
#97355=CARTESIAN_POINT('Ctrl Pts',(111.868662421724,14.0059958801699,31.));
#97356=CARTESIAN_POINT('Ctrl Pts',(111.864430146015,13.9710650286956,31.));
#97357=CARTESIAN_POINT('Ctrl Pts',(111.860594222842,13.9427582472186,31.));
#97358=CARTESIAN_POINT('Ctrl Pts',(111.857465615073,13.9213259759228,31.));
#97359=CARTESIAN_POINT('Ctrl Pts',(111.85526822796,13.9069480979796,31.));
#97360=CARTESIAN_POINT('Ctrl Pts',(111.854141622223,13.8997367347037,31.));
#97361=CARTESIAN_POINT('Ctrl Pts',(111.804617131104,14.702771989219,26.));
#97362=CARTESIAN_POINT('Ctrl Pts',(111.805708883808,14.7006852604798,26.));
#97363=CARTESIAN_POINT('Ctrl Pts',(111.807900012971,14.6963371269573,26.));
#97364=CARTESIAN_POINT('Ctrl Pts',(111.811209579963,14.6892908937737,26.));
#97365=CARTESIAN_POINT('Ctrl Pts',(111.815668148138,14.6788459938606,26.));
#97366=CARTESIAN_POINT('Ctrl Pts',(111.82131290279,14.6640400995954,26.));
#97367=CARTESIAN_POINT('Ctrl Pts',(111.827013583967,14.6475048278114,26.));
#97368=CARTESIAN_POINT('Ctrl Pts',(111.832738794595,14.6292944653143,26.));
#97369=CARTESIAN_POINT('Ctrl Pts',(111.838434156619,14.6095165692379,26.));
#97370=CARTESIAN_POINT('Ctrl Pts',(111.844021598942,14.5883354024137,26.));
#97371=CARTESIAN_POINT('Ctrl Pts',(111.849412603956,14.5659407047175,26.));
#97372=CARTESIAN_POINT('Ctrl Pts',(111.85451904696,14.5425228839233,26.));
#97373=CARTESIAN_POINT('Ctrl Pts',(111.859263936817,14.5182483587386,26.));
#97374=CARTESIAN_POINT('Ctrl Pts',(111.863594917364,14.4932291911909,26.));
#97375=CARTESIAN_POINT('Ctrl Pts',(111.867487146992,14.4675164161785,26.));
#97376=CARTESIAN_POINT('Ctrl Pts',(111.870932952987,14.4411228648671,26.));
#97377=CARTESIAN_POINT('Ctrl Pts',(111.873934841617,14.4140388871515,26.));
#97378=CARTESIAN_POINT('Ctrl Pts',(111.876497875346,14.3862495604319,26.));
#97379=CARTESIAN_POINT('Ctrl Pts',(111.878621136093,14.3577546056918,26.));
#97380=CARTESIAN_POINT('Ctrl Pts',(111.880294678097,14.3285749073818,26.));
#97381=CARTESIAN_POINT('Ctrl Pts',(111.881503038178,14.2987431062045,26.));
#97382=CARTESIAN_POINT('Ctrl Pts',(111.882227113853,14.2682984546204,26.));
#97383=CARTESIAN_POINT('Ctrl Pts',(111.882446650243,14.2372805163331,26.));
#97384=CARTESIAN_POINT('Ctrl Pts',(111.882142859859,14.2057226050428,26.));
#97385=CARTESIAN_POINT('Ctrl Pts',(111.881300030722,14.1736486380898,26.));
#97386=CARTESIAN_POINT('Ctrl Pts',(111.879905244617,14.1410758485617,26.));
#97387=CARTESIAN_POINT('Ctrl Pts',(111.877948703475,14.1080161789671,26.));
#97388=CARTESIAN_POINT('Ctrl Pts',(111.87542388573,14.074478194107,26.));
#97389=CARTESIAN_POINT('Ctrl Pts',(111.872328079638,14.0404690398371,26.));
#97390=CARTESIAN_POINT('Ctrl Pts',(111.868662421724,14.0059958801699,26.));
#97391=CARTESIAN_POINT('Ctrl Pts',(111.864430146015,13.9710650286956,26.));
#97392=CARTESIAN_POINT('Ctrl Pts',(111.860594222842,13.9427582472186,26.));
#97393=CARTESIAN_POINT('Ctrl Pts',(111.857465615073,13.9213259759228,26.));
#97394=CARTESIAN_POINT('Ctrl Pts',(111.85526822796,13.9069480979796,26.));
#97395=CARTESIAN_POINT('Ctrl Pts',(111.854141622223,13.8997367347037,26.));
#97396=CARTESIAN_POINT('Origin',(111.474514194069,14.4402078348085,31.));
#97397=CARTESIAN_POINT('Origin',(109.59454570101,14.2631614489809,31.));
#97398=CARTESIAN_POINT('',(109.59454570101,14.2631614489809,26.));
#97399=CARTESIAN_POINT('',(109.652122916228,14.7938174514562,26.));
#97400=CARTESIAN_POINT('',(109.59454570101,14.2631614489809,31.));
#97401=CARTESIAN_POINT('',(109.59454570101,14.2631614489809,31.));
#97402=CARTESIAN_POINT('',(109.652122916228,14.7938174514562,31.));
#97403=CARTESIAN_POINT('Ctrl Pts',(109.856099324815,13.5023014112014,31.));
#97404=CARTESIAN_POINT('Ctrl Pts',(109.856099324815,13.5023014112014,26.));
#97405=CARTESIAN_POINT('Ctrl Pts',(109.852298807528,13.5085327087832,31.));
#97406=CARTESIAN_POINT('Ctrl Pts',(109.852298807528,13.5085327087832,26.));
#97407=CARTESIAN_POINT('Ctrl Pts',(109.844766510775,13.5209752322934,31.));
#97408=CARTESIAN_POINT('Ctrl Pts',(109.844766510775,13.5209752322934,26.));
#97409=CARTESIAN_POINT('Ctrl Pts',(109.833674278855,13.5395788027196,31.));
#97410=CARTESIAN_POINT('Ctrl Pts',(109.833674278855,13.5395788027196,26.));
#97411=CARTESIAN_POINT('Ctrl Pts',(109.819297811611,13.5642629145113,31.));
#97412=CARTESIAN_POINT('Ctrl Pts',(109.819297811611,13.5642629145113,26.));
#97413=CARTESIAN_POINT('Ctrl Pts',(109.802020240621,13.5949151914465,31.));
#97414=CARTESIAN_POINT('Ctrl Pts',(109.802020240621,13.5949151914465,26.));
#97415=CARTESIAN_POINT('Ctrl Pts',(109.785441307341,13.6253614515315,31.));
#97416=CARTESIAN_POINT('Ctrl Pts',(109.785441307341,13.6253614515315,26.));
#97417=CARTESIAN_POINT('Ctrl Pts',(109.76956641568,13.6555970993782,31.));
#97418=CARTESIAN_POINT('Ctrl Pts',(109.76956641568,13.6555970993782,26.));
#97419=CARTESIAN_POINT('Ctrl Pts',(109.754399357163,13.685615951231,31.));
#97420=CARTESIAN_POINT('Ctrl Pts',(109.754399357163,13.685615951231,26.));
#97421=CARTESIAN_POINT('Ctrl Pts',(109.73994036105,13.7154103674413,31.));
#97422=CARTESIAN_POINT('Ctrl Pts',(109.73994036105,13.7154103674413,26.));
#97423=CARTESIAN_POINT('Ctrl Pts',(109.72618667981,13.7449699394692,31.));
#97424=CARTESIAN_POINT('Ctrl Pts',(109.72618667981,13.7449699394692,26.));
#97425=CARTESIAN_POINT('Ctrl Pts',(109.713133831421,13.7742798843163,31.));
#97426=CARTESIAN_POINT('Ctrl Pts',(109.713133831421,13.7742798843163,26.));
#97427=CARTESIAN_POINT('Ctrl Pts',(109.700776475847,13.8033193370997,31.));
#97428=CARTESIAN_POINT('Ctrl Pts',(109.700776475847,13.8033193370997,26.));
#97429=CARTESIAN_POINT('Ctrl Pts',(109.689109249897,13.8320601883634,31.));
#97430=CARTESIAN_POINT('Ctrl Pts',(109.689109249897,13.8320601883634,26.));
#97431=CARTESIAN_POINT('Ctrl Pts',(109.678127544808,13.8604644706008,31.));
#97432=CARTESIAN_POINT('Ctrl Pts',(109.678127544808,13.8604644706008,26.));
#97433=CARTESIAN_POINT('Ctrl Pts',(109.667827787886,13.8884878805099,31.));
#97434=CARTESIAN_POINT('Ctrl Pts',(109.667827787886,13.8884878805099,26.));
#97435=CARTESIAN_POINT('Ctrl Pts',(109.658207351999,13.9160868433413,31.));
#97436=CARTESIAN_POINT('Ctrl Pts',(109.658207351999,13.9160868433413,26.));
#97437=CARTESIAN_POINT('Ctrl Pts',(109.649264442082,13.943225285516,31.));
#97438=CARTESIAN_POINT('Ctrl Pts',(109.649264442082,13.943225285516,26.));
#97439=CARTESIAN_POINT('Ctrl Pts',(109.640997861574,13.9698801062394,31.));
#97440=CARTESIAN_POINT('Ctrl Pts',(109.640997861574,13.9698801062394,26.));
#97441=CARTESIAN_POINT('Ctrl Pts',(109.633406655496,13.9960512119544,31.));
#97442=CARTESIAN_POINT('Ctrl Pts',(109.633406655496,13.9960512119544,26.));
#97443=CARTESIAN_POINT('Ctrl Pts',(109.626489790322,14.021754326667,31.));
#97444=CARTESIAN_POINT('Ctrl Pts',(109.626489790322,14.021754326667,26.));
#97445=CARTESIAN_POINT('Ctrl Pts',(109.620245888607,14.0469993250184,31.));
#97446=CARTESIAN_POINT('Ctrl Pts',(109.620245888607,14.0469993250184,26.));
#97447=CARTESIAN_POINT('Ctrl Pts',(109.614672771965,14.0717714163373,31.));
#97448=CARTESIAN_POINT('Ctrl Pts',(109.614672771965,14.0717714163373,26.));
#97449=CARTESIAN_POINT('Ctrl Pts',(109.609767019958,14.0960139440534,31.));
#97450=CARTESIAN_POINT('Ctrl Pts',(109.609767019958,14.0960139440534,26.));
#97451=CARTESIAN_POINT('Ctrl Pts',(109.60552314608,14.1196033405166,31.));
#97452=CARTESIAN_POINT('Ctrl Pts',(109.60552314608,14.1196033405166,26.));
#97453=CARTESIAN_POINT('Ctrl Pts',(109.601933705487,14.1423563916575,31.));
#97454=CARTESIAN_POINT('Ctrl Pts',(109.601933705487,14.1423563916575,26.));
#97455=CARTESIAN_POINT('Ctrl Pts',(109.598990147472,14.1640634597676,31.));
#97456=CARTESIAN_POINT('Ctrl Pts',(109.598990147472,14.1640634597676,26.));
#97457=CARTESIAN_POINT('Ctrl Pts',(109.596683302734,14.1845153738368,31.));
#97458=CARTESIAN_POINT('Ctrl Pts',(109.596683302734,14.1845153738368,26.));
#97459=CARTESIAN_POINT('Ctrl Pts',(109.595003903645,14.2035304982823,31.));
#97460=CARTESIAN_POINT('Ctrl Pts',(109.595003903645,14.2035304982823,26.));
#97461=CARTESIAN_POINT('Ctrl Pts',(109.593942871758,14.2209886536882,31.));
#97462=CARTESIAN_POINT('Ctrl Pts',(109.593942871758,14.2209886536882,26.));
#97463=CARTESIAN_POINT('Ctrl Pts',(109.593491974617,14.2368276704459,31.));
#97464=CARTESIAN_POINT('Ctrl Pts',(109.593491974617,14.2368276704459,26.));
#97465=CARTESIAN_POINT('Ctrl Pts',(109.593614064345,14.2481837198673,31.));
#97466=CARTESIAN_POINT('Ctrl Pts',(109.593614064345,14.2481837198673,26.));
#97467=CARTESIAN_POINT('Ctrl Pts',(109.593975228839,14.2559601069423,31.));
#97468=CARTESIAN_POINT('Ctrl Pts',(109.593975228839,14.2559601069423,26.));
#97469=CARTESIAN_POINT('Ctrl Pts',(109.594335609554,14.2608157673368,31.));
#97470=CARTESIAN_POINT('Ctrl Pts',(109.594335609554,14.2608157673368,26.));
#97471=CARTESIAN_POINT('Ctrl Pts',(109.59454570101,14.2631614489809,31.));
#97472=CARTESIAN_POINT('Ctrl Pts',(109.59454570101,14.2631614489809,26.));
#97473=CARTESIAN_POINT('',(109.856099324815,13.5023014112014,31.));
#97474=CARTESIAN_POINT('Ctrl Pts',(109.59454570101,14.2631614489809,31.));
#97475=CARTESIAN_POINT('Ctrl Pts',(109.594335609554,14.2608157673368,31.));
#97476=CARTESIAN_POINT('Ctrl Pts',(109.593975228839,14.2559601069423,31.));
#97477=CARTESIAN_POINT('Ctrl Pts',(109.593614064345,14.2481837198673,31.));
#97478=CARTESIAN_POINT('Ctrl Pts',(109.593491974617,14.2368276704459,31.));
#97479=CARTESIAN_POINT('Ctrl Pts',(109.593942871758,14.2209886536882,31.));
#97480=CARTESIAN_POINT('Ctrl Pts',(109.595003903645,14.2035304982823,31.));
#97481=CARTESIAN_POINT('Ctrl Pts',(109.596683302734,14.1845153738368,31.));
#97482=CARTESIAN_POINT('Ctrl Pts',(109.598990147472,14.1640634597676,31.));
#97483=CARTESIAN_POINT('Ctrl Pts',(109.601933705487,14.1423563916575,31.));
#97484=CARTESIAN_POINT('Ctrl Pts',(109.60552314608,14.1196033405166,31.));
#97485=CARTESIAN_POINT('Ctrl Pts',(109.609767019958,14.0960139440534,31.));
#97486=CARTESIAN_POINT('Ctrl Pts',(109.614672771965,14.0717714163373,31.));
#97487=CARTESIAN_POINT('Ctrl Pts',(109.620245888607,14.0469993250184,31.));
#97488=CARTESIAN_POINT('Ctrl Pts',(109.626489790322,14.021754326667,31.));
#97489=CARTESIAN_POINT('Ctrl Pts',(109.633406655496,13.9960512119544,31.));
#97490=CARTESIAN_POINT('Ctrl Pts',(109.640997861574,13.9698801062394,31.));
#97491=CARTESIAN_POINT('Ctrl Pts',(109.649264442082,13.943225285516,31.));
#97492=CARTESIAN_POINT('Ctrl Pts',(109.658207351999,13.9160868433413,31.));
#97493=CARTESIAN_POINT('Ctrl Pts',(109.667827787886,13.8884878805099,31.));
#97494=CARTESIAN_POINT('Ctrl Pts',(109.678127544808,13.8604644706008,31.));
#97495=CARTESIAN_POINT('Ctrl Pts',(109.689109249897,13.8320601883634,31.));
#97496=CARTESIAN_POINT('Ctrl Pts',(109.700776475847,13.8033193370997,31.));
#97497=CARTESIAN_POINT('Ctrl Pts',(109.713133831421,13.7742798843163,31.));
#97498=CARTESIAN_POINT('Ctrl Pts',(109.72618667981,13.7449699394692,31.));
#97499=CARTESIAN_POINT('Ctrl Pts',(109.73994036105,13.7154103674413,31.));
#97500=CARTESIAN_POINT('Ctrl Pts',(109.754399357163,13.685615951231,31.));
#97501=CARTESIAN_POINT('Ctrl Pts',(109.76956641568,13.6555970993782,31.));
#97502=CARTESIAN_POINT('Ctrl Pts',(109.785441307341,13.6253614515315,31.));
#97503=CARTESIAN_POINT('Ctrl Pts',(109.802020240621,13.5949151914465,31.));
#97504=CARTESIAN_POINT('Ctrl Pts',(109.819297811611,13.5642629145113,31.));
#97505=CARTESIAN_POINT('Ctrl Pts',(109.833674278855,13.5395788027196,31.));
#97506=CARTESIAN_POINT('Ctrl Pts',(109.844766510775,13.5209752322934,31.));
#97507=CARTESIAN_POINT('Ctrl Pts',(109.852298807528,13.5085327087832,31.));
#97508=CARTESIAN_POINT('Ctrl Pts',(109.856099324815,13.5023014112014,31.));
#97509=CARTESIAN_POINT('',(109.856099324815,13.5023014112014,26.));
#97510=CARTESIAN_POINT('Ctrl Pts',(109.856099324815,13.5023014112014,26.));
#97511=CARTESIAN_POINT('Ctrl Pts',(109.852298807528,13.5085327087832,26.));
#97512=CARTESIAN_POINT('Ctrl Pts',(109.844766510775,13.5209752322934,26.));
#97513=CARTESIAN_POINT('Ctrl Pts',(109.833674278855,13.5395788027196,26.));
#97514=CARTESIAN_POINT('Ctrl Pts',(109.819297811611,13.5642629145113,26.));
#97515=CARTESIAN_POINT('Ctrl Pts',(109.802020240621,13.5949151914465,26.));
#97516=CARTESIAN_POINT('Ctrl Pts',(109.785441307341,13.6253614515315,26.));
#97517=CARTESIAN_POINT('Ctrl Pts',(109.76956641568,13.6555970993782,26.));
#97518=CARTESIAN_POINT('Ctrl Pts',(109.754399357163,13.685615951231,26.));
#97519=CARTESIAN_POINT('Ctrl Pts',(109.73994036105,13.7154103674413,26.));
#97520=CARTESIAN_POINT('Ctrl Pts',(109.72618667981,13.7449699394692,26.));
#97521=CARTESIAN_POINT('Ctrl Pts',(109.713133831421,13.7742798843163,26.));
#97522=CARTESIAN_POINT('Ctrl Pts',(109.700776475847,13.8033193370997,26.));
#97523=CARTESIAN_POINT('Ctrl Pts',(109.689109249897,13.8320601883634,26.));
#97524=CARTESIAN_POINT('Ctrl Pts',(109.678127544808,13.8604644706008,26.));
#97525=CARTESIAN_POINT('Ctrl Pts',(109.667827787886,13.8884878805099,26.));
#97526=CARTESIAN_POINT('Ctrl Pts',(109.658207351999,13.9160868433413,26.));
#97527=CARTESIAN_POINT('Ctrl Pts',(109.649264442082,13.943225285516,26.));
#97528=CARTESIAN_POINT('Ctrl Pts',(109.640997861574,13.9698801062394,26.));
#97529=CARTESIAN_POINT('Ctrl Pts',(109.633406655496,13.9960512119544,26.));
#97530=CARTESIAN_POINT('Ctrl Pts',(109.626489790322,14.021754326667,26.));
#97531=CARTESIAN_POINT('Ctrl Pts',(109.620245888607,14.0469993250184,26.));
#97532=CARTESIAN_POINT('Ctrl Pts',(109.614672771965,14.0717714163373,26.));
#97533=CARTESIAN_POINT('Ctrl Pts',(109.609767019958,14.0960139440534,26.));
#97534=CARTESIAN_POINT('Ctrl Pts',(109.60552314608,14.1196033405166,26.));
#97535=CARTESIAN_POINT('Ctrl Pts',(109.601933705487,14.1423563916575,26.));
#97536=CARTESIAN_POINT('Ctrl Pts',(109.598990147472,14.1640634597676,26.));
#97537=CARTESIAN_POINT('Ctrl Pts',(109.596683302734,14.1845153738368,26.));
#97538=CARTESIAN_POINT('Ctrl Pts',(109.595003903645,14.2035304982823,26.));
#97539=CARTESIAN_POINT('Ctrl Pts',(109.593942871758,14.2209886536882,26.));
#97540=CARTESIAN_POINT('Ctrl Pts',(109.593491974617,14.2368276704459,26.));
#97541=CARTESIAN_POINT('Ctrl Pts',(109.593614064345,14.2481837198673,26.));
#97542=CARTESIAN_POINT('Ctrl Pts',(109.593975228839,14.2559601069423,26.));
#97543=CARTESIAN_POINT('Ctrl Pts',(109.594335609554,14.2608157673368,26.));
#97544=CARTESIAN_POINT('Ctrl Pts',(109.59454570101,14.2631614489809,26.));
#97545=CARTESIAN_POINT('',(109.856099324815,13.5023014112014,31.));
#97546=CARTESIAN_POINT('Origin',(110.,18.000000000003,31.));
#97547=CARTESIAN_POINT('',(110.143900675185,13.5023014112014,31.));
#97548=CARTESIAN_POINT('Origin',(110.,18.000000000003,31.));
#97549=CARTESIAN_POINT('',(110.143900675185,13.5023014112014,26.));
#97550=CARTESIAN_POINT('Origin',(110.,18.000000000003,26.));
#97551=CARTESIAN_POINT('',(110.143900675185,13.5023014112014,31.));
#97552=CARTESIAN_POINT('Ctrl Pts',(110.40545429899,14.2631614489809,31.));
#97553=CARTESIAN_POINT('Ctrl Pts',(110.40545429899,14.2631614489809,26.));
#97554=CARTESIAN_POINT('Ctrl Pts',(110.405664390452,14.2608157673365,31.));
#97555=CARTESIAN_POINT('Ctrl Pts',(110.405664390452,14.2608157673365,26.));
#97556=CARTESIAN_POINT('Ctrl Pts',(110.406024771178,14.2559601069417,31.));
#97557=CARTESIAN_POINT('Ctrl Pts',(110.406024771178,14.2559601069417,26.));
#97558=CARTESIAN_POINT('Ctrl Pts',(110.406385935683,14.2481837198662,31.));
#97559=CARTESIAN_POINT('Ctrl Pts',(110.406385935683,14.2481837198662,26.));
#97560=CARTESIAN_POINT('Ctrl Pts',(110.406508025415,14.2368276704446,31.));
#97561=CARTESIAN_POINT('Ctrl Pts',(110.406508025415,14.2368276704446,26.));
#97562=CARTESIAN_POINT('Ctrl Pts',(110.406057128268,14.2209886536872,31.));
#97563=CARTESIAN_POINT('Ctrl Pts',(110.406057128268,14.2209886536872,26.));
#97564=CARTESIAN_POINT('Ctrl Pts',(110.404996096367,14.2035304982819,31.));
#97565=CARTESIAN_POINT('Ctrl Pts',(110.404996096367,14.2035304982819,26.));
#97566=CARTESIAN_POINT('Ctrl Pts',(110.40331669726,14.184515373837,31.));
#97567=CARTESIAN_POINT('Ctrl Pts',(110.40331669726,14.184515373837,26.));
#97568=CARTESIAN_POINT('Ctrl Pts',(110.401009852508,14.1640634597682,31.));
#97569=CARTESIAN_POINT('Ctrl Pts',(110.401009852508,14.1640634597682,26.));
#97570=CARTESIAN_POINT('Ctrl Pts',(110.398066294489,14.1423563916581,31.));
#97571=CARTESIAN_POINT('Ctrl Pts',(110.398066294489,14.1423563916581,26.));
#97572=CARTESIAN_POINT('Ctrl Pts',(110.3944768539,14.1196033405171,31.));
#97573=CARTESIAN_POINT('Ctrl Pts',(110.3944768539,14.1196033405171,26.));
#97574=CARTESIAN_POINT('Ctrl Pts',(110.390232980035,14.0960139440535,31.));
#97575=CARTESIAN_POINT('Ctrl Pts',(110.390232980035,14.0960139440535,26.));
#97576=CARTESIAN_POINT('Ctrl Pts',(110.385327228041,14.0717714163371,31.));
#97577=CARTESIAN_POINT('Ctrl Pts',(110.385327228041,14.0717714163371,26.));
#97578=CARTESIAN_POINT('Ctrl Pts',(110.379754111412,14.0469993250182,31.));
#97579=CARTESIAN_POINT('Ctrl Pts',(110.379754111412,14.0469993250182,26.));
#97580=CARTESIAN_POINT('Ctrl Pts',(110.373510209703,14.0217543266667,31.));
#97581=CARTESIAN_POINT('Ctrl Pts',(110.373510209703,14.0217543266667,26.));
#97582=CARTESIAN_POINT('Ctrl Pts',(110.366593344528,13.9960512119543,31.));
#97583=CARTESIAN_POINT('Ctrl Pts',(110.366593344528,13.9960512119543,26.));
#97584=CARTESIAN_POINT('Ctrl Pts',(110.359002138437,13.9698801062394,31.));
#97585=CARTESIAN_POINT('Ctrl Pts',(110.359002138437,13.9698801062394,26.));
#97586=CARTESIAN_POINT('Ctrl Pts',(110.350735557909,13.943225285516,31.));
#97587=CARTESIAN_POINT('Ctrl Pts',(110.350735557909,13.943225285516,26.));
#97588=CARTESIAN_POINT('Ctrl Pts',(110.34179264797,13.9160868433413,31.));
#97589=CARTESIAN_POINT('Ctrl Pts',(110.34179264797,13.9160868433413,26.));
#97590=CARTESIAN_POINT('Ctrl Pts',(110.332172212069,13.8884878805099,31.));
#97591=CARTESIAN_POINT('Ctrl Pts',(110.332172212069,13.8884878805099,26.));
#97592=CARTESIAN_POINT('Ctrl Pts',(110.321872455148,13.8604644706007,31.));
#97593=CARTESIAN_POINT('Ctrl Pts',(110.321872455148,13.8604644706007,26.));
#97594=CARTESIAN_POINT('Ctrl Pts',(110.310890750078,13.8320601883633,31.));
#97595=CARTESIAN_POINT('Ctrl Pts',(110.310890750078,13.8320601883633,26.));
#97596=CARTESIAN_POINT('Ctrl Pts',(110.299223524167,13.8033193370998,31.));
#97597=CARTESIAN_POINT('Ctrl Pts',(110.299223524167,13.8033193370998,26.));
#97598=CARTESIAN_POINT('Ctrl Pts',(110.286866168639,13.7742798843164,31.));
#97599=CARTESIAN_POINT('Ctrl Pts',(110.286866168639,13.7742798843164,26.));
#97600=CARTESIAN_POINT('Ctrl Pts',(110.273813320286,13.7449699394693,31.));
#97601=CARTESIAN_POINT('Ctrl Pts',(110.273813320286,13.7449699394693,26.));
#97602=CARTESIAN_POINT('Ctrl Pts',(110.260059639053,13.7154103674415,31.));
#97603=CARTESIAN_POINT('Ctrl Pts',(110.260059639053,13.7154103674415,26.));
#97604=CARTESIAN_POINT('Ctrl Pts',(110.245600642905,13.6856159512311,31.));
#97605=CARTESIAN_POINT('Ctrl Pts',(110.245600642905,13.6856159512311,26.));
#97606=CARTESIAN_POINT('Ctrl Pts',(110.230433584305,13.6555970993781,31.));
#97607=CARTESIAN_POINT('Ctrl Pts',(110.230433584305,13.6555970993781,26.));
#97608=CARTESIAN_POINT('Ctrl Pts',(110.214558692533,13.6253614515313,31.));
#97609=CARTESIAN_POINT('Ctrl Pts',(110.214558692533,13.6253614515313,26.));
#97610=CARTESIAN_POINT('Ctrl Pts',(110.197979759147,13.5949151914461,31.));
#97611=CARTESIAN_POINT('Ctrl Pts',(110.197979759147,13.5949151914461,26.));
#97612=CARTESIAN_POINT('Ctrl Pts',(110.180702188106,13.564262914511,31.));
#97613=CARTESIAN_POINT('Ctrl Pts',(110.180702188106,13.564262914511,26.));
#97614=CARTESIAN_POINT('Ctrl Pts',(110.166325720903,13.5395788027193,31.));
#97615=CARTESIAN_POINT('Ctrl Pts',(110.166325720903,13.5395788027193,26.));
#97616=CARTESIAN_POINT('Ctrl Pts',(110.155233489078,13.5209752322933,31.));
#97617=CARTESIAN_POINT('Ctrl Pts',(110.155233489078,13.5209752322933,26.));
#97618=CARTESIAN_POINT('Ctrl Pts',(110.147701192417,13.5085327087831,31.));
#97619=CARTESIAN_POINT('Ctrl Pts',(110.147701192417,13.5085327087831,26.));
#97620=CARTESIAN_POINT('Ctrl Pts',(110.143900675185,13.5023014112014,31.));
#97621=CARTESIAN_POINT('Ctrl Pts',(110.143900675185,13.5023014112014,26.));
#97622=CARTESIAN_POINT('',(110.40545429899,14.2631614489809,31.));
#97623=CARTESIAN_POINT('Ctrl Pts',(110.40545429899,14.2631614489809,31.));
#97624=CARTESIAN_POINT('Ctrl Pts',(110.405664390452,14.2608157673365,31.));
#97625=CARTESIAN_POINT('Ctrl Pts',(110.406024771178,14.2559601069417,31.));
#97626=CARTESIAN_POINT('Ctrl Pts',(110.406385935683,14.2481837198662,31.));
#97627=CARTESIAN_POINT('Ctrl Pts',(110.406508025415,14.2368276704446,31.));
#97628=CARTESIAN_POINT('Ctrl Pts',(110.406057128268,14.2209886536872,31.));
#97629=CARTESIAN_POINT('Ctrl Pts',(110.404996096367,14.2035304982819,31.));
#97630=CARTESIAN_POINT('Ctrl Pts',(110.40331669726,14.184515373837,31.));
#97631=CARTESIAN_POINT('Ctrl Pts',(110.401009852508,14.1640634597682,31.));
#97632=CARTESIAN_POINT('Ctrl Pts',(110.398066294489,14.1423563916581,31.));
#97633=CARTESIAN_POINT('Ctrl Pts',(110.3944768539,14.1196033405171,31.));
#97634=CARTESIAN_POINT('Ctrl Pts',(110.390232980035,14.0960139440535,31.));
#97635=CARTESIAN_POINT('Ctrl Pts',(110.385327228041,14.0717714163371,31.));
#97636=CARTESIAN_POINT('Ctrl Pts',(110.379754111412,14.0469993250182,31.));
#97637=CARTESIAN_POINT('Ctrl Pts',(110.373510209703,14.0217543266667,31.));
#97638=CARTESIAN_POINT('Ctrl Pts',(110.366593344528,13.9960512119543,31.));
#97639=CARTESIAN_POINT('Ctrl Pts',(110.359002138437,13.9698801062394,31.));
#97640=CARTESIAN_POINT('Ctrl Pts',(110.350735557909,13.943225285516,31.));
#97641=CARTESIAN_POINT('Ctrl Pts',(110.34179264797,13.9160868433413,31.));
#97642=CARTESIAN_POINT('Ctrl Pts',(110.332172212069,13.8884878805099,31.));
#97643=CARTESIAN_POINT('Ctrl Pts',(110.321872455148,13.8604644706007,31.));
#97644=CARTESIAN_POINT('Ctrl Pts',(110.310890750078,13.8320601883633,31.));
#97645=CARTESIAN_POINT('Ctrl Pts',(110.299223524167,13.8033193370998,31.));
#97646=CARTESIAN_POINT('Ctrl Pts',(110.286866168639,13.7742798843164,31.));
#97647=CARTESIAN_POINT('Ctrl Pts',(110.273813320286,13.7449699394693,31.));
#97648=CARTESIAN_POINT('Ctrl Pts',(110.260059639053,13.7154103674415,31.));
#97649=CARTESIAN_POINT('Ctrl Pts',(110.245600642905,13.6856159512311,31.));
#97650=CARTESIAN_POINT('Ctrl Pts',(110.230433584305,13.6555970993781,31.));
#97651=CARTESIAN_POINT('Ctrl Pts',(110.214558692533,13.6253614515313,31.));
#97652=CARTESIAN_POINT('Ctrl Pts',(110.197979759147,13.5949151914461,31.));
#97653=CARTESIAN_POINT('Ctrl Pts',(110.180702188106,13.564262914511,31.));
#97654=CARTESIAN_POINT('Ctrl Pts',(110.166325720903,13.5395788027193,31.));
#97655=CARTESIAN_POINT('Ctrl Pts',(110.155233489078,13.5209752322933,31.));
#97656=CARTESIAN_POINT('Ctrl Pts',(110.147701192417,13.5085327087831,31.));
#97657=CARTESIAN_POINT('Ctrl Pts',(110.143900675185,13.5023014112014,31.));
#97658=CARTESIAN_POINT('',(110.40545429899,14.2631614489809,26.));
#97659=CARTESIAN_POINT('Ctrl Pts',(110.40545429899,14.2631614489809,26.));
#97660=CARTESIAN_POINT('Ctrl Pts',(110.405664390452,14.2608157673365,26.));
#97661=CARTESIAN_POINT('Ctrl Pts',(110.406024771178,14.2559601069417,26.));
#97662=CARTESIAN_POINT('Ctrl Pts',(110.406385935683,14.2481837198662,26.));
#97663=CARTESIAN_POINT('Ctrl Pts',(110.406508025415,14.2368276704446,26.));
#97664=CARTESIAN_POINT('Ctrl Pts',(110.406057128268,14.2209886536872,26.));
#97665=CARTESIAN_POINT('Ctrl Pts',(110.404996096367,14.2035304982819,26.));
#97666=CARTESIAN_POINT('Ctrl Pts',(110.40331669726,14.184515373837,26.));
#97667=CARTESIAN_POINT('Ctrl Pts',(110.401009852508,14.1640634597682,26.));
#97668=CARTESIAN_POINT('Ctrl Pts',(110.398066294489,14.1423563916581,26.));
#97669=CARTESIAN_POINT('Ctrl Pts',(110.3944768539,14.1196033405171,26.));
#97670=CARTESIAN_POINT('Ctrl Pts',(110.390232980035,14.0960139440535,26.));
#97671=CARTESIAN_POINT('Ctrl Pts',(110.385327228041,14.0717714163371,26.));
#97672=CARTESIAN_POINT('Ctrl Pts',(110.379754111412,14.0469993250182,26.));
#97673=CARTESIAN_POINT('Ctrl Pts',(110.373510209703,14.0217543266667,26.));
#97674=CARTESIAN_POINT('Ctrl Pts',(110.366593344528,13.9960512119543,26.));
#97675=CARTESIAN_POINT('Ctrl Pts',(110.359002138437,13.9698801062394,26.));
#97676=CARTESIAN_POINT('Ctrl Pts',(110.350735557909,13.943225285516,26.));
#97677=CARTESIAN_POINT('Ctrl Pts',(110.34179264797,13.9160868433413,26.));
#97678=CARTESIAN_POINT('Ctrl Pts',(110.332172212069,13.8884878805099,26.));
#97679=CARTESIAN_POINT('Ctrl Pts',(110.321872455148,13.8604644706007,26.));
#97680=CARTESIAN_POINT('Ctrl Pts',(110.310890750078,13.8320601883633,26.));
#97681=CARTESIAN_POINT('Ctrl Pts',(110.299223524167,13.8033193370998,26.));
#97682=CARTESIAN_POINT('Ctrl Pts',(110.286866168639,13.7742798843164,26.));
#97683=CARTESIAN_POINT('Ctrl Pts',(110.273813320286,13.7449699394693,26.));
#97684=CARTESIAN_POINT('Ctrl Pts',(110.260059639053,13.7154103674415,26.));
#97685=CARTESIAN_POINT('Ctrl Pts',(110.245600642905,13.6856159512311,26.));
#97686=CARTESIAN_POINT('Ctrl Pts',(110.230433584305,13.6555970993781,26.));
#97687=CARTESIAN_POINT('Ctrl Pts',(110.214558692533,13.6253614515313,26.));
#97688=CARTESIAN_POINT('Ctrl Pts',(110.197979759147,13.5949151914461,26.));
#97689=CARTESIAN_POINT('Ctrl Pts',(110.180702188106,13.564262914511,26.));
#97690=CARTESIAN_POINT('Ctrl Pts',(110.166325720903,13.5395788027193,26.));
#97691=CARTESIAN_POINT('Ctrl Pts',(110.155233489078,13.5209752322933,26.));
#97692=CARTESIAN_POINT('Ctrl Pts',(110.147701192417,13.5085327087831,26.));
#97693=CARTESIAN_POINT('Ctrl Pts',(110.143900675185,13.5023014112014,26.));
#97694=CARTESIAN_POINT('',(110.40545429899,14.2631614489809,31.));
#97695=CARTESIAN_POINT('Origin',(110.347877083772,14.7938174514562,31.));
#97696=CARTESIAN_POINT('',(110.40545429899,14.2631614489809,31.));
#97697=CARTESIAN_POINT('',(110.40545429899,14.2631614489809,26.));
#97698=CARTESIAN_POINT('Origin',(110.000000000016,14.1469087257281,31.));
#97699=CARTESIAN_POINT('Origin',(110.,18.,30.4));
#97700=CARTESIAN_POINT('',(107.5,18.,34.8));
#97701=CARTESIAN_POINT('Origin',(110.,18.,34.8));
#97702=CARTESIAN_POINT('',(107.5,18.,26.));
#97703=CARTESIAN_POINT('',(107.5,18.,30.4));
#97704=CARTESIAN_POINT('Origin',(110.,18.,26.));
#97705=CARTESIAN_POINT('Origin',(113.375,18.,26.));
#97706=CARTESIAN_POINT('Origin',(114.5,18.,31.8));
#97707=CARTESIAN_POINT('',(105.5,18.,31.8));
#97708=CARTESIAN_POINT('Origin',(110.,18.,31.8));
#97709=CARTESIAN_POINT('Origin',(110.,18.,33.15));
#97710=CARTESIAN_POINT('',(105.5,18.,34.5));
#97711=CARTESIAN_POINT('Origin',(110.,18.,34.5));
#97712=CARTESIAN_POINT('',(105.5,18.,33.15));
#97713=CARTESIAN_POINT('Origin',(110.,18.,34.65));
#97714=CARTESIAN_POINT('',(105.8,18.,34.8));
#97715=CARTESIAN_POINT('Origin',(110.,18.,34.8));
#97716=CARTESIAN_POINT('',(105.65,18.,34.65));
#97717=CARTESIAN_POINT('Origin',(112.5,18.,34.8));
#113950=UNCERTAINTY_MEASURE_WITH_UNIT(LENGTH_MEASURE(0.01),#113985,
'DISTANCE_ACCURACY_VALUE',
'Maximum model space distance between geometric entities at asserted c
onnectivities');
#113964=UNCERTAINTY_MEASURE_WITH_UNIT(LENGTH_MEASURE(0.01),#113985,
'DISTANCE_ACCURACY_VALUE',
'Maximum model space distance between geometric entities at asserted c
onnectivities');
#113970=(
GEOMETRIC_REPRESENTATION_CONTEXT(3)
GLOBAL_UNCERTAINTY_ASSIGNED_CONTEXT((#113950))
GLOBAL_UNIT_ASSIGNED_CONTEXT((#113985,#113987,#113988))
REPRESENTATION_CONTEXT('','3D')
);
#113984=(
GEOMETRIC_REPRESENTATION_CONTEXT(3)
GLOBAL_UNCERTAINTY_ASSIGNED_CONTEXT((#113964))
GLOBAL_UNIT_ASSIGNED_CONTEXT((#113985,#113987,#113988))
REPRESENTATION_CONTEXT('','3D')
);
#113985=(
LENGTH_UNIT()
NAMED_UNIT(*)
SI_UNIT(.MILLI.,.METRE.)
);
#113987=(
NAMED_UNIT(*)
PLANE_ANGLE_UNIT()
SI_UNIT($,.RADIAN.)
);
#113988=(
NAMED_UNIT(*)
SI_UNIT($,.STERADIAN.)
SOLID_ANGLE_UNIT()
);
#113994=SHAPE_DEFINITION_REPRESENTATION(#114013,#114056);
#114013=PRODUCT_DEFINITION_SHAPE('',$,#114076);
#114056=SHAPE_REPRESENTATION('',(#61989),#113970);
#114070=PRODUCT_DEFINITION_CONTEXT('part definition',#114129,'design');
#114076=PRODUCT_DEFINITION('2026-10-05-09-49-09-808',
'Spur Pinion m0.5 z16 with Hub',#114095,#114070);
#114095=PRODUCT_DEFINITION_FORMATION('',$,#114136);
#114129=APPLICATION_CONTEXT(
'Core Data for Automotive Mechanical Design Process');
#114130=PRODUCT_CONTEXT('part definition',#114129,'mechanical');
#114136=PRODUCT('2026-10-05-09-49-09-808',
'Spur Pinion m0.5 z16 with Hub',$,(#114130));
#114297=COLOUR_RGB('Sky Blue',0.24,0.69,0.87);
#114298=FILL_AREA_STYLE_COLOUR('',#114297);
#114299=FILL_AREA_STYLE('',(#114298));
#114300=SURFACE_STYLE_FILL_AREA(#114299);
#114301=SURFACE_SIDE_STYLE('',(#114300));
#114302=SURFACE_STYLE_USAGE(.BOTH.,#114301);
#114303=PRESENTATION_STYLE_ASSIGNMENT((#114302));
ENDSEC;
END-ISO-10303-21;
